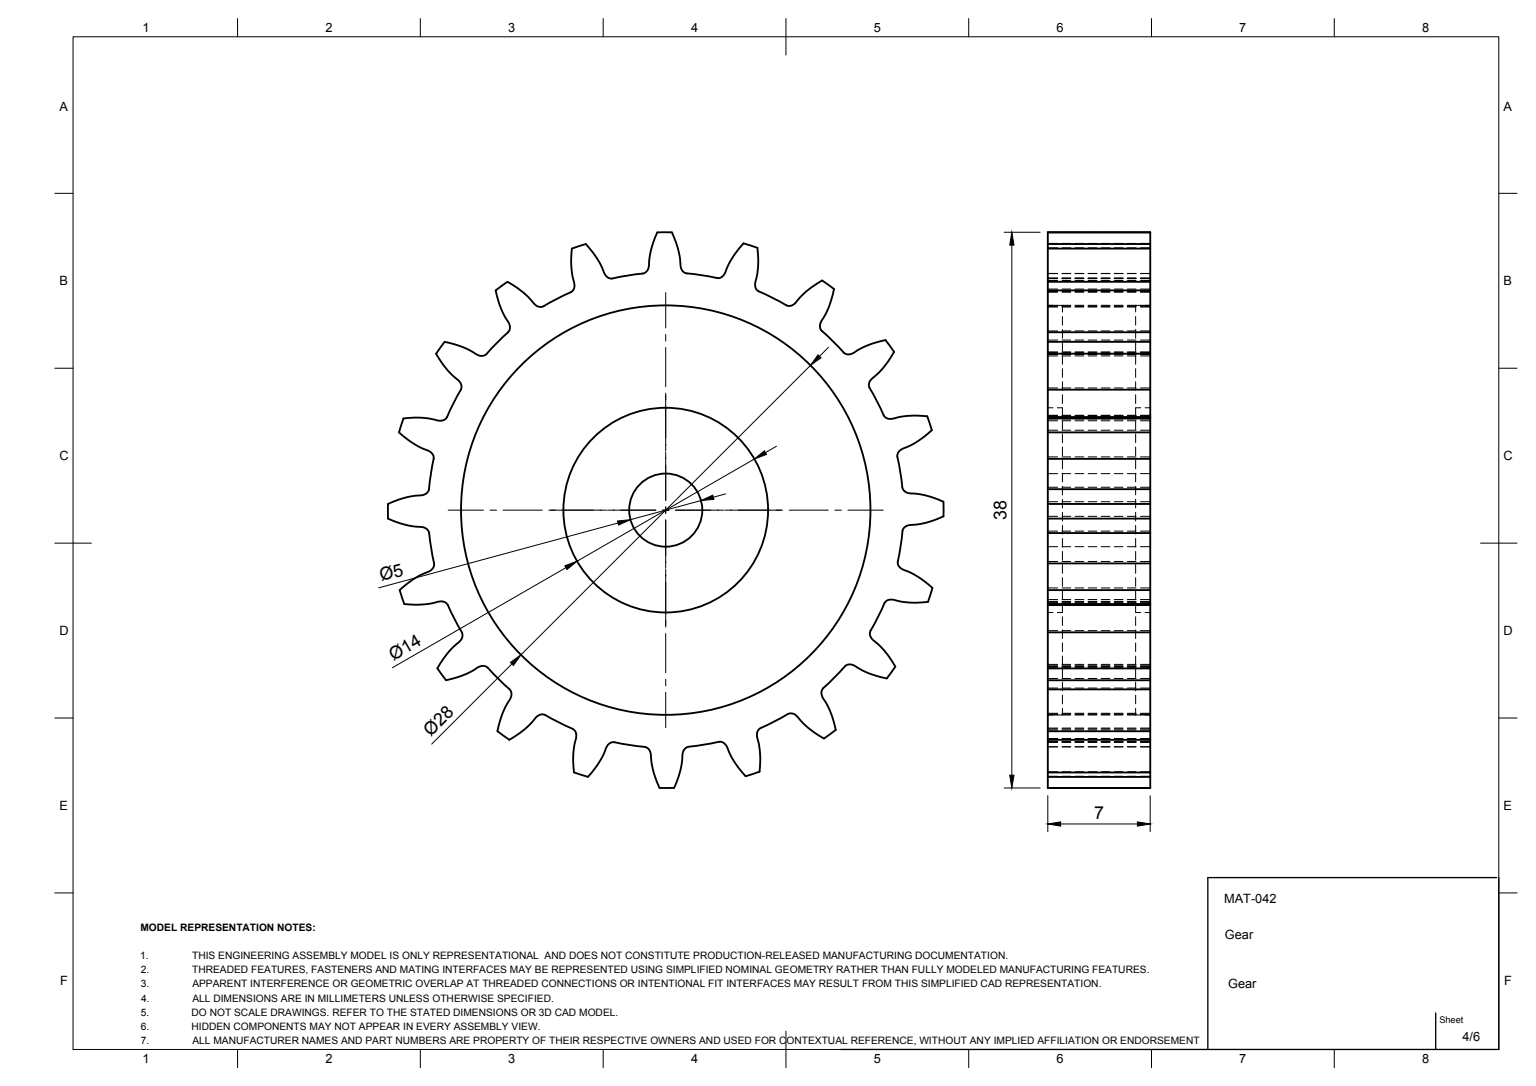
ISO-10303-21;
HEADER;
/* Generated by software containing ST-Developer
 * from STEP Tools, Inc. (www.steptools.com) 
 */

FILE_DESCRIPTION(
/* description */ ('STEP AP214'),
/* implementation_level */ '2;1');

FILE_NAME(
/* name */ 'Gear.step',
/* time_stamp */ '2026-11-14T22:03:06-08:00',
/* author */ (''),
/* organization */ (''),
/* preprocessor_version */ 'ST-DEVELOPER v20.2',
/* originating_system */ 'Autodesk Translation Framework v15.17.0.0',
/* authorisation */ '');

FILE_SCHEMA (('AUTOMOTIVE_DESIGN { 1 0 10303 214 3 1 1 }'));
ENDSEC;

DATA;
#10=MECHANICAL_DESIGN_GEOMETRIC_PRESENTATION_REPRESENTATION('',(#309),#12966);
#167=B_SPLINE_SURFACE_WITH_KNOTS('',3,1,((#10554,#10555),(#10556,#10557),
(#10558,#10559),(#10560,#10561),(#10562,#10563),(#10564,#10565),(#10566,
#10567),(#10568,#10569),(#10570,#10571),(#10572,#10573),(#10574,#10575),
(#10576,#10577),(#10578,#10579),(#10580,#10581),(#10582,#10583),(#10584,
#10585),(#10586,#10587),(#10588,#10589),(#10590,#10591),(#10592,#10593),
(#10594,#10595),(#10596,#10597),(#10598,#10599)),.UNSPECIFIED.,.F.,.F.,
 .F.,(4,1,1,1,1,1,1,1,1,1,1,1,1,1,1,1,1,1,1,1,4),(2,2),(0.0323453817713401,
0.0983189520624214,0.14064060480402,0.176193019733645,0.208307484243854,
0.23948443235858,0.271287112904486,0.28220667781497,0.293329328714142,0.304676551002397,
0.319437818234531,0.350137192454192,0.38765864687273,0.432002181900136,
0.483167797782405,0.541155494678712,0.605965272697963,0.67759713191795,
0.75605107239617,0.841327094176323,1.),(0.,0.84),.UNSPECIFIED.);
#168=B_SPLINE_SURFACE_WITH_KNOTS('',3,1,((#10604,#10605),(#10606,#10607),
(#10608,#10609),(#10610,#10611),(#10612,#10613),(#10614,#10615),(#10616,
#10617),(#10618,#10619),(#10620,#10621),(#10622,#10623),(#10624,#10625),
(#10626,#10627),(#10628,#10629),(#10630,#10631),(#10632,#10633),(#10634,
#10635),(#10636,#10637),(#10638,#10639),(#10640,#10641),(#10642,#10643),
(#10644,#10645),(#10646,#10647),(#10648,#10649)),.UNSPECIFIED.,.F.,.F.,
 .F.,(4,1,1,1,1,1,1,1,1,1,1,1,1,1,1,1,1,1,1,1,4),(2,2),(0.,0.158672905823676,
0.243948927603829,0.322402868082049,0.394034727302036,0.458844505321287,
0.516832202217594,0.567997818099863,0.612341353127269,0.649862807545807,
0.680562181765468,0.695323448997602,0.706670671285856,0.717793322185029,
0.728712887095513,0.760515567641419,0.791692515756145,0.823806980266354,
0.859359395195979,0.901681047937578,0.967654618228659),(0.,0.839999999999999),
 .UNSPECIFIED.);
#169=B_SPLINE_SURFACE_WITH_KNOTS('',3,1,((#10653,#10654),(#10655,#10656),
(#10657,#10658),(#10659,#10660),(#10661,#10662),(#10663,#10664),(#10665,
#10666),(#10667,#10668),(#10669,#10670),(#10671,#10672),(#10673,#10674),
(#10675,#10676),(#10677,#10678),(#10679,#10680),(#10681,#10682),(#10683,
#10684),(#10685,#10686),(#10687,#10688),(#10689,#10690),(#10691,#10692),
(#10693,#10694),(#10695,#10696),(#10697,#10698)),.UNSPECIFIED.,.F.,.F.,
 .F.,(4,1,1,1,1,1,1,1,1,1,1,1,1,1,1,1,1,1,1,1,4),(2,2),(0.0323453817713401,
0.0983189520624214,0.14064060480402,0.176193019733645,0.208307484243854,
0.23948443235858,0.271287112904486,0.28220667781497,0.293329328714142,0.304676551002397,
0.319437818234531,0.350137192454192,0.38765864687273,0.432002181900136,
0.483167797782405,0.541155494678712,0.605965272697963,0.67759713191795,
0.75605107239617,0.841327094176323,1.),(0.,0.84),.UNSPECIFIED.);
#170=B_SPLINE_SURFACE_WITH_KNOTS('',3,1,((#10702,#10703),(#10704,#10705),
(#10706,#10707),(#10708,#10709),(#10710,#10711),(#10712,#10713),(#10714,
#10715),(#10716,#10717),(#10718,#10719),(#10720,#10721),(#10722,#10723),
(#10724,#10725),(#10726,#10727),(#10728,#10729),(#10730,#10731),(#10732,
#10733),(#10734,#10735),(#10736,#10737),(#10738,#10739),(#10740,#10741),
(#10742,#10743),(#10744,#10745),(#10746,#10747)),.UNSPECIFIED.,.F.,.F.,
 .F.,(4,1,1,1,1,1,1,1,1,1,1,1,1,1,1,1,1,1,1,1,4),(2,2),(0.,0.158672905823676,
0.243948927603829,0.322402868082049,0.394034727302036,0.458844505321287,
0.516832202217594,0.567997818099863,0.612341353127269,0.649862807545807,
0.680562181765468,0.695323448997602,0.706670671285856,0.717793322185029,
0.728712887095513,0.760515567641419,0.791692515756145,0.823806980266354,
0.859359395195979,0.901681047937578,0.967654618228659),(0.,0.839999999999998),
 .UNSPECIFIED.);
#171=B_SPLINE_SURFACE_WITH_KNOTS('',3,1,((#10751,#10752),(#10753,#10754),
(#10755,#10756),(#10757,#10758),(#10759,#10760),(#10761,#10762),(#10763,
#10764),(#10765,#10766),(#10767,#10768),(#10769,#10770),(#10771,#10772),
(#10773,#10774),(#10775,#10776),(#10777,#10778),(#10779,#10780),(#10781,
#10782),(#10783,#10784),(#10785,#10786),(#10787,#10788),(#10789,#10790),
(#10791,#10792),(#10793,#10794),(#10795,#10796)),.UNSPECIFIED.,.F.,.F.,
 .F.,(4,1,1,1,1,1,1,1,1,1,1,1,1,1,1,1,1,1,1,1,4),(2,2),(0.0323453817713401,
0.0983189520624214,0.14064060480402,0.176193019733645,0.208307484243854,
0.23948443235858,0.271287112904486,0.28220667781497,0.293329328714142,0.304676551002397,
0.319437818234531,0.350137192454192,0.38765864687273,0.432002181900136,
0.483167797782405,0.541155494678712,0.605965272697963,0.67759713191795,
0.75605107239617,0.841327094176323,1.),(0.,0.84),.UNSPECIFIED.);
#172=B_SPLINE_SURFACE_WITH_KNOTS('',3,1,((#10800,#10801),(#10802,#10803),
(#10804,#10805),(#10806,#10807),(#10808,#10809),(#10810,#10811),(#10812,
#10813),(#10814,#10815),(#10816,#10817),(#10818,#10819),(#10820,#10821),
(#10822,#10823),(#10824,#10825),(#10826,#10827),(#10828,#10829),(#10830,
#10831),(#10832,#10833),(#10834,#10835),(#10836,#10837),(#10838,#10839),
(#10840,#10841),(#10842,#10843),(#10844,#10845)),.UNSPECIFIED.,.F.,.F.,
 .F.,(4,1,1,1,1,1,1,1,1,1,1,1,1,1,1,1,1,1,1,1,4),(2,2),(0.,0.158672905823676,
0.243948927603829,0.322402868082049,0.394034727302036,0.458844505321287,
0.516832202217594,0.567997818099863,0.612341353127269,0.649862807545807,
0.680562181765468,0.695323448997602,0.706670671285856,0.717793322185029,
0.728712887095513,0.760515567641419,0.791692515756145,0.823806980266354,
0.859359395195979,0.901681047937578,0.967654618228659),(0.,0.839999999999999),
 .UNSPECIFIED.);
#173=B_SPLINE_SURFACE_WITH_KNOTS('',3,1,((#10849,#10850),(#10851,#10852),
(#10853,#10854),(#10855,#10856),(#10857,#10858),(#10859,#10860),(#10861,
#10862),(#10863,#10864),(#10865,#10866),(#10867,#10868),(#10869,#10870),
(#10871,#10872),(#10873,#10874),(#10875,#10876),(#10877,#10878),(#10879,
#10880),(#10881,#10882),(#10883,#10884),(#10885,#10886),(#10887,#10888),
(#10889,#10890),(#10891,#10892),(#10893,#10894)),.UNSPECIFIED.,.F.,.F.,
 .F.,(4,1,1,1,1,1,1,1,1,1,1,1,1,1,1,1,1,1,1,1,4),(2,2),(0.0323453817713401,
0.0983189520624214,0.14064060480402,0.176193019733645,0.208307484243854,
0.23948443235858,0.271287112904486,0.28220667781497,0.293329328714142,0.304676551002397,
0.319437818234531,0.350137192454192,0.38765864687273,0.432002181900136,
0.483167797782405,0.541155494678712,0.605965272697963,0.67759713191795,
0.75605107239617,0.841327094176323,1.),(0.,0.840000000000002),
 .UNSPECIFIED.);
#174=B_SPLINE_SURFACE_WITH_KNOTS('',3,1,((#10898,#10899),(#10900,#10901),
(#10902,#10903),(#10904,#10905),(#10906,#10907),(#10908,#10909),(#10910,
#10911),(#10912,#10913),(#10914,#10915),(#10916,#10917),(#10918,#10919),
(#10920,#10921),(#10922,#10923),(#10924,#10925),(#10926,#10927),(#10928,
#10929),(#10930,#10931),(#10932,#10933),(#10934,#10935),(#10936,#10937),
(#10938,#10939),(#10940,#10941),(#10942,#10943)),.UNSPECIFIED.,.F.,.F.,
 .F.,(4,1,1,1,1,1,1,1,1,1,1,1,1,1,1,1,1,1,1,1,4),(2,2),(0.,0.158672905823676,
0.243948927603829,0.322402868082049,0.394034727302036,0.458844505321287,
0.516832202217594,0.567997818099863,0.612341353127269,0.649862807545807,
0.680562181765468,0.695323448997602,0.706670671285856,0.717793322185029,
0.728712887095513,0.760515567641419,0.791692515756145,0.823806980266354,
0.859359395195979,0.901681047937578,0.967654618228659),(0.,0.84),
 .UNSPECIFIED.);
#175=B_SPLINE_SURFACE_WITH_KNOTS('',3,1,((#10947,#10948),(#10949,#10950),
(#10951,#10952),(#10953,#10954),(#10955,#10956),(#10957,#10958),(#10959,
#10960),(#10961,#10962),(#10963,#10964),(#10965,#10966),(#10967,#10968),
(#10969,#10970),(#10971,#10972),(#10973,#10974),(#10975,#10976),(#10977,
#10978),(#10979,#10980),(#10981,#10982),(#10983,#10984),(#10985,#10986),
(#10987,#10988),(#10989,#10990),(#10991,#10992)),.UNSPECIFIED.,.F.,.F.,
 .F.,(4,1,1,1,1,1,1,1,1,1,1,1,1,1,1,1,1,1,1,1,4),(2,2),(0.0323453817713401,
0.0983189520624214,0.14064060480402,0.176193019733645,0.208307484243854,
0.23948443235858,0.271287112904486,0.28220667781497,0.293329328714142,0.304676551002397,
0.319437818234531,0.350137192454192,0.38765864687273,0.432002181900136,
0.483167797782405,0.541155494678712,0.605965272697963,0.67759713191795,
0.75605107239617,0.841327094176323,1.),(0.,0.84),.UNSPECIFIED.);
#176=B_SPLINE_SURFACE_WITH_KNOTS('',3,1,((#10996,#10997),(#10998,#10999),
(#11000,#11001),(#11002,#11003),(#11004,#11005),(#11006,#11007),(#11008,
#11009),(#11010,#11011),(#11012,#11013),(#11014,#11015),(#11016,#11017),
(#11018,#11019),(#11020,#11021),(#11022,#11023),(#11024,#11025),(#11026,
#11027),(#11028,#11029),(#11030,#11031),(#11032,#11033),(#11034,#11035),
(#11036,#11037),(#11038,#11039),(#11040,#11041)),.UNSPECIFIED.,.F.,.F.,
 .F.,(4,1,1,1,1,1,1,1,1,1,1,1,1,1,1,1,1,1,1,1,4),(2,2),(0.,0.158672905823676,
0.243948927603829,0.322402868082049,0.394034727302036,0.458844505321287,
0.516832202217594,0.567997818099863,0.612341353127269,0.649862807545807,
0.680562181765468,0.695323448997602,0.706670671285856,0.717793322185029,
0.728712887095513,0.760515567641419,0.791692515756145,0.823806980266354,
0.859359395195979,0.901681047937578,0.967654618228659),(0.,0.839999999999999),
 .UNSPECIFIED.);
#177=B_SPLINE_SURFACE_WITH_KNOTS('',3,1,((#11045,#11046),(#11047,#11048),
(#11049,#11050),(#11051,#11052),(#11053,#11054),(#11055,#11056),(#11057,
#11058),(#11059,#11060),(#11061,#11062),(#11063,#11064),(#11065,#11066),
(#11067,#11068),(#11069,#11070),(#11071,#11072),(#11073,#11074),(#11075,
#11076),(#11077,#11078),(#11079,#11080),(#11081,#11082),(#11083,#11084),
(#11085,#11086),(#11087,#11088),(#11089,#11090)),.UNSPECIFIED.,.F.,.F.,
 .F.,(4,1,1,1,1,1,1,1,1,1,1,1,1,1,1,1,1,1,1,1,4),(2,2),(0.0323453817713401,
0.0983189520624214,0.14064060480402,0.176193019733645,0.208307484243854,
0.23948443235858,0.271287112904486,0.28220667781497,0.293329328714142,0.304676551002397,
0.319437818234531,0.350137192454192,0.38765864687273,0.432002181900136,
0.483167797782405,0.541155494678712,0.605965272697963,0.67759713191795,
0.75605107239617,0.841327094176323,1.),(0.,0.84),.UNSPECIFIED.);
#178=B_SPLINE_SURFACE_WITH_KNOTS('',3,1,((#11094,#11095),(#11096,#11097),
(#11098,#11099),(#11100,#11101),(#11102,#11103),(#11104,#11105),(#11106,
#11107),(#11108,#11109),(#11110,#11111),(#11112,#11113),(#11114,#11115),
(#11116,#11117),(#11118,#11119),(#11120,#11121),(#11122,#11123),(#11124,
#11125),(#11126,#11127),(#11128,#11129),(#11130,#11131),(#11132,#11133),
(#11134,#11135),(#11136,#11137),(#11138,#11139)),.UNSPECIFIED.,.F.,.F.,
 .F.,(4,1,1,1,1,1,1,1,1,1,1,1,1,1,1,1,1,1,1,1,4),(2,2),(0.,0.158672905823676,
0.243948927603829,0.322402868082049,0.394034727302036,0.458844505321287,
0.516832202217594,0.567997818099863,0.612341353127269,0.649862807545807,
0.680562181765468,0.695323448997602,0.706670671285856,0.717793322185029,
0.728712887095513,0.760515567641419,0.791692515756145,0.823806980266354,
0.859359395195979,0.901681047937578,0.967654618228659),(0.,0.84),
 .UNSPECIFIED.);
#179=B_SPLINE_SURFACE_WITH_KNOTS('',3,1,((#11143,#11144),(#11145,#11146),
(#11147,#11148),(#11149,#11150),(#11151,#11152),(#11153,#11154),(#11155,
#11156),(#11157,#11158),(#11159,#11160),(#11161,#11162),(#11163,#11164),
(#11165,#11166),(#11167,#11168),(#11169,#11170),(#11171,#11172),(#11173,
#11174),(#11175,#11176),(#11177,#11178),(#11179,#11180),(#11181,#11182),
(#11183,#11184),(#11185,#11186),(#11187,#11188)),.UNSPECIFIED.,.F.,.F.,
 .F.,(4,1,1,1,1,1,1,1,1,1,1,1,1,1,1,1,1,1,1,1,4),(2,2),(0.0323453817713401,
0.0983189520624214,0.14064060480402,0.176193019733645,0.208307484243854,
0.23948443235858,0.271287112904486,0.28220667781497,0.293329328714142,0.304676551002397,
0.319437818234531,0.350137192454192,0.38765864687273,0.432002181900136,
0.483167797782405,0.541155494678712,0.605965272697963,0.67759713191795,
0.75605107239617,0.841327094176323,1.),(0.,0.84),.UNSPECIFIED.);
#180=B_SPLINE_SURFACE_WITH_KNOTS('',3,1,((#11192,#11193),(#11194,#11195),
(#11196,#11197),(#11198,#11199),(#11200,#11201),(#11202,#11203),(#11204,
#11205),(#11206,#11207),(#11208,#11209),(#11210,#11211),(#11212,#11213),
(#11214,#11215),(#11216,#11217),(#11218,#11219),(#11220,#11221),(#11222,
#11223),(#11224,#11225),(#11226,#11227),(#11228,#11229),(#11230,#11231),
(#11232,#11233),(#11234,#11235),(#11236,#11237)),.UNSPECIFIED.,.F.,.F.,
 .F.,(4,1,1,1,1,1,1,1,1,1,1,1,1,1,1,1,1,1,1,1,4),(2,2),(0.,0.158672905823676,
0.243948927603829,0.322402868082049,0.394034727302036,0.458844505321287,
0.516832202217594,0.567997818099863,0.612341353127269,0.649862807545807,
0.680562181765468,0.695323448997602,0.706670671285856,0.717793322185029,
0.728712887095513,0.760515567641419,0.791692515756145,0.823806980266354,
0.859359395195979,0.901681047937578,0.967654618228659),(0.,0.84),
 .UNSPECIFIED.);
#181=B_SPLINE_SURFACE_WITH_KNOTS('',3,1,((#11241,#11242),(#11243,#11244),
(#11245,#11246),(#11247,#11248),(#11249,#11250),(#11251,#11252),(#11253,
#11254),(#11255,#11256),(#11257,#11258),(#11259,#11260),(#11261,#11262),
(#11263,#11264),(#11265,#11266),(#11267,#11268),(#11269,#11270),(#11271,
#11272),(#11273,#11274),(#11275,#11276),(#11277,#11278),(#11279,#11280),
(#11281,#11282),(#11283,#11284),(#11285,#11286)),.UNSPECIFIED.,.F.,.F.,
 .F.,(4,1,1,1,1,1,1,1,1,1,1,1,1,1,1,1,1,1,1,1,4),(2,2),(0.0323453817713401,
0.0983189520624214,0.14064060480402,0.176193019733645,0.208307484243854,
0.23948443235858,0.271287112904486,0.28220667781497,0.293329328714142,0.304676551002397,
0.319437818234531,0.350137192454192,0.38765864687273,0.432002181900136,
0.483167797782405,0.541155494678712,0.605965272697963,0.67759713191795,
0.75605107239617,0.841327094176323,1.),(0.,0.84),.UNSPECIFIED.);
#182=B_SPLINE_SURFACE_WITH_KNOTS('',3,1,((#11290,#11291),(#11292,#11293),
(#11294,#11295),(#11296,#11297),(#11298,#11299),(#11300,#11301),(#11302,
#11303),(#11304,#11305),(#11306,#11307),(#11308,#11309),(#11310,#11311),
(#11312,#11313),(#11314,#11315),(#11316,#11317),(#11318,#11319),(#11320,
#11321),(#11322,#11323),(#11324,#11325),(#11326,#11327),(#11328,#11329),
(#11330,#11331),(#11332,#11333),(#11334,#11335)),.UNSPECIFIED.,.F.,.F.,
 .F.,(4,1,1,1,1,1,1,1,1,1,1,1,1,1,1,1,1,1,1,1,4),(2,2),(0.,0.158672905823676,
0.243948927603829,0.322402868082049,0.394034727302036,0.458844505321287,
0.516832202217594,0.567997818099863,0.612341353127269,0.649862807545807,
0.680562181765468,0.695323448997602,0.706670671285856,0.717793322185029,
0.728712887095513,0.760515567641419,0.791692515756145,0.823806980266354,
0.859359395195979,0.901681047937578,0.967654618228659),(0.,0.839999999999999),
 .UNSPECIFIED.);
#183=B_SPLINE_SURFACE_WITH_KNOTS('',3,1,((#11339,#11340),(#11341,#11342),
(#11343,#11344),(#11345,#11346),(#11347,#11348),(#11349,#11350),(#11351,
#11352),(#11353,#11354),(#11355,#11356),(#11357,#11358),(#11359,#11360),
(#11361,#11362),(#11363,#11364),(#11365,#11366),(#11367,#11368),(#11369,
#11370),(#11371,#11372),(#11373,#11374),(#11375,#11376),(#11377,#11378),
(#11379,#11380),(#11381,#11382),(#11383,#11384)),.UNSPECIFIED.,.F.,.F.,
 .F.,(4,1,1,1,1,1,1,1,1,1,1,1,1,1,1,1,1,1,1,1,4),(2,2),(0.0323453817713401,
0.0983189520624214,0.14064060480402,0.176193019733645,0.208307484243854,
0.23948443235858,0.271287112904486,0.28220667781497,0.293329328714142,0.304676551002397,
0.319437818234531,0.350137192454192,0.38765864687273,0.432002181900136,
0.483167797782405,0.541155494678712,0.605965272697963,0.67759713191795,
0.75605107239617,0.841327094176323,1.),(0.,0.84),.UNSPECIFIED.);
#184=B_SPLINE_SURFACE_WITH_KNOTS('',3,1,((#11388,#11389),(#11390,#11391),
(#11392,#11393),(#11394,#11395),(#11396,#11397),(#11398,#11399),(#11400,
#11401),(#11402,#11403),(#11404,#11405),(#11406,#11407),(#11408,#11409),
(#11410,#11411),(#11412,#11413),(#11414,#11415),(#11416,#11417),(#11418,
#11419),(#11420,#11421),(#11422,#11423),(#11424,#11425),(#11426,#11427),
(#11428,#11429),(#11430,#11431),(#11432,#11433)),.UNSPECIFIED.,.F.,.F.,
 .F.,(4,1,1,1,1,1,1,1,1,1,1,1,1,1,1,1,1,1,1,1,4),(2,2),(0.,0.158672905823676,
0.243948927603829,0.322402868082049,0.394034727302036,0.458844505321287,
0.516832202217594,0.567997818099863,0.612341353127269,0.649862807545807,
0.680562181765468,0.695323448997602,0.706670671285856,0.717793322185029,
0.728712887095513,0.760515567641419,0.791692515756145,0.823806980266354,
0.859359395195979,0.901681047937578,0.967654618228659),(0.,0.839999999999999),
 .UNSPECIFIED.);
#185=B_SPLINE_SURFACE_WITH_KNOTS('',3,1,((#11434,#11435),(#11436,#11437),
(#11438,#11439),(#11440,#11441),(#11442,#11443),(#11444,#11445),(#11446,
#11447),(#11448,#11449),(#11450,#11451),(#11452,#11453),(#11454,#11455),
(#11456,#11457),(#11458,#11459),(#11460,#11461),(#11462,#11463),(#11464,
#11465),(#11466,#11467),(#11468,#11469),(#11470,#11471),(#11472,#11473),
(#11474,#11475),(#11476,#11477),(#11478,#11479)),.UNSPECIFIED.,.F.,.F.,
 .F.,(4,1,1,1,1,1,1,1,1,1,1,1,1,1,1,1,1,1,1,1,4),(2,2),(0.0323453817713401,
0.0983189520624214,0.14064060480402,0.176193019733645,0.208307484243854,
0.23948443235858,0.271287112904486,0.28220667781497,0.293329328714142,0.304676551002397,
0.319437818234531,0.350137192454192,0.38765864687273,0.432002181900136,
0.483167797782405,0.541155494678712,0.605965272697963,0.67759713191795,
0.75605107239617,0.841327094176323,1.),(0.,0.84),.UNSPECIFIED.);
#186=B_SPLINE_SURFACE_WITH_KNOTS('',3,1,((#11483,#11484),(#11485,#11486),
(#11487,#11488),(#11489,#11490),(#11491,#11492),(#11493,#11494),(#11495,
#11496),(#11497,#11498),(#11499,#11500),(#11501,#11502),(#11503,#11504),
(#11505,#11506),(#11507,#11508),(#11509,#11510),(#11511,#11512),(#11513,
#11514),(#11515,#11516),(#11517,#11518),(#11519,#11520),(#11521,#11522),
(#11523,#11524),(#11525,#11526),(#11527,#11528)),.UNSPECIFIED.,.F.,.F.,
 .F.,(4,1,1,1,1,1,1,1,1,1,1,1,1,1,1,1,1,1,1,1,4),(2,2),(0.,0.158672905823676,
0.243948927603829,0.322402868082049,0.394034727302036,0.458844505321287,
0.516832202217594,0.567997818099863,0.612341353127269,0.649862807545807,
0.680562181765468,0.695323448997602,0.706670671285856,0.717793322185029,
0.728712887095513,0.760515567641419,0.791692515756145,0.823806980266354,
0.859359395195979,0.901681047937578,0.967654618228659),(0.,0.839999999999999),
 .UNSPECIFIED.);
#187=B_SPLINE_SURFACE_WITH_KNOTS('',3,1,((#11532,#11533),(#11534,#11535),
(#11536,#11537),(#11538,#11539),(#11540,#11541),(#11542,#11543),(#11544,
#11545),(#11546,#11547),(#11548,#11549),(#11550,#11551),(#11552,#11553),
(#11554,#11555),(#11556,#11557),(#11558,#11559),(#11560,#11561),(#11562,
#11563),(#11564,#11565),(#11566,#11567),(#11568,#11569),(#11570,#11571),
(#11572,#11573),(#11574,#11575),(#11576,#11577)),.UNSPECIFIED.,.F.,.F.,
 .F.,(4,1,1,1,1,1,1,1,1,1,1,1,1,1,1,1,1,1,1,1,4),(2,2),(0.0323453817713401,
0.0983189520624214,0.14064060480402,0.176193019733645,0.208307484243854,
0.23948443235858,0.271287112904486,0.28220667781497,0.293329328714142,0.304676551002397,
0.319437818234531,0.350137192454192,0.38765864687273,0.432002181900136,
0.483167797782405,0.541155494678712,0.605965272697963,0.67759713191795,
0.75605107239617,0.841327094176323,1.),(0.,0.840000000000002),
 .UNSPECIFIED.);
#188=B_SPLINE_SURFACE_WITH_KNOTS('',3,1,((#11581,#11582),(#11583,#11584),
(#11585,#11586),(#11587,#11588),(#11589,#11590),(#11591,#11592),(#11593,
#11594),(#11595,#11596),(#11597,#11598),(#11599,#11600),(#11601,#11602),
(#11603,#11604),(#11605,#11606),(#11607,#11608),(#11609,#11610),(#11611,
#11612),(#11613,#11614),(#11615,#11616),(#11617,#11618),(#11619,#11620),
(#11621,#11622),(#11623,#11624),(#11625,#11626)),.UNSPECIFIED.,.F.,.F.,
 .F.,(4,1,1,1,1,1,1,1,1,1,1,1,1,1,1,1,1,1,1,1,4),(2,2),(0.,0.158672905823676,
0.243948927603829,0.322402868082049,0.394034727302036,0.458844505321287,
0.516832202217594,0.567997818099863,0.612341353127269,0.649862807545807,
0.680562181765468,0.695323448997602,0.706670671285856,0.717793322185029,
0.728712887095513,0.760515567641419,0.791692515756145,0.823806980266354,
0.859359395195979,0.901681047937578,0.967654618228659),(0.,0.84),
 .UNSPECIFIED.);
#189=B_SPLINE_SURFACE_WITH_KNOTS('',3,1,((#11630,#11631),(#11632,#11633),
(#11634,#11635),(#11636,#11637),(#11638,#11639),(#11640,#11641),(#11642,
#11643),(#11644,#11645),(#11646,#11647),(#11648,#11649),(#11650,#11651),
(#11652,#11653),(#11654,#11655),(#11656,#11657),(#11658,#11659),(#11660,
#11661),(#11662,#11663),(#11664,#11665),(#11666,#11667),(#11668,#11669),
(#11670,#11671),(#11672,#11673),(#11674,#11675)),.UNSPECIFIED.,.F.,.F.,
 .F.,(4,1,1,1,1,1,1,1,1,1,1,1,1,1,1,1,1,1,1,1,4),(2,2),(0.0323453817713401,
0.0983189520624214,0.14064060480402,0.176193019733645,0.208307484243854,
0.23948443235858,0.271287112904486,0.28220667781497,0.293329328714142,0.304676551002397,
0.319437818234531,0.350137192454192,0.38765864687273,0.432002181900136,
0.483167797782405,0.541155494678712,0.605965272697963,0.67759713191795,
0.75605107239617,0.841327094176323,1.),(0.,0.84),.UNSPECIFIED.);
#190=B_SPLINE_SURFACE_WITH_KNOTS('',3,1,((#11679,#11680),(#11681,#11682),
(#11683,#11684),(#11685,#11686),(#11687,#11688),(#11689,#11690),(#11691,
#11692),(#11693,#11694),(#11695,#11696),(#11697,#11698),(#11699,#11700),
(#11701,#11702),(#11703,#11704),(#11705,#11706),(#11707,#11708),(#11709,
#11710),(#11711,#11712),(#11713,#11714),(#11715,#11716),(#11717,#11718),
(#11719,#11720),(#11721,#11722),(#11723,#11724)),.UNSPECIFIED.,.F.,.F.,
 .F.,(4,1,1,1,1,1,1,1,1,1,1,1,1,1,1,1,1,1,1,1,4),(2,2),(0.,0.158672905823676,
0.243948927603829,0.322402868082049,0.394034727302036,0.458844505321287,
0.516832202217594,0.567997818099863,0.612341353127269,0.649862807545807,
0.680562181765468,0.695323448997602,0.706670671285856,0.717793322185029,
0.728712887095513,0.760515567641419,0.791692515756145,0.823806980266354,
0.859359395195979,0.901681047937578,0.967654618228659),(0.,0.839999999999999),
 .UNSPECIFIED.);
#191=B_SPLINE_SURFACE_WITH_KNOTS('',3,1,((#11728,#11729),(#11730,#11731),
(#11732,#11733),(#11734,#11735),(#11736,#11737),(#11738,#11739),(#11740,
#11741),(#11742,#11743),(#11744,#11745),(#11746,#11747),(#11748,#11749),
(#11750,#11751),(#11752,#11753),(#11754,#11755),(#11756,#11757),(#11758,
#11759),(#11760,#11761),(#11762,#11763),(#11764,#11765),(#11766,#11767),
(#11768,#11769),(#11770,#11771),(#11772,#11773)),.UNSPECIFIED.,.F.,.F.,
 .F.,(4,1,1,1,1,1,1,1,1,1,1,1,1,1,1,1,1,1,1,1,4),(2,2),(0.0323453817713401,
0.0983189520624214,0.14064060480402,0.176193019733645,0.208307484243854,
0.23948443235858,0.271287112904486,0.28220667781497,0.293329328714142,0.304676551002397,
0.319437818234531,0.350137192454192,0.38765864687273,0.432002181900136,
0.483167797782405,0.541155494678712,0.605965272697963,0.67759713191795,
0.75605107239617,0.841327094176323,1.),(0.,0.839999999999998),
 .UNSPECIFIED.);
#192=B_SPLINE_SURFACE_WITH_KNOTS('',3,1,((#11777,#11778),(#11779,#11780),
(#11781,#11782),(#11783,#11784),(#11785,#11786),(#11787,#11788),(#11789,
#11790),(#11791,#11792),(#11793,#11794),(#11795,#11796),(#11797,#11798),
(#11799,#11800),(#11801,#11802),(#11803,#11804),(#11805,#11806),(#11807,
#11808),(#11809,#11810),(#11811,#11812),(#11813,#11814),(#11815,#11816),
(#11817,#11818),(#11819,#11820),(#11821,#11822)),.UNSPECIFIED.,.F.,.F.,
 .F.,(4,1,1,1,1,1,1,1,1,1,1,1,1,1,1,1,1,1,1,1,4),(2,2),(0.,0.158672905823676,
0.243948927603829,0.322402868082049,0.394034727302036,0.458844505321287,
0.516832202217594,0.567997818099863,0.612341353127269,0.649862807545807,
0.680562181765468,0.695323448997602,0.706670671285856,0.717793322185029,
0.728712887095513,0.760515567641419,0.791692515756145,0.823806980266354,
0.859359395195979,0.901681047937578,0.967654618228659),(0.,0.839999999999998),
 .UNSPECIFIED.);
#193=B_SPLINE_SURFACE_WITH_KNOTS('',3,1,((#11826,#11827),(#11828,#11829),
(#11830,#11831),(#11832,#11833),(#11834,#11835),(#11836,#11837),(#11838,
#11839),(#11840,#11841),(#11842,#11843),(#11844,#11845),(#11846,#11847),
(#11848,#11849),(#11850,#11851),(#11852,#11853),(#11854,#11855),(#11856,
#11857),(#11858,#11859),(#11860,#11861),(#11862,#11863),(#11864,#11865),
(#11866,#11867),(#11868,#11869),(#11870,#11871)),.UNSPECIFIED.,.F.,.F.,
 .F.,(4,1,1,1,1,1,1,1,1,1,1,1,1,1,1,1,1,1,1,1,4),(2,2),(0.0323453817713401,
0.0983189520624214,0.14064060480402,0.176193019733645,0.208307484243854,
0.23948443235858,0.271287112904486,0.28220667781497,0.293329328714142,0.304676551002397,
0.319437818234531,0.350137192454192,0.38765864687273,0.432002181900136,
0.483167797782405,0.541155494678712,0.605965272697963,0.67759713191795,
0.75605107239617,0.841327094176323,1.),(0.,0.839999999999998),
 .UNSPECIFIED.);
#194=B_SPLINE_SURFACE_WITH_KNOTS('',3,1,((#11875,#11876),(#11877,#11878),
(#11879,#11880),(#11881,#11882),(#11883,#11884),(#11885,#11886),(#11887,
#11888),(#11889,#11890),(#11891,#11892),(#11893,#11894),(#11895,#11896),
(#11897,#11898),(#11899,#11900),(#11901,#11902),(#11903,#11904),(#11905,
#11906),(#11907,#11908),(#11909,#11910),(#11911,#11912),(#11913,#11914),
(#11915,#11916),(#11917,#11918),(#11919,#11920)),.UNSPECIFIED.,.F.,.F.,
 .F.,(4,1,1,1,1,1,1,1,1,1,1,1,1,1,1,1,1,1,1,1,4),(2,2),(0.,0.158672905823676,
0.243948927603829,0.322402868082049,0.394034727302036,0.458844505321287,
0.516832202217594,0.567997818099863,0.612341353127269,0.649862807545807,
0.680562181765468,0.695323448997602,0.706670671285856,0.717793322185029,
0.728712887095513,0.760515567641419,0.791692515756145,0.823806980266354,
0.859359395195979,0.901681047937578,0.967654618228659),(0.,0.839999999999999),
 .UNSPECIFIED.);
#195=B_SPLINE_SURFACE_WITH_KNOTS('',3,1,((#11924,#11925),(#11926,#11927),
(#11928,#11929),(#11930,#11931),(#11932,#11933),(#11934,#11935),(#11936,
#11937),(#11938,#11939),(#11940,#11941),(#11942,#11943),(#11944,#11945),
(#11946,#11947),(#11948,#11949),(#11950,#11951),(#11952,#11953),(#11954,
#11955),(#11956,#11957),(#11958,#11959),(#11960,#11961),(#11962,#11963),
(#11964,#11965),(#11966,#11967),(#11968,#11969)),.UNSPECIFIED.,.F.,.F.,
 .F.,(4,1,1,1,1,1,1,1,1,1,1,1,1,1,1,1,1,1,1,1,4),(2,2),(0.0323453817713401,
0.0983189520624214,0.14064060480402,0.176193019733645,0.208307484243854,
0.23948443235858,0.271287112904486,0.28220667781497,0.293329328714142,0.304676551002397,
0.319437818234531,0.350137192454192,0.38765864687273,0.432002181900136,
0.483167797782405,0.541155494678712,0.605965272697963,0.67759713191795,
0.75605107239617,0.841327094176323,1.),(0.,0.84),.UNSPECIFIED.);
#196=B_SPLINE_SURFACE_WITH_KNOTS('',3,1,((#11973,#11974),(#11975,#11976),
(#11977,#11978),(#11979,#11980),(#11981,#11982),(#11983,#11984),(#11985,
#11986),(#11987,#11988),(#11989,#11990),(#11991,#11992),(#11993,#11994),
(#11995,#11996),(#11997,#11998),(#11999,#12000),(#12001,#12002),(#12003,
#12004),(#12005,#12006),(#12007,#12008),(#12009,#12010),(#12011,#12012),
(#12013,#12014),(#12015,#12016),(#12017,#12018)),.UNSPECIFIED.,.F.,.F.,
 .F.,(4,1,1,1,1,1,1,1,1,1,1,1,1,1,1,1,1,1,1,1,4),(2,2),(0.,0.158672905823676,
0.243948927603829,0.322402868082049,0.394034727302036,0.458844505321287,
0.516832202217594,0.567997818099863,0.612341353127269,0.649862807545807,
0.680562181765468,0.695323448997602,0.706670671285856,0.717793322185029,
0.728712887095513,0.760515567641419,0.791692515756145,0.823806980266354,
0.859359395195979,0.901681047937578,0.967654618228659),(0.,0.84),
 .UNSPECIFIED.);
#197=B_SPLINE_SURFACE_WITH_KNOTS('',3,1,((#12022,#12023),(#12024,#12025),
(#12026,#12027),(#12028,#12029),(#12030,#12031),(#12032,#12033),(#12034,
#12035),(#12036,#12037),(#12038,#12039),(#12040,#12041),(#12042,#12043),
(#12044,#12045),(#12046,#12047),(#12048,#12049),(#12050,#12051),(#12052,
#12053),(#12054,#12055),(#12056,#12057),(#12058,#12059),(#12060,#12061),
(#12062,#12063),(#12064,#12065),(#12066,#12067)),.UNSPECIFIED.,.F.,.F.,
 .F.,(4,1,1,1,1,1,1,1,1,1,1,1,1,1,1,1,1,1,1,1,4),(2,2),(0.0323453817713401,
0.0983189520624214,0.14064060480402,0.176193019733645,0.208307484243854,
0.23948443235858,0.271287112904486,0.28220667781497,0.293329328714142,0.304676551002397,
0.319437818234531,0.350137192454192,0.38765864687273,0.432002181900136,
0.483167797782405,0.541155494678712,0.605965272697963,0.67759713191795,
0.75605107239617,0.841327094176323,1.),(0.,0.84),.UNSPECIFIED.);
#198=B_SPLINE_SURFACE_WITH_KNOTS('',3,1,((#12071,#12072),(#12073,#12074),
(#12075,#12076),(#12077,#12078),(#12079,#12080),(#12081,#12082),(#12083,
#12084),(#12085,#12086),(#12087,#12088),(#12089,#12090),(#12091,#12092),
(#12093,#12094),(#12095,#12096),(#12097,#12098),(#12099,#12100),(#12101,
#12102),(#12103,#12104),(#12105,#12106),(#12107,#12108),(#12109,#12110),
(#12111,#12112),(#12113,#12114),(#12115,#12116)),.UNSPECIFIED.,.F.,.F.,
 .F.,(4,1,1,1,1,1,1,1,1,1,1,1,1,1,1,1,1,1,1,1,4),(2,2),(0.,0.158672905823676,
0.243948927603829,0.322402868082049,0.394034727302036,0.458844505321287,
0.516832202217594,0.567997818099863,0.612341353127269,0.649862807545807,
0.680562181765468,0.695323448997602,0.706670671285856,0.717793322185029,
0.728712887095513,0.760515567641419,0.791692515756145,0.823806980266354,
0.859359395195979,0.901681047937578,0.967654618228659),(0.,0.839999999999999),
 .UNSPECIFIED.);
#199=B_SPLINE_SURFACE_WITH_KNOTS('',3,1,((#12120,#12121),(#12122,#12123),
(#12124,#12125),(#12126,#12127),(#12128,#12129),(#12130,#12131),(#12132,
#12133),(#12134,#12135),(#12136,#12137),(#12138,#12139),(#12140,#12141),
(#12142,#12143),(#12144,#12145),(#12146,#12147),(#12148,#12149),(#12150,
#12151),(#12152,#12153),(#12154,#12155),(#12156,#12157),(#12158,#12159),
(#12160,#12161),(#12162,#12163),(#12164,#12165)),.UNSPECIFIED.,.F.,.F.,
 .F.,(4,1,1,1,1,1,1,1,1,1,1,1,1,1,1,1,1,1,1,1,4),(2,2),(0.0323453817713401,
0.0983189520624214,0.14064060480402,0.176193019733645,0.208307484243854,
0.23948443235858,0.271287112904486,0.28220667781497,0.293329328714142,0.304676551002397,
0.319437818234531,0.350137192454192,0.38765864687273,0.432002181900136,
0.483167797782405,0.541155494678712,0.605965272697963,0.67759713191795,
0.75605107239617,0.841327094176323,1.),(0.,0.84),.UNSPECIFIED.);
#200=B_SPLINE_SURFACE_WITH_KNOTS('',3,1,((#12169,#12170),(#12171,#12172),
(#12173,#12174),(#12175,#12176),(#12177,#12178),(#12179,#12180),(#12181,
#12182),(#12183,#12184),(#12185,#12186),(#12187,#12188),(#12189,#12190),
(#12191,#12192),(#12193,#12194),(#12195,#12196),(#12197,#12198),(#12199,
#12200),(#12201,#12202),(#12203,#12204),(#12205,#12206),(#12207,#12208),
(#12209,#12210),(#12211,#12212),(#12213,#12214)),.UNSPECIFIED.,.F.,.F.,
 .F.,(4,1,1,1,1,1,1,1,1,1,1,1,1,1,1,1,1,1,1,1,4),(2,2),(0.,0.158672905823676,
0.243948927603829,0.322402868082049,0.394034727302036,0.458844505321287,
0.516832202217594,0.567997818099863,0.612341353127269,0.649862807545807,
0.680562181765468,0.695323448997602,0.706670671285856,0.717793322185029,
0.728712887095513,0.760515567641419,0.791692515756145,0.823806980266354,
0.859359395195979,0.901681047937578,0.967654618228659),(0.,0.84),
 .UNSPECIFIED.);
#201=B_SPLINE_SURFACE_WITH_KNOTS('',3,1,((#12218,#12219),(#12220,#12221),
(#12222,#12223),(#12224,#12225),(#12226,#12227),(#12228,#12229),(#12230,
#12231),(#12232,#12233),(#12234,#12235),(#12236,#12237),(#12238,#12239),
(#12240,#12241),(#12242,#12243),(#12244,#12245),(#12246,#12247),(#12248,
#12249),(#12250,#12251),(#12252,#12253),(#12254,#12255),(#12256,#12257),
(#12258,#12259),(#12260,#12261),(#12262,#12263)),.UNSPECIFIED.,.F.,.F.,
 .F.,(4,1,1,1,1,1,1,1,1,1,1,1,1,1,1,1,1,1,1,1,4),(2,2),(0.0323453817713401,
0.0983189520624214,0.14064060480402,0.176193019733645,0.208307484243854,
0.23948443235858,0.271287112904486,0.28220667781497,0.293329328714142,0.304676551002397,
0.319437818234531,0.350137192454192,0.38765864687273,0.432002181900136,
0.483167797782405,0.541155494678712,0.605965272697963,0.67759713191795,
0.75605107239617,0.841327094176323,1.),(0.,0.839999999999998),
 .UNSPECIFIED.);
#202=B_SPLINE_SURFACE_WITH_KNOTS('',3,1,((#12267,#12268),(#12269,#12270),
(#12271,#12272),(#12273,#12274),(#12275,#12276),(#12277,#12278),(#12279,
#12280),(#12281,#12282),(#12283,#12284),(#12285,#12286),(#12287,#12288),
(#12289,#12290),(#12291,#12292),(#12293,#12294),(#12295,#12296),(#12297,
#12298),(#12299,#12300),(#12301,#12302),(#12303,#12304),(#12305,#12306),
(#12307,#12308),(#12309,#12310),(#12311,#12312)),.UNSPECIFIED.,.F.,.F.,
 .F.,(4,1,1,1,1,1,1,1,1,1,1,1,1,1,1,1,1,1,1,1,4),(2,2),(0.,0.158672905823676,
0.243948927603829,0.322402868082049,0.394034727302036,0.458844505321287,
0.516832202217594,0.567997818099863,0.612341353127269,0.649862807545807,
0.680562181765468,0.695323448997602,0.706670671285856,0.717793322185029,
0.728712887095513,0.760515567641419,0.791692515756145,0.823806980266354,
0.859359395195979,0.901681047937578,0.967654618228659),(0.,0.839999999999999),
 .UNSPECIFIED.);
#203=B_SPLINE_SURFACE_WITH_KNOTS('',3,1,((#12316,#12317),(#12318,#12319),
(#12320,#12321),(#12322,#12323),(#12324,#12325),(#12326,#12327),(#12328,
#12329),(#12330,#12331),(#12332,#12333),(#12334,#12335),(#12336,#12337),
(#12338,#12339),(#12340,#12341),(#12342,#12343),(#12344,#12345),(#12346,
#12347),(#12348,#12349),(#12350,#12351),(#12352,#12353),(#12354,#12355),
(#12356,#12357),(#12358,#12359),(#12360,#12361)),.UNSPECIFIED.,.F.,.F.,
 .F.,(4,1,1,1,1,1,1,1,1,1,1,1,1,1,1,1,1,1,1,1,4),(2,2),(0.0323453817713401,
0.0983189520624214,0.14064060480402,0.176193019733645,0.208307484243854,
0.23948443235858,0.271287112904486,0.28220667781497,0.293329328714142,0.304676551002397,
0.319437818234531,0.350137192454192,0.38765864687273,0.432002181900136,
0.483167797782405,0.541155494678712,0.605965272697963,0.67759713191795,
0.75605107239617,0.841327094176323,1.),(0.,0.84),.UNSPECIFIED.);
#204=B_SPLINE_SURFACE_WITH_KNOTS('',3,1,((#12365,#12366),(#12367,#12368),
(#12369,#12370),(#12371,#12372),(#12373,#12374),(#12375,#12376),(#12377,
#12378),(#12379,#12380),(#12381,#12382),(#12383,#12384),(#12385,#12386),
(#12387,#12388),(#12389,#12390),(#12391,#12392),(#12393,#12394),(#12395,
#12396),(#12397,#12398),(#12399,#12400),(#12401,#12402),(#12403,#12404),
(#12405,#12406),(#12407,#12408),(#12409,#12410)),.UNSPECIFIED.,.F.,.F.,
 .F.,(4,1,1,1,1,1,1,1,1,1,1,1,1,1,1,1,1,1,1,1,4),(2,2),(0.,0.158672905823676,
0.243948927603829,0.322402868082049,0.394034727302036,0.458844505321287,
0.516832202217594,0.567997818099863,0.612341353127269,0.649862807545807,
0.680562181765468,0.695323448997602,0.706670671285856,0.717793322185029,
0.728712887095513,0.760515567641419,0.791692515756145,0.823806980266354,
0.859359395195979,0.901681047937578,0.967654618228659),(0.,0.839999999999999),
 .UNSPECIFIED.);
#205=B_SPLINE_SURFACE_WITH_KNOTS('',3,1,((#12414,#12415),(#12416,#12417),
(#12418,#12419),(#12420,#12421),(#12422,#12423),(#12424,#12425),(#12426,
#12427),(#12428,#12429),(#12430,#12431),(#12432,#12433),(#12434,#12435),
(#12436,#12437),(#12438,#12439),(#12440,#12441),(#12442,#12443),(#12444,
#12445),(#12446,#12447),(#12448,#12449),(#12450,#12451),(#12452,#12453),
(#12454,#12455),(#12456,#12457),(#12458,#12459)),.UNSPECIFIED.,.F.,.F.,
 .F.,(4,1,1,1,1,1,1,1,1,1,1,1,1,1,1,1,1,1,1,1,4),(2,2),(0.0323453817713401,
0.0983189520624214,0.14064060480402,0.176193019733645,0.208307484243854,
0.23948443235858,0.271287112904486,0.28220667781497,0.293329328714142,0.304676551002397,
0.319437818234531,0.350137192454192,0.38765864687273,0.432002181900136,
0.483167797782405,0.541155494678712,0.605965272697963,0.67759713191795,
0.75605107239617,0.841327094176323,1.),(0.,0.84),.UNSPECIFIED.);
#206=B_SPLINE_SURFACE_WITH_KNOTS('',3,1,((#12463,#12464),(#12465,#12466),
(#12467,#12468),(#12469,#12470),(#12471,#12472),(#12473,#12474),(#12475,
#12476),(#12477,#12478),(#12479,#12480),(#12481,#12482),(#12483,#12484),
(#12485,#12486),(#12487,#12488),(#12489,#12490),(#12491,#12492),(#12493,
#12494),(#12495,#12496),(#12497,#12498),(#12499,#12500),(#12501,#12502),
(#12503,#12504),(#12505,#12506),(#12507,#12508)),.UNSPECIFIED.,.F.,.F.,
 .F.,(4,1,1,1,1,1,1,1,1,1,1,1,1,1,1,1,1,1,1,1,4),(2,2),(0.,0.158672905823676,
0.243948927603829,0.322402868082049,0.394034727302036,0.458844505321287,
0.516832202217594,0.567997818099863,0.612341353127269,0.649862807545807,
0.680562181765468,0.695323448997602,0.706670671285856,0.717793322185029,
0.728712887095513,0.760515567641419,0.791692515756145,0.823806980266354,
0.859359395195979,0.901681047937578,0.967654618228659),(0.,0.839999999999999),
 .UNSPECIFIED.);
#207=B_SPLINE_CURVE_WITH_KNOTS('',3,(#8481,#8482,#8483,#8484,#8485,#8486,
#8487,#8488,#8489,#8490,#8491,#8492,#8493,#8494,#8495,#8496,#8497,#8498,
#8499,#8500,#8501,#8502,#8503),.UNSPECIFIED.,.F.,.F.,(4,1,1,1,1,1,1,1,1,
1,1,1,1,1,1,1,1,1,1,1,4),(0.0323453817713401,0.0983189520624214,0.14064060480402,
0.176193019733645,0.208307484243854,0.23948443235858,0.271287112904486,
0.28220667781497,0.293329328714142,0.304676551002397,0.319437818234531,
0.350137192454192,0.38765864687273,0.432002181900136,0.483167797782405,
0.541155494678712,0.605965272697963,0.67759713191795,0.75605107239617,0.841327094176323,
1.),.UNSPECIFIED.);
#208=B_SPLINE_CURVE_WITH_KNOTS('',3,(#8507,#8508,#8509,#8510,#8511,#8512,
#8513,#8514,#8515,#8516,#8517,#8518,#8519,#8520,#8521,#8522,#8523,#8524,
#8525,#8526,#8527,#8528,#8529),.UNSPECIFIED.,.F.,.F.,(4,1,1,1,1,1,1,1,1,
1,1,1,1,1,1,1,1,1,1,1,4),(0.,0.158672905823676,0.243948927603829,0.322402868082049,
0.394034727302036,0.458844505321287,0.516832202217594,0.567997818099863,
0.612341353127269,0.649862807545807,0.680562181765468,0.695323448997602,
0.706670671285856,0.717793322185029,0.728712887095513,0.760515567641419,
0.791692515756145,0.823806980266354,0.859359395195979,0.901681047937578,
0.967654618228659),.UNSPECIFIED.);
#209=B_SPLINE_CURVE_WITH_KNOTS('',3,(#8533,#8534,#8535,#8536,#8537,#8538,
#8539,#8540,#8541,#8542,#8543,#8544,#8545,#8546,#8547,#8548,#8549,#8550,
#8551,#8552,#8553,#8554,#8555),.UNSPECIFIED.,.F.,.F.,(4,1,1,1,1,1,1,1,1,
1,1,1,1,1,1,1,1,1,1,1,4),(0.0323453817713401,0.0983189520624214,0.14064060480402,
0.176193019733645,0.208307484243854,0.23948443235858,0.271287112904486,
0.28220667781497,0.293329328714142,0.304676551002397,0.319437818234531,
0.350137192454192,0.38765864687273,0.432002181900136,0.483167797782405,
0.541155494678712,0.605965272697963,0.67759713191795,0.75605107239617,0.841327094176323,
1.),.UNSPECIFIED.);
#210=B_SPLINE_CURVE_WITH_KNOTS('',3,(#8559,#8560,#8561,#8562,#8563,#8564,
#8565,#8566,#8567,#8568,#8569,#8570,#8571,#8572,#8573,#8574,#8575,#8576,
#8577,#8578,#8579,#8580,#8581),.UNSPECIFIED.,.F.,.F.,(4,1,1,1,1,1,1,1,1,
1,1,1,1,1,1,1,1,1,1,1,4),(0.,0.158672905823676,0.243948927603829,0.322402868082049,
0.394034727302036,0.458844505321287,0.516832202217594,0.567997818099863,
0.612341353127269,0.649862807545807,0.680562181765468,0.695323448997602,
0.706670671285856,0.717793322185029,0.728712887095513,0.760515567641419,
0.791692515756145,0.823806980266354,0.859359395195979,0.901681047937578,
0.967654618228659),.UNSPECIFIED.);
#211=B_SPLINE_CURVE_WITH_KNOTS('',3,(#8585,#8586,#8587,#8588,#8589,#8590,
#8591,#8592,#8593,#8594,#8595,#8596,#8597,#8598,#8599,#8600,#8601,#8602,
#8603,#8604,#8605,#8606,#8607),.UNSPECIFIED.,.F.,.F.,(4,1,1,1,1,1,1,1,1,
1,1,1,1,1,1,1,1,1,1,1,4),(0.0323453817713401,0.0983189520624214,0.14064060480402,
0.176193019733645,0.208307484243854,0.23948443235858,0.271287112904486,
0.28220667781497,0.293329328714142,0.304676551002397,0.319437818234531,
0.350137192454192,0.38765864687273,0.432002181900136,0.483167797782405,
0.541155494678712,0.605965272697963,0.67759713191795,0.75605107239617,0.841327094176323,
1.),.UNSPECIFIED.);
#212=B_SPLINE_CURVE_WITH_KNOTS('',3,(#8611,#8612,#8613,#8614,#8615,#8616,
#8617,#8618,#8619,#8620,#8621,#8622,#8623,#8624,#8625,#8626,#8627,#8628,
#8629,#8630,#8631,#8632,#8633),.UNSPECIFIED.,.F.,.F.,(4,1,1,1,1,1,1,1,1,
1,1,1,1,1,1,1,1,1,1,1,4),(0.,0.158672905823676,0.243948927603829,0.322402868082049,
0.394034727302036,0.458844505321287,0.516832202217594,0.567997818099863,
0.612341353127269,0.649862807545807,0.680562181765468,0.695323448997602,
0.706670671285856,0.717793322185029,0.728712887095513,0.760515567641419,
0.791692515756145,0.823806980266354,0.859359395195979,0.901681047937578,
0.967654618228659),.UNSPECIFIED.);
#213=B_SPLINE_CURVE_WITH_KNOTS('',3,(#8637,#8638,#8639,#8640,#8641,#8642,
#8643,#8644,#8645,#8646,#8647,#8648,#8649,#8650,#8651,#8652,#8653,#8654,
#8655,#8656,#8657,#8658,#8659),.UNSPECIFIED.,.F.,.F.,(4,1,1,1,1,1,1,1,1,
1,1,1,1,1,1,1,1,1,1,1,4),(0.0323453817713401,0.0983189520624214,0.14064060480402,
0.176193019733645,0.208307484243854,0.23948443235858,0.271287112904486,
0.28220667781497,0.293329328714142,0.304676551002397,0.319437818234531,
0.350137192454192,0.38765864687273,0.432002181900136,0.483167797782405,
0.541155494678712,0.605965272697963,0.67759713191795,0.75605107239617,0.841327094176323,
1.),.UNSPECIFIED.);
#214=B_SPLINE_CURVE_WITH_KNOTS('',3,(#8663,#8664,#8665,#8666,#8667,#8668,
#8669,#8670,#8671,#8672,#8673,#8674,#8675,#8676,#8677,#8678,#8679,#8680,
#8681,#8682,#8683,#8684,#8685),.UNSPECIFIED.,.F.,.F.,(4,1,1,1,1,1,1,1,1,
1,1,1,1,1,1,1,1,1,1,1,4),(0.,0.158672905823676,0.243948927603829,0.322402868082049,
0.394034727302036,0.458844505321287,0.516832202217594,0.567997818099863,
0.612341353127269,0.649862807545807,0.680562181765468,0.695323448997602,
0.706670671285856,0.717793322185029,0.728712887095513,0.760515567641419,
0.791692515756145,0.823806980266354,0.859359395195979,0.901681047937578,
0.967654618228659),.UNSPECIFIED.);
#215=B_SPLINE_CURVE_WITH_KNOTS('',3,(#8689,#8690,#8691,#8692,#8693,#8694,
#8695,#8696,#8697,#8698,#8699,#8700,#8701,#8702,#8703,#8704,#8705,#8706,
#8707,#8708,#8709,#8710,#8711),.UNSPECIFIED.,.F.,.F.,(4,1,1,1,1,1,1,1,1,
1,1,1,1,1,1,1,1,1,1,1,4),(0.0323453817713401,0.0983189520624214,0.14064060480402,
0.176193019733645,0.208307484243854,0.23948443235858,0.271287112904486,
0.28220667781497,0.293329328714142,0.304676551002397,0.319437818234531,
0.350137192454192,0.38765864687273,0.432002181900136,0.483167797782405,
0.541155494678712,0.605965272697963,0.67759713191795,0.75605107239617,0.841327094176323,
1.),.UNSPECIFIED.);
#216=B_SPLINE_CURVE_WITH_KNOTS('',3,(#8715,#8716,#8717,#8718,#8719,#8720,
#8721,#8722,#8723,#8724,#8725,#8726,#8727,#8728,#8729,#8730,#8731,#8732,
#8733,#8734,#8735,#8736,#8737),.UNSPECIFIED.,.F.,.F.,(4,1,1,1,1,1,1,1,1,
1,1,1,1,1,1,1,1,1,1,1,4),(0.,0.158672905823676,0.243948927603829,0.322402868082049,
0.394034727302036,0.458844505321287,0.516832202217594,0.567997818099863,
0.612341353127269,0.649862807545807,0.680562181765468,0.695323448997602,
0.706670671285856,0.717793322185029,0.728712887095513,0.760515567641419,
0.791692515756145,0.823806980266354,0.859359395195979,0.901681047937578,
0.967654618228659),.UNSPECIFIED.);
#217=B_SPLINE_CURVE_WITH_KNOTS('',3,(#8741,#8742,#8743,#8744,#8745,#8746,
#8747,#8748,#8749,#8750,#8751,#8752,#8753,#8754,#8755,#8756,#8757,#8758,
#8759,#8760,#8761,#8762,#8763),.UNSPECIFIED.,.F.,.F.,(4,1,1,1,1,1,1,1,1,
1,1,1,1,1,1,1,1,1,1,1,4),(0.0323453817713401,0.0983189520624214,0.14064060480402,
0.176193019733645,0.208307484243854,0.23948443235858,0.271287112904486,
0.28220667781497,0.293329328714142,0.304676551002397,0.319437818234531,
0.350137192454192,0.38765864687273,0.432002181900136,0.483167797782405,
0.541155494678712,0.605965272697963,0.67759713191795,0.75605107239617,0.841327094176323,
1.),.UNSPECIFIED.);
#218=B_SPLINE_CURVE_WITH_KNOTS('',3,(#8767,#8768,#8769,#8770,#8771,#8772,
#8773,#8774,#8775,#8776,#8777,#8778,#8779,#8780,#8781,#8782,#8783,#8784,
#8785,#8786,#8787,#8788,#8789),.UNSPECIFIED.,.F.,.F.,(4,1,1,1,1,1,1,1,1,
1,1,1,1,1,1,1,1,1,1,1,4),(0.,0.158672905823676,0.243948927603829,0.322402868082049,
0.394034727302036,0.458844505321287,0.516832202217594,0.567997818099863,
0.612341353127269,0.649862807545807,0.680562181765468,0.695323448997602,
0.706670671285856,0.717793322185029,0.728712887095513,0.760515567641419,
0.791692515756145,0.823806980266354,0.859359395195979,0.901681047937578,
0.967654618228659),.UNSPECIFIED.);
#219=B_SPLINE_CURVE_WITH_KNOTS('',3,(#8793,#8794,#8795,#8796,#8797,#8798,
#8799,#8800,#8801,#8802,#8803,#8804,#8805,#8806,#8807,#8808,#8809,#8810,
#8811,#8812,#8813,#8814,#8815),.UNSPECIFIED.,.F.,.F.,(4,1,1,1,1,1,1,1,1,
1,1,1,1,1,1,1,1,1,1,1,4),(0.0323453817713401,0.0983189520624214,0.14064060480402,
0.176193019733645,0.208307484243854,0.23948443235858,0.271287112904486,
0.28220667781497,0.293329328714142,0.304676551002397,0.319437818234531,
0.350137192454192,0.38765864687273,0.432002181900136,0.483167797782405,
0.541155494678712,0.605965272697963,0.67759713191795,0.75605107239617,0.841327094176323,
1.),.UNSPECIFIED.);
#220=B_SPLINE_CURVE_WITH_KNOTS('',3,(#8819,#8820,#8821,#8822,#8823,#8824,
#8825,#8826,#8827,#8828,#8829,#8830,#8831,#8832,#8833,#8834,#8835,#8836,
#8837,#8838,#8839,#8840,#8841),.UNSPECIFIED.,.F.,.F.,(4,1,1,1,1,1,1,1,1,
1,1,1,1,1,1,1,1,1,1,1,4),(0.,0.158672905823676,0.243948927603829,0.322402868082049,
0.394034727302036,0.458844505321287,0.516832202217594,0.567997818099863,
0.612341353127269,0.649862807545807,0.680562181765468,0.695323448997602,
0.706670671285856,0.717793322185029,0.728712887095513,0.760515567641419,
0.791692515756145,0.823806980266354,0.859359395195979,0.901681047937578,
0.967654618228659),.UNSPECIFIED.);
#221=B_SPLINE_CURVE_WITH_KNOTS('',3,(#8845,#8846,#8847,#8848,#8849,#8850,
#8851,#8852,#8853,#8854,#8855,#8856,#8857,#8858,#8859,#8860,#8861,#8862,
#8863,#8864,#8865,#8866,#8867),.UNSPECIFIED.,.F.,.F.,(4,1,1,1,1,1,1,1,1,
1,1,1,1,1,1,1,1,1,1,1,4),(0.0323453817713401,0.0983189520624214,0.14064060480402,
0.176193019733645,0.208307484243854,0.23948443235858,0.271287112904486,
0.28220667781497,0.293329328714142,0.304676551002397,0.319437818234531,
0.350137192454192,0.38765864687273,0.432002181900136,0.483167797782405,
0.541155494678712,0.605965272697963,0.67759713191795,0.75605107239617,0.841327094176323,
1.),.UNSPECIFIED.);
#222=B_SPLINE_CURVE_WITH_KNOTS('',3,(#8871,#8872,#8873,#8874,#8875,#8876,
#8877,#8878,#8879,#8880,#8881,#8882,#8883,#8884,#8885,#8886,#8887,#8888,
#8889,#8890,#8891,#8892,#8893),.UNSPECIFIED.,.F.,.F.,(4,1,1,1,1,1,1,1,1,
1,1,1,1,1,1,1,1,1,1,1,4),(0.,0.158672905823676,0.243948927603829,0.322402868082049,
0.394034727302036,0.458844505321287,0.516832202217594,0.567997818099863,
0.612341353127269,0.649862807545807,0.680562181765468,0.695323448997602,
0.706670671285856,0.717793322185029,0.728712887095513,0.760515567641419,
0.791692515756145,0.823806980266354,0.859359395195979,0.901681047937578,
0.967654618228659),.UNSPECIFIED.);
#223=B_SPLINE_CURVE_WITH_KNOTS('',3,(#8897,#8898,#8899,#8900,#8901,#8902,
#8903,#8904,#8905,#8906,#8907,#8908,#8909,#8910,#8911,#8912,#8913,#8914,
#8915,#8916,#8917,#8918,#8919),.UNSPECIFIED.,.F.,.F.,(4,1,1,1,1,1,1,1,1,
1,1,1,1,1,1,1,1,1,1,1,4),(0.0323453817713401,0.0983189520624214,0.14064060480402,
0.176193019733645,0.208307484243854,0.23948443235858,0.271287112904486,
0.28220667781497,0.293329328714142,0.304676551002397,0.319437818234531,
0.350137192454192,0.38765864687273,0.432002181900136,0.483167797782405,
0.541155494678712,0.605965272697963,0.67759713191795,0.75605107239617,0.841327094176323,
1.),.UNSPECIFIED.);
#224=B_SPLINE_CURVE_WITH_KNOTS('',3,(#8922,#8923,#8924,#8925,#8926,#8927,
#8928,#8929,#8930,#8931,#8932,#8933,#8934,#8935,#8936,#8937,#8938,#8939,
#8940,#8941,#8942,#8943,#8944),.UNSPECIFIED.,.F.,.F.,(4,1,1,1,1,1,1,1,1,
1,1,1,1,1,1,1,1,1,1,1,4),(0.,0.158672905823676,0.243948927603829,0.322402868082049,
0.394034727302036,0.458844505321287,0.516832202217594,0.567997818099863,
0.612341353127269,0.649862807545807,0.680562181765468,0.695323448997602,
0.706670671285856,0.717793322185029,0.728712887095513,0.760515567641419,
0.791692515756145,0.823806980266354,0.859359395195979,0.901681047937578,
0.967654618228659),.UNSPECIFIED.);
#225=B_SPLINE_CURVE_WITH_KNOTS('',3,(#8946,#8947,#8948,#8949,#8950,#8951,
#8952,#8953,#8954,#8955,#8956,#8957,#8958,#8959,#8960,#8961,#8962,#8963,
#8964,#8965,#8966,#8967,#8968),.UNSPECIFIED.,.F.,.F.,(4,1,1,1,1,1,1,1,1,
1,1,1,1,1,1,1,1,1,1,1,4),(0.0323453817713401,0.0983189520624214,0.14064060480402,
0.176193019733645,0.208307484243854,0.23948443235858,0.271287112904486,
0.28220667781497,0.293329328714142,0.304676551002397,0.319437818234531,
0.350137192454192,0.38765864687273,0.432002181900136,0.483167797782405,
0.541155494678712,0.605965272697963,0.67759713191795,0.75605107239617,0.841327094176323,
1.),.UNSPECIFIED.);
#226=B_SPLINE_CURVE_WITH_KNOTS('',3,(#8972,#8973,#8974,#8975,#8976,#8977,
#8978,#8979,#8980,#8981,#8982,#8983,#8984,#8985,#8986,#8987,#8988,#8989,
#8990,#8991,#8992,#8993,#8994),.UNSPECIFIED.,.F.,.F.,(4,1,1,1,1,1,1,1,1,
1,1,1,1,1,1,1,1,1,1,1,4),(0.,0.158672905823676,0.243948927603829,0.322402868082049,
0.394034727302036,0.458844505321287,0.516832202217594,0.567997818099863,
0.612341353127269,0.649862807545807,0.680562181765468,0.695323448997602,
0.706670671285856,0.717793322185029,0.728712887095513,0.760515567641419,
0.791692515756145,0.823806980266354,0.859359395195979,0.901681047937578,
0.967654618228659),.UNSPECIFIED.);
#227=B_SPLINE_CURVE_WITH_KNOTS('',3,(#8998,#8999,#9000,#9001,#9002,#9003,
#9004,#9005,#9006,#9007,#9008,#9009,#9010,#9011,#9012,#9013,#9014,#9015,
#9016,#9017,#9018,#9019,#9020),.UNSPECIFIED.,.F.,.F.,(4,1,1,1,1,1,1,1,1,
1,1,1,1,1,1,1,1,1,1,1,4),(0.0323453817713401,0.0983189520624214,0.14064060480402,
0.176193019733645,0.208307484243854,0.23948443235858,0.271287112904486,
0.28220667781497,0.293329328714142,0.304676551002397,0.319437818234531,
0.350137192454192,0.38765864687273,0.432002181900136,0.483167797782405,
0.541155494678712,0.605965272697963,0.67759713191795,0.75605107239617,0.841327094176323,
1.),.UNSPECIFIED.);
#228=B_SPLINE_CURVE_WITH_KNOTS('',3,(#9024,#9025,#9026,#9027,#9028,#9029,
#9030,#9031,#9032,#9033,#9034,#9035,#9036,#9037,#9038,#9039,#9040,#9041,
#9042,#9043,#9044,#9045,#9046),.UNSPECIFIED.,.F.,.F.,(4,1,1,1,1,1,1,1,1,
1,1,1,1,1,1,1,1,1,1,1,4),(0.,0.158672905823676,0.243948927603829,0.322402868082049,
0.394034727302036,0.458844505321287,0.516832202217594,0.567997818099863,
0.612341353127269,0.649862807545807,0.680562181765468,0.695323448997602,
0.706670671285856,0.717793322185029,0.728712887095513,0.760515567641419,
0.791692515756145,0.823806980266354,0.859359395195979,0.901681047937578,
0.967654618228659),.UNSPECIFIED.);
#229=B_SPLINE_CURVE_WITH_KNOTS('',3,(#9050,#9051,#9052,#9053,#9054,#9055,
#9056,#9057,#9058,#9059,#9060,#9061,#9062,#9063,#9064,#9065,#9066,#9067,
#9068,#9069,#9070,#9071,#9072),.UNSPECIFIED.,.F.,.F.,(4,1,1,1,1,1,1,1,1,
1,1,1,1,1,1,1,1,1,1,1,4),(0.0323453817713401,0.0983189520624214,0.14064060480402,
0.176193019733645,0.208307484243854,0.23948443235858,0.271287112904486,
0.28220667781497,0.293329328714142,0.304676551002397,0.319437818234531,
0.350137192454192,0.38765864687273,0.432002181900136,0.483167797782405,
0.541155494678712,0.605965272697963,0.67759713191795,0.75605107239617,0.841327094176323,
1.),.UNSPECIFIED.);
#230=B_SPLINE_CURVE_WITH_KNOTS('',3,(#9076,#9077,#9078,#9079,#9080,#9081,
#9082,#9083,#9084,#9085,#9086,#9087,#9088,#9089,#9090,#9091,#9092,#9093,
#9094,#9095,#9096,#9097,#9098),.UNSPECIFIED.,.F.,.F.,(4,1,1,1,1,1,1,1,1,
1,1,1,1,1,1,1,1,1,1,1,4),(0.,0.158672905823676,0.243948927603829,0.322402868082049,
0.394034727302036,0.458844505321287,0.516832202217594,0.567997818099863,
0.612341353127269,0.649862807545807,0.680562181765468,0.695323448997602,
0.706670671285856,0.717793322185029,0.728712887095513,0.760515567641419,
0.791692515756145,0.823806980266354,0.859359395195979,0.901681047937578,
0.967654618228659),.UNSPECIFIED.);
#231=B_SPLINE_CURVE_WITH_KNOTS('',3,(#9102,#9103,#9104,#9105,#9106,#9107,
#9108,#9109,#9110,#9111,#9112,#9113,#9114,#9115,#9116,#9117,#9118,#9119,
#9120,#9121,#9122,#9123,#9124),.UNSPECIFIED.,.F.,.F.,(4,1,1,1,1,1,1,1,1,
1,1,1,1,1,1,1,1,1,1,1,4),(0.0323453817713401,0.0983189520624214,0.14064060480402,
0.176193019733645,0.208307484243854,0.23948443235858,0.271287112904486,
0.28220667781497,0.293329328714142,0.304676551002397,0.319437818234531,
0.350137192454192,0.38765864687273,0.432002181900136,0.483167797782405,
0.541155494678712,0.605965272697963,0.67759713191795,0.75605107239617,0.841327094176323,
1.),.UNSPECIFIED.);
#232=B_SPLINE_CURVE_WITH_KNOTS('',3,(#9128,#9129,#9130,#9131,#9132,#9133,
#9134,#9135,#9136,#9137,#9138,#9139,#9140,#9141,#9142,#9143,#9144,#9145,
#9146,#9147,#9148,#9149,#9150),.UNSPECIFIED.,.F.,.F.,(4,1,1,1,1,1,1,1,1,
1,1,1,1,1,1,1,1,1,1,1,4),(0.,0.158672905823676,0.243948927603829,0.322402868082049,
0.394034727302036,0.458844505321287,0.516832202217594,0.567997818099863,
0.612341353127269,0.649862807545807,0.680562181765468,0.695323448997602,
0.706670671285856,0.717793322185029,0.728712887095513,0.760515567641419,
0.791692515756145,0.823806980266354,0.859359395195979,0.901681047937578,
0.967654618228659),.UNSPECIFIED.);
#233=B_SPLINE_CURVE_WITH_KNOTS('',3,(#9154,#9155,#9156,#9157,#9158,#9159,
#9160,#9161,#9162,#9163,#9164,#9165,#9166,#9167,#9168,#9169,#9170,#9171,
#9172,#9173,#9174,#9175,#9176),.UNSPECIFIED.,.F.,.F.,(4,1,1,1,1,1,1,1,1,
1,1,1,1,1,1,1,1,1,1,1,4),(0.0323453817713401,0.0983189520624214,0.14064060480402,
0.176193019733645,0.208307484243854,0.23948443235858,0.271287112904486,
0.28220667781497,0.293329328714142,0.304676551002397,0.319437818234531,
0.350137192454192,0.38765864687273,0.432002181900136,0.483167797782405,
0.541155494678712,0.605965272697963,0.67759713191795,0.75605107239617,0.841327094176323,
1.),.UNSPECIFIED.);
#234=B_SPLINE_CURVE_WITH_KNOTS('',3,(#9180,#9181,#9182,#9183,#9184,#9185,
#9186,#9187,#9188,#9189,#9190,#9191,#9192,#9193,#9194,#9195,#9196,#9197,
#9198,#9199,#9200,#9201,#9202),.UNSPECIFIED.,.F.,.F.,(4,1,1,1,1,1,1,1,1,
1,1,1,1,1,1,1,1,1,1,1,4),(0.,0.158672905823676,0.243948927603829,0.322402868082049,
0.394034727302036,0.458844505321287,0.516832202217594,0.567997818099863,
0.612341353127269,0.649862807545807,0.680562181765468,0.695323448997602,
0.706670671285856,0.717793322185029,0.728712887095513,0.760515567641419,
0.791692515756145,0.823806980266354,0.859359395195979,0.901681047937578,
0.967654618228659),.UNSPECIFIED.);
#235=B_SPLINE_CURVE_WITH_KNOTS('',3,(#9206,#9207,#9208,#9209,#9210,#9211,
#9212,#9213,#9214,#9215,#9216,#9217,#9218,#9219,#9220,#9221,#9222,#9223,
#9224,#9225,#9226,#9227,#9228),.UNSPECIFIED.,.F.,.F.,(4,1,1,1,1,1,1,1,1,
1,1,1,1,1,1,1,1,1,1,1,4),(0.0323453817713401,0.0983189520624214,0.14064060480402,
0.176193019733645,0.208307484243854,0.23948443235858,0.271287112904486,
0.28220667781497,0.293329328714142,0.304676551002397,0.319437818234531,
0.350137192454192,0.38765864687273,0.432002181900136,0.483167797782405,
0.541155494678712,0.605965272697963,0.67759713191795,0.75605107239617,0.841327094176323,
1.),.UNSPECIFIED.);
#236=B_SPLINE_CURVE_WITH_KNOTS('',3,(#9232,#9233,#9234,#9235,#9236,#9237,
#9238,#9239,#9240,#9241,#9242,#9243,#9244,#9245,#9246,#9247,#9248,#9249,
#9250,#9251,#9252,#9253,#9254),.UNSPECIFIED.,.F.,.F.,(4,1,1,1,1,1,1,1,1,
1,1,1,1,1,1,1,1,1,1,1,4),(0.,0.158672905823676,0.243948927603829,0.322402868082049,
0.394034727302036,0.458844505321287,0.516832202217594,0.567997818099863,
0.612341353127269,0.649862807545807,0.680562181765468,0.695323448997602,
0.706670671285856,0.717793322185029,0.728712887095513,0.760515567641419,
0.791692515756145,0.823806980266354,0.859359395195979,0.901681047937578,
0.967654618228659),.UNSPECIFIED.);
#237=B_SPLINE_CURVE_WITH_KNOTS('',3,(#9258,#9259,#9260,#9261,#9262,#9263,
#9264,#9265,#9266,#9267,#9268,#9269,#9270,#9271,#9272,#9273,#9274,#9275,
#9276,#9277,#9278,#9279,#9280),.UNSPECIFIED.,.F.,.F.,(4,1,1,1,1,1,1,1,1,
1,1,1,1,1,1,1,1,1,1,1,4),(0.0323453817713401,0.0983189520624214,0.14064060480402,
0.176193019733645,0.208307484243854,0.23948443235858,0.271287112904486,
0.28220667781497,0.293329328714142,0.304676551002397,0.319437818234531,
0.350137192454192,0.38765864687273,0.432002181900136,0.483167797782405,
0.541155494678712,0.605965272697963,0.67759713191795,0.75605107239617,0.841327094176323,
1.),.UNSPECIFIED.);
#238=B_SPLINE_CURVE_WITH_KNOTS('',3,(#9284,#9285,#9286,#9287,#9288,#9289,
#9290,#9291,#9292,#9293,#9294,#9295,#9296,#9297,#9298,#9299,#9300,#9301,
#9302,#9303,#9304,#9305,#9306),.UNSPECIFIED.,.F.,.F.,(4,1,1,1,1,1,1,1,1,
1,1,1,1,1,1,1,1,1,1,1,4),(0.,0.158672905823676,0.243948927603829,0.322402868082049,
0.394034727302036,0.458844505321287,0.516832202217594,0.567997818099863,
0.612341353127269,0.649862807545807,0.680562181765468,0.695323448997602,
0.706670671285856,0.717793322185029,0.728712887095513,0.760515567641419,
0.791692515756145,0.823806980266354,0.859359395195979,0.901681047937578,
0.967654618228659),.UNSPECIFIED.);
#239=B_SPLINE_CURVE_WITH_KNOTS('',3,(#9310,#9311,#9312,#9313,#9314,#9315,
#9316,#9317,#9318,#9319,#9320,#9321,#9322,#9323,#9324,#9325,#9326,#9327,
#9328,#9329,#9330,#9331,#9332),.UNSPECIFIED.,.F.,.F.,(4,1,1,1,1,1,1,1,1,
1,1,1,1,1,1,1,1,1,1,1,4),(0.0323453817713401,0.0983189520624214,0.14064060480402,
0.176193019733645,0.208307484243854,0.23948443235858,0.271287112904486,
0.28220667781497,0.293329328714142,0.304676551002397,0.319437818234531,
0.350137192454192,0.38765864687273,0.432002181900136,0.483167797782405,
0.541155494678712,0.605965272697963,0.67759713191795,0.75605107239617,0.841327094176323,
1.),.UNSPECIFIED.);
#240=B_SPLINE_CURVE_WITH_KNOTS('',3,(#9336,#9337,#9338,#9339,#9340,#9341,
#9342,#9343,#9344,#9345,#9346,#9347,#9348,#9349,#9350,#9351,#9352,#9353,
#9354,#9355,#9356,#9357,#9358),.UNSPECIFIED.,.F.,.F.,(4,1,1,1,1,1,1,1,1,
1,1,1,1,1,1,1,1,1,1,1,4),(0.,0.158672905823676,0.243948927603829,0.322402868082049,
0.394034727302036,0.458844505321287,0.516832202217594,0.567997818099863,
0.612341353127269,0.649862807545807,0.680562181765468,0.695323448997602,
0.706670671285856,0.717793322185029,0.728712887095513,0.760515567641419,
0.791692515756145,0.823806980266354,0.859359395195979,0.901681047937578,
0.967654618228659),.UNSPECIFIED.);
#241=B_SPLINE_CURVE_WITH_KNOTS('',3,(#9362,#9363,#9364,#9365,#9366,#9367,
#9368,#9369,#9370,#9371,#9372,#9373,#9374,#9375,#9376,#9377,#9378,#9379,
#9380,#9381,#9382,#9383,#9384),.UNSPECIFIED.,.F.,.F.,(4,1,1,1,1,1,1,1,1,
1,1,1,1,1,1,1,1,1,1,1,4),(0.0323453817713401,0.0983189520624214,0.14064060480402,
0.176193019733645,0.208307484243854,0.23948443235858,0.271287112904486,
0.28220667781497,0.293329328714142,0.304676551002397,0.319437818234531,
0.350137192454192,0.38765864687273,0.432002181900136,0.483167797782405,
0.541155494678712,0.605965272697963,0.67759713191795,0.75605107239617,0.841327094176323,
1.),.UNSPECIFIED.);
#242=B_SPLINE_CURVE_WITH_KNOTS('',3,(#9388,#9389,#9390,#9391,#9392,#9393,
#9394,#9395,#9396,#9397,#9398,#9399,#9400,#9401,#9402,#9403,#9404,#9405,
#9406,#9407,#9408,#9409,#9410),.UNSPECIFIED.,.F.,.F.,(4,1,1,1,1,1,1,1,1,
1,1,1,1,1,1,1,1,1,1,1,4),(0.,0.158672905823676,0.243948927603829,0.322402868082049,
0.394034727302036,0.458844505321287,0.516832202217594,0.567997818099863,
0.612341353127269,0.649862807545807,0.680562181765468,0.695323448997602,
0.706670671285856,0.717793322185029,0.728712887095513,0.760515567641419,
0.791692515756145,0.823806980266354,0.859359395195979,0.901681047937578,
0.967654618228659),.UNSPECIFIED.);
#243=B_SPLINE_CURVE_WITH_KNOTS('',3,(#9414,#9415,#9416,#9417,#9418,#9419,
#9420,#9421,#9422,#9423,#9424,#9425,#9426,#9427,#9428,#9429,#9430,#9431,
#9432,#9433,#9434,#9435,#9436),.UNSPECIFIED.,.F.,.F.,(4,1,1,1,1,1,1,1,1,
1,1,1,1,1,1,1,1,1,1,1,4),(0.0323453817713401,0.0983189520624214,0.14064060480402,
0.176193019733645,0.208307484243854,0.23948443235858,0.271287112904486,
0.28220667781497,0.293329328714142,0.304676551002397,0.319437818234531,
0.350137192454192,0.38765864687273,0.432002181900136,0.483167797782405,
0.541155494678712,0.605965272697963,0.67759713191795,0.75605107239617,0.841327094176323,
1.),.UNSPECIFIED.);
#244=B_SPLINE_CURVE_WITH_KNOTS('',3,(#9440,#9441,#9442,#9443,#9444,#9445,
#9446,#9447,#9448,#9449,#9450,#9451,#9452,#9453,#9454,#9455,#9456,#9457,
#9458,#9459,#9460,#9461,#9462),.UNSPECIFIED.,.F.,.F.,(4,1,1,1,1,1,1,1,1,
1,1,1,1,1,1,1,1,1,1,1,4),(0.,0.158672905823676,0.243948927603829,0.322402868082049,
0.394034727302036,0.458844505321287,0.516832202217594,0.567997818099863,
0.612341353127269,0.649862807545807,0.680562181765468,0.695323448997602,
0.706670671285856,0.717793322185029,0.728712887095513,0.760515567641419,
0.791692515756145,0.823806980266354,0.859359395195979,0.901681047937578,
0.967654618228659),.UNSPECIFIED.);
#245=B_SPLINE_CURVE_WITH_KNOTS('',3,(#9466,#9467,#9468,#9469,#9470,#9471,
#9472,#9473,#9474,#9475,#9476,#9477,#9478,#9479,#9480,#9481,#9482,#9483,
#9484,#9485,#9486,#9487,#9488),.UNSPECIFIED.,.F.,.F.,(4,1,1,1,1,1,1,1,1,
1,1,1,1,1,1,1,1,1,1,1,4),(0.0323453817713401,0.0983189520624214,0.14064060480402,
0.176193019733645,0.208307484243854,0.23948443235858,0.271287112904486,
0.28220667781497,0.293329328714142,0.304676551002397,0.319437818234531,
0.350137192454192,0.38765864687273,0.432002181900136,0.483167797782405,
0.541155494678712,0.605965272697963,0.67759713191795,0.75605107239617,0.841327094176323,
1.),.UNSPECIFIED.);
#246=B_SPLINE_CURVE_WITH_KNOTS('',3,(#9492,#9493,#9494,#9495,#9496,#9497,
#9498,#9499,#9500,#9501,#9502,#9503,#9504,#9505,#9506,#9507,#9508,#9509,
#9510,#9511,#9512,#9513,#9514),.UNSPECIFIED.,.F.,.F.,(4,1,1,1,1,1,1,1,1,
1,1,1,1,1,1,1,1,1,1,1,4),(0.,0.158672905823676,0.243948927603829,0.322402868082049,
0.394034727302036,0.458844505321287,0.516832202217594,0.567997818099863,
0.612341353127269,0.649862807545807,0.680562181765468,0.695323448997602,
0.706670671285856,0.717793322185029,0.728712887095513,0.760515567641419,
0.791692515756145,0.823806980266354,0.859359395195979,0.901681047937578,
0.967654618228659),.UNSPECIFIED.);
#247=B_SPLINE_CURVE_WITH_KNOTS('',3,(#9519,#9520,#9521,#9522,#9523,#9524,
#9525,#9526,#9527,#9528,#9529,#9530,#9531,#9532,#9533,#9534,#9535,#9536,
#9537,#9538,#9539,#9540,#9541),.UNSPECIFIED.,.F.,.F.,(4,1,1,1,1,1,1,1,1,
1,1,1,1,1,1,1,1,1,1,1,4),(0.0323453817713401,0.0983189520624214,0.14064060480402,
0.176193019733645,0.208307484243854,0.23948443235858,0.271287112904486,
0.28220667781497,0.293329328714142,0.304676551002397,0.319437818234531,
0.350137192454192,0.38765864687273,0.432002181900136,0.483167797782405,
0.541155494678712,0.605965272697963,0.67759713191795,0.75605107239617,0.841327094176323,
1.),.UNSPECIFIED.);
#248=B_SPLINE_CURVE_WITH_KNOTS('',3,(#9545,#9546,#9547,#9548,#9549,#9550,
#9551,#9552,#9553,#9554,#9555,#9556,#9557,#9558,#9559,#9560,#9561,#9562,
#9563,#9564,#9565,#9566,#9567),.UNSPECIFIED.,.F.,.F.,(4,1,1,1,1,1,1,1,1,
1,1,1,1,1,1,1,1,1,1,1,4),(0.,0.158672905823676,0.243948927603829,0.322402868082049,
0.394034727302036,0.458844505321287,0.516832202217594,0.567997818099863,
0.612341353127269,0.649862807545807,0.680562181765468,0.695323448997602,
0.706670671285856,0.717793322185029,0.728712887095513,0.760515567641419,
0.791692515756145,0.823806980266354,0.859359395195979,0.901681047937578,
0.967654618228659),.UNSPECIFIED.);
#249=B_SPLINE_CURVE_WITH_KNOTS('',3,(#9571,#9572,#9573,#9574,#9575,#9576,
#9577,#9578,#9579,#9580,#9581,#9582,#9583,#9584,#9585,#9586,#9587,#9588,
#9589,#9590,#9591,#9592,#9593),.UNSPECIFIED.,.F.,.F.,(4,1,1,1,1,1,1,1,1,
1,1,1,1,1,1,1,1,1,1,1,4),(0.0323453817713401,0.0983189520624214,0.14064060480402,
0.176193019733645,0.208307484243854,0.23948443235858,0.271287112904486,
0.28220667781497,0.293329328714142,0.304676551002397,0.319437818234531,
0.350137192454192,0.38765864687273,0.432002181900136,0.483167797782405,
0.541155494678712,0.605965272697963,0.67759713191795,0.75605107239617,0.841327094176323,
1.),.UNSPECIFIED.);
#250=B_SPLINE_CURVE_WITH_KNOTS('',3,(#9597,#9598,#9599,#9600,#9601,#9602,
#9603,#9604,#9605,#9606,#9607,#9608,#9609,#9610,#9611,#9612,#9613,#9614,
#9615,#9616,#9617,#9618,#9619),.UNSPECIFIED.,.F.,.F.,(4,1,1,1,1,1,1,1,1,
1,1,1,1,1,1,1,1,1,1,1,4),(0.,0.158672905823676,0.243948927603829,0.322402868082049,
0.394034727302036,0.458844505321287,0.516832202217594,0.567997818099863,
0.612341353127269,0.649862807545807,0.680562181765468,0.695323448997602,
0.706670671285856,0.717793322185029,0.728712887095513,0.760515567641419,
0.791692515756145,0.823806980266354,0.859359395195979,0.901681047937578,
0.967654618228659),.UNSPECIFIED.);
#251=B_SPLINE_CURVE_WITH_KNOTS('',3,(#9623,#9624,#9625,#9626,#9627,#9628,
#9629,#9630,#9631,#9632,#9633,#9634,#9635,#9636,#9637,#9638,#9639,#9640,
#9641,#9642,#9643,#9644,#9645),.UNSPECIFIED.,.F.,.F.,(4,1,1,1,1,1,1,1,1,
1,1,1,1,1,1,1,1,1,1,1,4),(0.0323453817713401,0.0983189520624214,0.14064060480402,
0.176193019733645,0.208307484243854,0.23948443235858,0.271287112904486,
0.28220667781497,0.293329328714142,0.304676551002397,0.319437818234531,
0.350137192454192,0.38765864687273,0.432002181900136,0.483167797782405,
0.541155494678712,0.605965272697963,0.67759713191795,0.75605107239617,0.841327094176323,
1.),.UNSPECIFIED.);
#252=B_SPLINE_CURVE_WITH_KNOTS('',3,(#9649,#9650,#9651,#9652,#9653,#9654,
#9655,#9656,#9657,#9658,#9659,#9660,#9661,#9662,#9663,#9664,#9665,#9666,
#9667,#9668,#9669,#9670,#9671),.UNSPECIFIED.,.F.,.F.,(4,1,1,1,1,1,1,1,1,
1,1,1,1,1,1,1,1,1,1,1,4),(0.,0.158672905823676,0.243948927603829,0.322402868082049,
0.394034727302036,0.458844505321287,0.516832202217594,0.567997818099863,
0.612341353127269,0.649862807545807,0.680562181765468,0.695323448997602,
0.706670671285856,0.717793322185029,0.728712887095513,0.760515567641419,
0.791692515756145,0.823806980266354,0.859359395195979,0.901681047937578,
0.967654618228659),.UNSPECIFIED.);
#253=B_SPLINE_CURVE_WITH_KNOTS('',3,(#9675,#9676,#9677,#9678,#9679,#9680,
#9681,#9682,#9683,#9684,#9685,#9686,#9687,#9688,#9689,#9690,#9691,#9692,
#9693,#9694,#9695,#9696,#9697),.UNSPECIFIED.,.F.,.F.,(4,1,1,1,1,1,1,1,1,
1,1,1,1,1,1,1,1,1,1,1,4),(0.0323453817713401,0.0983189520624214,0.14064060480402,
0.176193019733645,0.208307484243854,0.23948443235858,0.271287112904486,
0.28220667781497,0.293329328714142,0.304676551002397,0.319437818234531,
0.350137192454192,0.38765864687273,0.432002181900136,0.483167797782405,
0.541155494678712,0.605965272697963,0.67759713191795,0.75605107239617,0.841327094176323,
1.),.UNSPECIFIED.);
#254=B_SPLINE_CURVE_WITH_KNOTS('',3,(#9701,#9702,#9703,#9704,#9705,#9706,
#9707,#9708,#9709,#9710,#9711,#9712,#9713,#9714,#9715,#9716,#9717,#9718,
#9719,#9720,#9721,#9722,#9723),.UNSPECIFIED.,.F.,.F.,(4,1,1,1,1,1,1,1,1,
1,1,1,1,1,1,1,1,1,1,1,4),(0.,0.158672905823676,0.243948927603829,0.322402868082049,
0.394034727302036,0.458844505321287,0.516832202217594,0.567997818099863,
0.612341353127269,0.649862807545807,0.680562181765468,0.695323448997602,
0.706670671285856,0.717793322185029,0.728712887095513,0.760515567641419,
0.791692515756145,0.823806980266354,0.859359395195979,0.901681047937578,
0.967654618228659),.UNSPECIFIED.);
#255=B_SPLINE_CURVE_WITH_KNOTS('',3,(#9727,#9728,#9729,#9730,#9731,#9732,
#9733,#9734,#9735,#9736,#9737,#9738,#9739,#9740,#9741,#9742,#9743,#9744,
#9745,#9746,#9747,#9748,#9749),.UNSPECIFIED.,.F.,.F.,(4,1,1,1,1,1,1,1,1,
1,1,1,1,1,1,1,1,1,1,1,4),(0.0323453817713401,0.0983189520624214,0.14064060480402,
0.176193019733645,0.208307484243854,0.23948443235858,0.271287112904486,
0.28220667781497,0.293329328714142,0.304676551002397,0.319437818234531,
0.350137192454192,0.38765864687273,0.432002181900136,0.483167797782405,
0.541155494678712,0.605965272697963,0.67759713191795,0.75605107239617,0.841327094176323,
1.),.UNSPECIFIED.);
#256=B_SPLINE_CURVE_WITH_KNOTS('',3,(#9753,#9754,#9755,#9756,#9757,#9758,
#9759,#9760,#9761,#9762,#9763,#9764,#9765,#9766,#9767,#9768,#9769,#9770,
#9771,#9772,#9773,#9774,#9775),.UNSPECIFIED.,.F.,.F.,(4,1,1,1,1,1,1,1,1,
1,1,1,1,1,1,1,1,1,1,1,4),(0.,0.158672905823676,0.243948927603829,0.322402868082049,
0.394034727302036,0.458844505321287,0.516832202217594,0.567997818099863,
0.612341353127269,0.649862807545807,0.680562181765468,0.695323448997602,
0.706670671285856,0.717793322185029,0.728712887095513,0.760515567641419,
0.791692515756145,0.823806980266354,0.859359395195979,0.901681047937578,
0.967654618228659),.UNSPECIFIED.);
#257=B_SPLINE_CURVE_WITH_KNOTS('',3,(#9779,#9780,#9781,#9782,#9783,#9784,
#9785,#9786,#9787,#9788,#9789,#9790,#9791,#9792,#9793,#9794,#9795,#9796,
#9797,#9798,#9799,#9800,#9801),.UNSPECIFIED.,.F.,.F.,(4,1,1,1,1,1,1,1,1,
1,1,1,1,1,1,1,1,1,1,1,4),(0.0323453817713401,0.0983189520624214,0.14064060480402,
0.176193019733645,0.208307484243854,0.23948443235858,0.271287112904486,
0.28220667781497,0.293329328714142,0.304676551002397,0.319437818234531,
0.350137192454192,0.38765864687273,0.432002181900136,0.483167797782405,
0.541155494678712,0.605965272697963,0.67759713191795,0.75605107239617,0.841327094176323,
1.),.UNSPECIFIED.);
#258=B_SPLINE_CURVE_WITH_KNOTS('',3,(#9805,#9806,#9807,#9808,#9809,#9810,
#9811,#9812,#9813,#9814,#9815,#9816,#9817,#9818,#9819,#9820,#9821,#9822,
#9823,#9824,#9825,#9826,#9827),.UNSPECIFIED.,.F.,.F.,(4,1,1,1,1,1,1,1,1,
1,1,1,1,1,1,1,1,1,1,1,4),(0.,0.158672905823676,0.243948927603829,0.322402868082049,
0.394034727302036,0.458844505321287,0.516832202217594,0.567997818099863,
0.612341353127269,0.649862807545807,0.680562181765468,0.695323448997602,
0.706670671285856,0.717793322185029,0.728712887095513,0.760515567641419,
0.791692515756145,0.823806980266354,0.859359395195979,0.901681047937578,
0.967654618228659),.UNSPECIFIED.);
#259=B_SPLINE_CURVE_WITH_KNOTS('',3,(#9831,#9832,#9833,#9834,#9835,#9836,
#9837,#9838,#9839,#9840,#9841,#9842,#9843,#9844,#9845,#9846,#9847,#9848,
#9849,#9850,#9851,#9852,#9853),.UNSPECIFIED.,.F.,.F.,(4,1,1,1,1,1,1,1,1,
1,1,1,1,1,1,1,1,1,1,1,4),(0.0323453817713401,0.0983189520624214,0.14064060480402,
0.176193019733645,0.208307484243854,0.23948443235858,0.271287112904486,
0.28220667781497,0.293329328714142,0.304676551002397,0.319437818234531,
0.350137192454192,0.38765864687273,0.432002181900136,0.483167797782405,
0.541155494678712,0.605965272697963,0.67759713191795,0.75605107239617,0.841327094176323,
1.),.UNSPECIFIED.);
#260=B_SPLINE_CURVE_WITH_KNOTS('',3,(#9857,#9858,#9859,#9860,#9861,#9862,
#9863,#9864,#9865,#9866,#9867,#9868,#9869,#9870,#9871,#9872,#9873,#9874,
#9875,#9876,#9877,#9878,#9879),.UNSPECIFIED.,.F.,.F.,(4,1,1,1,1,1,1,1,1,
1,1,1,1,1,1,1,1,1,1,1,4),(0.,0.158672905823676,0.243948927603829,0.322402868082049,
0.394034727302036,0.458844505321287,0.516832202217594,0.567997818099863,
0.612341353127269,0.649862807545807,0.680562181765468,0.695323448997602,
0.706670671285856,0.717793322185029,0.728712887095513,0.760515567641419,
0.791692515756145,0.823806980266354,0.859359395195979,0.901681047937578,
0.967654618228659),.UNSPECIFIED.);
#261=B_SPLINE_CURVE_WITH_KNOTS('',3,(#9883,#9884,#9885,#9886,#9887,#9888,
#9889,#9890,#9891,#9892,#9893,#9894,#9895,#9896,#9897,#9898,#9899,#9900,
#9901,#9902,#9903,#9904,#9905),.UNSPECIFIED.,.F.,.F.,(4,1,1,1,1,1,1,1,1,
1,1,1,1,1,1,1,1,1,1,1,4),(0.0323453817713401,0.0983189520624214,0.14064060480402,
0.176193019733645,0.208307484243854,0.23948443235858,0.271287112904486,
0.28220667781497,0.293329328714142,0.304676551002397,0.319437818234531,
0.350137192454192,0.38765864687273,0.432002181900136,0.483167797782405,
0.541155494678712,0.605965272697963,0.67759713191795,0.75605107239617,0.841327094176323,
1.),.UNSPECIFIED.);
#262=B_SPLINE_CURVE_WITH_KNOTS('',3,(#9909,#9910,#9911,#9912,#9913,#9914,
#9915,#9916,#9917,#9918,#9919,#9920,#9921,#9922,#9923,#9924,#9925,#9926,
#9927,#9928,#9929,#9930,#9931),.UNSPECIFIED.,.F.,.F.,(4,1,1,1,1,1,1,1,1,
1,1,1,1,1,1,1,1,1,1,1,4),(0.,0.158672905823676,0.243948927603829,0.322402868082049,
0.394034727302036,0.458844505321287,0.516832202217594,0.567997818099863,
0.612341353127269,0.649862807545807,0.680562181765468,0.695323448997602,
0.706670671285856,0.717793322185029,0.728712887095513,0.760515567641419,
0.791692515756145,0.823806980266354,0.859359395195979,0.901681047937578,
0.967654618228659),.UNSPECIFIED.);
#263=B_SPLINE_CURVE_WITH_KNOTS('',3,(#9935,#9936,#9937,#9938,#9939,#9940,
#9941,#9942,#9943,#9944,#9945,#9946,#9947,#9948,#9949,#9950,#9951,#9952,
#9953,#9954,#9955,#9956,#9957),.UNSPECIFIED.,.F.,.F.,(4,1,1,1,1,1,1,1,1,
1,1,1,1,1,1,1,1,1,1,1,4),(0.0323453817713401,0.0983189520624214,0.14064060480402,
0.176193019733645,0.208307484243854,0.23948443235858,0.271287112904486,
0.28220667781497,0.293329328714142,0.304676551002397,0.319437818234531,
0.350137192454192,0.38765864687273,0.432002181900136,0.483167797782405,
0.541155494678712,0.605965272697963,0.67759713191795,0.75605107239617,0.841327094176323,
1.),.UNSPECIFIED.);
#264=B_SPLINE_CURVE_WITH_KNOTS('',3,(#9961,#9962,#9963,#9964,#9965,#9966,
#9967,#9968,#9969,#9970,#9971,#9972,#9973,#9974,#9975,#9976,#9977,#9978,
#9979,#9980,#9981,#9982,#9983),.UNSPECIFIED.,.F.,.F.,(4,1,1,1,1,1,1,1,1,
1,1,1,1,1,1,1,1,1,1,1,4),(0.,0.158672905823676,0.243948927603829,0.322402868082049,
0.394034727302036,0.458844505321287,0.516832202217594,0.567997818099863,
0.612341353127269,0.649862807545807,0.680562181765468,0.695323448997602,
0.706670671285856,0.717793322185029,0.728712887095513,0.760515567641419,
0.791692515756145,0.823806980266354,0.859359395195979,0.901681047937578,
0.967654618228659),.UNSPECIFIED.);
#265=B_SPLINE_CURVE_WITH_KNOTS('',3,(#9987,#9988,#9989,#9990,#9991,#9992,
#9993,#9994,#9995,#9996,#9997,#9998,#9999,#10000,#10001,#10002,#10003,#10004,
#10005,#10006,#10007,#10008,#10009),.UNSPECIFIED.,.F.,.F.,(4,1,1,1,1,1,
1,1,1,1,1,1,1,1,1,1,1,1,1,1,4),(0.0323453817713401,0.0983189520624214,0.14064060480402,
0.176193019733645,0.208307484243854,0.23948443235858,0.271287112904486,
0.28220667781497,0.293329328714142,0.304676551002397,0.319437818234531,
0.350137192454192,0.38765864687273,0.432002181900136,0.483167797782405,
0.541155494678712,0.605965272697963,0.67759713191795,0.75605107239617,0.841327094176323,
1.),.UNSPECIFIED.);
#266=B_SPLINE_CURVE_WITH_KNOTS('',3,(#10013,#10014,#10015,#10016,#10017,
#10018,#10019,#10020,#10021,#10022,#10023,#10024,#10025,#10026,#10027,#10028,
#10029,#10030,#10031,#10032,#10033,#10034,#10035),.UNSPECIFIED.,.F.,.F.,
(4,1,1,1,1,1,1,1,1,1,1,1,1,1,1,1,1,1,1,1,4),(0.,0.158672905823676,0.243948927603829,
0.322402868082049,0.394034727302036,0.458844505321287,0.516832202217594,
0.567997818099863,0.612341353127269,0.649862807545807,0.680562181765468,
0.695323448997602,0.706670671285856,0.717793322185029,0.728712887095513,
0.760515567641419,0.791692515756145,0.823806980266354,0.859359395195979,
0.901681047937578,0.967654618228659),.UNSPECIFIED.);
#267=B_SPLINE_CURVE_WITH_KNOTS('',3,(#10039,#10040,#10041,#10042,#10043,
#10044,#10045,#10046,#10047,#10048,#10049,#10050,#10051,#10052,#10053,#10054,
#10055,#10056,#10057,#10058,#10059,#10060,#10061),.UNSPECIFIED.,.F.,.F.,
(4,1,1,1,1,1,1,1,1,1,1,1,1,1,1,1,1,1,1,1,4),(0.0323453817713401,0.0983189520624214,
0.14064060480402,0.176193019733645,0.208307484243854,0.23948443235858,0.271287112904486,
0.28220667781497,0.293329328714142,0.304676551002397,0.319437818234531,
0.350137192454192,0.38765864687273,0.432002181900136,0.483167797782405,
0.541155494678712,0.605965272697963,0.67759713191795,0.75605107239617,0.841327094176323,
1.),.UNSPECIFIED.);
#268=B_SPLINE_CURVE_WITH_KNOTS('',3,(#10065,#10066,#10067,#10068,#10069,
#10070,#10071,#10072,#10073,#10074,#10075,#10076,#10077,#10078,#10079,#10080,
#10081,#10082,#10083,#10084,#10085,#10086,#10087),.UNSPECIFIED.,.F.,.F.,
(4,1,1,1,1,1,1,1,1,1,1,1,1,1,1,1,1,1,1,1,4),(0.,0.158672905823676,0.243948927603829,
0.322402868082049,0.394034727302036,0.458844505321287,0.516832202217594,
0.567997818099863,0.612341353127269,0.649862807545807,0.680562181765468,
0.695323448997602,0.706670671285856,0.717793322185029,0.728712887095513,
0.760515567641419,0.791692515756145,0.823806980266354,0.859359395195979,
0.901681047937578,0.967654618228659),.UNSPECIFIED.);
#269=B_SPLINE_CURVE_WITH_KNOTS('',3,(#10090,#10091,#10092,#10093,#10094,
#10095,#10096,#10097,#10098,#10099,#10100,#10101,#10102,#10103,#10104,#10105,
#10106,#10107,#10108,#10109,#10110,#10111,#10112),.UNSPECIFIED.,.F.,.F.,
(4,1,1,1,1,1,1,1,1,1,1,1,1,1,1,1,1,1,1,1,4),(0.0323453817713401,0.0983189520624214,
0.14064060480402,0.176193019733645,0.208307484243854,0.23948443235858,0.271287112904486,
0.28220667781497,0.293329328714142,0.304676551002397,0.319437818234531,
0.350137192454192,0.38765864687273,0.432002181900136,0.483167797782405,
0.541155494678712,0.605965272697963,0.67759713191795,0.75605107239617,0.841327094176323,
1.),.UNSPECIFIED.);
#270=B_SPLINE_CURVE_WITH_KNOTS('',3,(#10114,#10115,#10116,#10117,#10118,
#10119,#10120,#10121,#10122,#10123,#10124,#10125,#10126,#10127,#10128,#10129,
#10130,#10131,#10132,#10133,#10134,#10135,#10136),.UNSPECIFIED.,.F.,.F.,
(4,1,1,1,1,1,1,1,1,1,1,1,1,1,1,1,1,1,1,1,4),(0.,0.158672905823676,0.243948927603829,
0.322402868082049,0.394034727302036,0.458844505321287,0.516832202217594,
0.567997818099863,0.612341353127269,0.649862807545807,0.680562181765468,
0.695323448997602,0.706670671285856,0.717793322185029,0.728712887095513,
0.760515567641419,0.791692515756145,0.823806980266354,0.859359395195979,
0.901681047937578,0.967654618228659),.UNSPECIFIED.);
#271=B_SPLINE_CURVE_WITH_KNOTS('',3,(#10140,#10141,#10142,#10143,#10144,
#10145,#10146,#10147,#10148,#10149,#10150,#10151,#10152,#10153,#10154,#10155,
#10156,#10157,#10158,#10159,#10160,#10161,#10162),.UNSPECIFIED.,.F.,.F.,
(4,1,1,1,1,1,1,1,1,1,1,1,1,1,1,1,1,1,1,1,4),(0.0323453817713401,0.0983189520624214,
0.14064060480402,0.176193019733645,0.208307484243854,0.23948443235858,0.271287112904486,
0.28220667781497,0.293329328714142,0.304676551002397,0.319437818234531,
0.350137192454192,0.38765864687273,0.432002181900136,0.483167797782405,
0.541155494678712,0.605965272697963,0.67759713191795,0.75605107239617,0.841327094176323,
1.),.UNSPECIFIED.);
#272=B_SPLINE_CURVE_WITH_KNOTS('',3,(#10166,#10167,#10168,#10169,#10170,
#10171,#10172,#10173,#10174,#10175,#10176,#10177,#10178,#10179,#10180,#10181,
#10182,#10183,#10184,#10185,#10186,#10187,#10188),.UNSPECIFIED.,.F.,.F.,
(4,1,1,1,1,1,1,1,1,1,1,1,1,1,1,1,1,1,1,1,4),(0.,0.158672905823676,0.243948927603829,
0.322402868082049,0.394034727302036,0.458844505321287,0.516832202217594,
0.567997818099863,0.612341353127269,0.649862807545807,0.680562181765468,
0.695323448997602,0.706670671285856,0.717793322185029,0.728712887095513,
0.760515567641419,0.791692515756145,0.823806980266354,0.859359395195979,
0.901681047937578,0.967654618228659),.UNSPECIFIED.);
#273=B_SPLINE_CURVE_WITH_KNOTS('',3,(#10192,#10193,#10194,#10195,#10196,
#10197,#10198,#10199,#10200,#10201,#10202,#10203,#10204,#10205,#10206,#10207,
#10208,#10209,#10210,#10211,#10212,#10213,#10214),.UNSPECIFIED.,.F.,.F.,
(4,1,1,1,1,1,1,1,1,1,1,1,1,1,1,1,1,1,1,1,4),(0.0323453817713401,0.0983189520624214,
0.14064060480402,0.176193019733645,0.208307484243854,0.23948443235858,0.271287112904486,
0.28220667781497,0.293329328714142,0.304676551002397,0.319437818234531,
0.350137192454192,0.38765864687273,0.432002181900136,0.483167797782405,
0.541155494678712,0.605965272697963,0.67759713191795,0.75605107239617,0.841327094176323,
1.),.UNSPECIFIED.);
#274=B_SPLINE_CURVE_WITH_KNOTS('',3,(#10218,#10219,#10220,#10221,#10222,
#10223,#10224,#10225,#10226,#10227,#10228,#10229,#10230,#10231,#10232,#10233,
#10234,#10235,#10236,#10237,#10238,#10239,#10240),.UNSPECIFIED.,.F.,.F.,
(4,1,1,1,1,1,1,1,1,1,1,1,1,1,1,1,1,1,1,1,4),(0.,0.158672905823676,0.243948927603829,
0.322402868082049,0.394034727302036,0.458844505321287,0.516832202217594,
0.567997818099863,0.612341353127269,0.649862807545807,0.680562181765468,
0.695323448997602,0.706670671285856,0.717793322185029,0.728712887095513,
0.760515567641419,0.791692515756145,0.823806980266354,0.859359395195979,
0.901681047937578,0.967654618228659),.UNSPECIFIED.);
#275=B_SPLINE_CURVE_WITH_KNOTS('',3,(#10244,#10245,#10246,#10247,#10248,
#10249,#10250,#10251,#10252,#10253,#10254,#10255,#10256,#10257,#10258,#10259,
#10260,#10261,#10262,#10263,#10264,#10265,#10266),.UNSPECIFIED.,.F.,.F.,
(4,1,1,1,1,1,1,1,1,1,1,1,1,1,1,1,1,1,1,1,4),(0.0323453817713401,0.0983189520624214,
0.14064060480402,0.176193019733645,0.208307484243854,0.23948443235858,0.271287112904486,
0.28220667781497,0.293329328714142,0.304676551002397,0.319437818234531,
0.350137192454192,0.38765864687273,0.432002181900136,0.483167797782405,
0.541155494678712,0.605965272697963,0.67759713191795,0.75605107239617,0.841327094176323,
1.),.UNSPECIFIED.);
#276=B_SPLINE_CURVE_WITH_KNOTS('',3,(#10270,#10271,#10272,#10273,#10274,
#10275,#10276,#10277,#10278,#10279,#10280,#10281,#10282,#10283,#10284,#10285,
#10286,#10287,#10288,#10289,#10290,#10291,#10292),.UNSPECIFIED.,.F.,.F.,
(4,1,1,1,1,1,1,1,1,1,1,1,1,1,1,1,1,1,1,1,4),(0.,0.158672905823676,0.243948927603829,
0.322402868082049,0.394034727302036,0.458844505321287,0.516832202217594,
0.567997818099863,0.612341353127269,0.649862807545807,0.680562181765468,
0.695323448997602,0.706670671285856,0.717793322185029,0.728712887095513,
0.760515567641419,0.791692515756145,0.823806980266354,0.859359395195979,
0.901681047937578,0.967654618228659),.UNSPECIFIED.);
#277=B_SPLINE_CURVE_WITH_KNOTS('',3,(#10296,#10297,#10298,#10299,#10300,
#10301,#10302,#10303,#10304,#10305,#10306,#10307,#10308,#10309,#10310,#10311,
#10312,#10313,#10314,#10315,#10316,#10317,#10318),.UNSPECIFIED.,.F.,.F.,
(4,1,1,1,1,1,1,1,1,1,1,1,1,1,1,1,1,1,1,1,4),(0.0323453817713401,0.0983189520624214,
0.14064060480402,0.176193019733645,0.208307484243854,0.23948443235858,0.271287112904486,
0.28220667781497,0.293329328714142,0.304676551002397,0.319437818234531,
0.350137192454192,0.38765864687273,0.432002181900136,0.483167797782405,
0.541155494678712,0.605965272697963,0.67759713191795,0.75605107239617,0.841327094176323,
1.),.UNSPECIFIED.);
#278=B_SPLINE_CURVE_WITH_KNOTS('',3,(#10322,#10323,#10324,#10325,#10326,
#10327,#10328,#10329,#10330,#10331,#10332,#10333,#10334,#10335,#10336,#10337,
#10338,#10339,#10340,#10341,#10342,#10343,#10344),.UNSPECIFIED.,.F.,.F.,
(4,1,1,1,1,1,1,1,1,1,1,1,1,1,1,1,1,1,1,1,4),(0.,0.158672905823676,0.243948927603829,
0.322402868082049,0.394034727302036,0.458844505321287,0.516832202217594,
0.567997818099863,0.612341353127269,0.649862807545807,0.680562181765468,
0.695323448997602,0.706670671285856,0.717793322185029,0.728712887095513,
0.760515567641419,0.791692515756145,0.823806980266354,0.859359395195979,
0.901681047937578,0.967654618228659),.UNSPECIFIED.);
#279=B_SPLINE_CURVE_WITH_KNOTS('',3,(#10348,#10349,#10350,#10351,#10352,
#10353,#10354,#10355,#10356,#10357,#10358,#10359,#10360,#10361,#10362,#10363,
#10364,#10365,#10366,#10367,#10368,#10369,#10370),.UNSPECIFIED.,.F.,.F.,
(4,1,1,1,1,1,1,1,1,1,1,1,1,1,1,1,1,1,1,1,4),(0.0323453817713401,0.0983189520624214,
0.14064060480402,0.176193019733645,0.208307484243854,0.23948443235858,0.271287112904486,
0.28220667781497,0.293329328714142,0.304676551002397,0.319437818234531,
0.350137192454192,0.38765864687273,0.432002181900136,0.483167797782405,
0.541155494678712,0.605965272697963,0.67759713191795,0.75605107239617,0.841327094176323,
1.),.UNSPECIFIED.);
#280=B_SPLINE_CURVE_WITH_KNOTS('',3,(#10374,#10375,#10376,#10377,#10378,
#10379,#10380,#10381,#10382,#10383,#10384,#10385,#10386,#10387,#10388,#10389,
#10390,#10391,#10392,#10393,#10394,#10395,#10396),.UNSPECIFIED.,.F.,.F.,
(4,1,1,1,1,1,1,1,1,1,1,1,1,1,1,1,1,1,1,1,4),(0.,0.158672905823676,0.243948927603829,
0.322402868082049,0.394034727302036,0.458844505321287,0.516832202217594,
0.567997818099863,0.612341353127269,0.649862807545807,0.680562181765468,
0.695323448997602,0.706670671285856,0.717793322185029,0.728712887095513,
0.760515567641419,0.791692515756145,0.823806980266354,0.859359395195979,
0.901681047937578,0.967654618228659),.UNSPECIFIED.);
#281=B_SPLINE_CURVE_WITH_KNOTS('',3,(#10400,#10401,#10402,#10403,#10404,
#10405,#10406,#10407,#10408,#10409,#10410,#10411,#10412,#10413,#10414,#10415,
#10416,#10417,#10418,#10419,#10420,#10421,#10422),.UNSPECIFIED.,.F.,.F.,
(4,1,1,1,1,1,1,1,1,1,1,1,1,1,1,1,1,1,1,1,4),(0.0323453817713401,0.0983189520624214,
0.14064060480402,0.176193019733645,0.208307484243854,0.23948443235858,0.271287112904486,
0.28220667781497,0.293329328714142,0.304676551002397,0.319437818234531,
0.350137192454192,0.38765864687273,0.432002181900136,0.483167797782405,
0.541155494678712,0.605965272697963,0.67759713191795,0.75605107239617,0.841327094176323,
1.),.UNSPECIFIED.);
#282=B_SPLINE_CURVE_WITH_KNOTS('',3,(#10426,#10427,#10428,#10429,#10430,
#10431,#10432,#10433,#10434,#10435,#10436,#10437,#10438,#10439,#10440,#10441,
#10442,#10443,#10444,#10445,#10446,#10447,#10448),.UNSPECIFIED.,.F.,.F.,
(4,1,1,1,1,1,1,1,1,1,1,1,1,1,1,1,1,1,1,1,4),(0.,0.158672905823676,0.243948927603829,
0.322402868082049,0.394034727302036,0.458844505321287,0.516832202217594,
0.567997818099863,0.612341353127269,0.649862807545807,0.680562181765468,
0.695323448997602,0.706670671285856,0.717793322185029,0.728712887095513,
0.760515567641419,0.791692515756145,0.823806980266354,0.859359395195979,
0.901681047937578,0.967654618228659),.UNSPECIFIED.);
#283=B_SPLINE_CURVE_WITH_KNOTS('',3,(#10452,#10453,#10454,#10455,#10456,
#10457,#10458,#10459,#10460,#10461,#10462,#10463,#10464,#10465,#10466,#10467,
#10468,#10469,#10470,#10471,#10472,#10473,#10474),.UNSPECIFIED.,.F.,.F.,
(4,1,1,1,1,1,1,1,1,1,1,1,1,1,1,1,1,1,1,1,4),(0.0323453817713401,0.0983189520624214,
0.14064060480402,0.176193019733645,0.208307484243854,0.23948443235858,0.271287112904486,
0.28220667781497,0.293329328714142,0.304676551002397,0.319437818234531,
0.350137192454192,0.38765864687273,0.432002181900136,0.483167797782405,
0.541155494678712,0.605965272697963,0.67759713191795,0.75605107239617,0.841327094176323,
1.),.UNSPECIFIED.);
#284=B_SPLINE_CURVE_WITH_KNOTS('',3,(#10478,#10479,#10480,#10481,#10482,
#10483,#10484,#10485,#10486,#10487,#10488,#10489,#10490,#10491,#10492,#10493,
#10494,#10495,#10496,#10497,#10498,#10499,#10500),.UNSPECIFIED.,.F.,.F.,
(4,1,1,1,1,1,1,1,1,1,1,1,1,1,1,1,1,1,1,1,4),(0.,0.158672905823676,0.243948927603829,
0.322402868082049,0.394034727302036,0.458844505321287,0.516832202217594,
0.567997818099863,0.612341353127269,0.649862807545807,0.680562181765468,
0.695323448997602,0.706670671285856,0.717793322185029,0.728712887095513,
0.760515567641419,0.791692515756145,0.823806980266354,0.859359395195979,
0.901681047937578,0.967654618228659),.UNSPECIFIED.);
#285=B_SPLINE_CURVE_WITH_KNOTS('',3,(#10504,#10505,#10506,#10507,#10508,
#10509,#10510,#10511,#10512,#10513,#10514,#10515,#10516,#10517,#10518,#10519,
#10520,#10521,#10522,#10523,#10524,#10525,#10526),.UNSPECIFIED.,.F.,.F.,
(4,1,1,1,1,1,1,1,1,1,1,1,1,1,1,1,1,1,1,1,4),(0.0323453817713401,0.0983189520624214,
0.14064060480402,0.176193019733645,0.208307484243854,0.23948443235858,0.271287112904486,
0.28220667781497,0.293329328714142,0.304676551002397,0.319437818234531,
0.350137192454192,0.38765864687273,0.432002181900136,0.483167797782405,
0.541155494678712,0.605965272697963,0.67759713191795,0.75605107239617,0.841327094176323,
1.),.UNSPECIFIED.);
#286=B_SPLINE_CURVE_WITH_KNOTS('',3,(#10530,#10531,#10532,#10533,#10534,
#10535,#10536,#10537,#10538,#10539,#10540,#10541,#10542,#10543,#10544,#10545,
#10546,#10547,#10548,#10549,#10550,#10551,#10552),.UNSPECIFIED.,.F.,.F.,
(4,1,1,1,1,1,1,1,1,1,1,1,1,1,1,1,1,1,1,1,4),(0.,0.158672905823676,0.243948927603829,
0.322402868082049,0.394034727302036,0.458844505321287,0.516832202217594,
0.567997818099863,0.612341353127269,0.649862807545807,0.680562181765468,
0.695323448997602,0.706670671285856,0.717793322185029,0.728712887095513,
0.760515567641419,0.791692515756145,0.823806980266354,0.859359395195979,
0.901681047937578,0.967654618228659),.UNSPECIFIED.);
#289=SHAPE_REPRESENTATION_RELATIONSHIP('SRR','None',#13027,#297);
#297=ADVANCED_BREP_SHAPE_REPRESENTATION('',(#321),#12960);
#309=STYLED_ITEM('',(#13076),#321);
#321=MANIFOLD_SOLID_BREP('Body1',#5584);
#367=FACE_BOUND('',#1036,.T.);
#368=FACE_BOUND('',#1038,.T.);
#369=FACE_BOUND('',#1040,.T.);
#370=FACE_BOUND('',#1042,.T.);
#371=FACE_BOUND('',#1123,.T.);
#372=FACE_BOUND('',#1125,.T.);
#480=PLANE('',#5903);
#481=PLANE('',#5904);
#482=PLANE('',#5905);
#483=PLANE('',#5945);
#484=PLANE('',#6024);
#485=PLANE('',#6025);
#678=FACE_OUTER_BOUND('',#1029,.T.);
#679=FACE_OUTER_BOUND('',#1030,.T.);
#680=FACE_OUTER_BOUND('',#1031,.T.);
#681=FACE_OUTER_BOUND('',#1032,.T.);
#682=FACE_OUTER_BOUND('',#1033,.T.);
#683=FACE_OUTER_BOUND('',#1034,.T.);
#684=FACE_OUTER_BOUND('',#1035,.T.);
#685=FACE_OUTER_BOUND('',#1037,.T.);
#686=FACE_OUTER_BOUND('',#1039,.T.);
#687=FACE_OUTER_BOUND('',#1041,.T.);
#688=FACE_OUTER_BOUND('',#1043,.T.);
#689=FACE_OUTER_BOUND('',#1044,.T.);
#690=FACE_OUTER_BOUND('',#1045,.T.);
#691=FACE_OUTER_BOUND('',#1046,.T.);
#692=FACE_OUTER_BOUND('',#1047,.T.);
#693=FACE_OUTER_BOUND('',#1048,.T.);
#694=FACE_OUTER_BOUND('',#1049,.T.);
#695=FACE_OUTER_BOUND('',#1050,.T.);
#696=FACE_OUTER_BOUND('',#1051,.T.);
#697=FACE_OUTER_BOUND('',#1052,.T.);
#698=FACE_OUTER_BOUND('',#1053,.T.);
#699=FACE_OUTER_BOUND('',#1054,.T.);
#700=FACE_OUTER_BOUND('',#1055,.T.);
#701=FACE_OUTER_BOUND('',#1056,.T.);
#702=FACE_OUTER_BOUND('',#1057,.T.);
#703=FACE_OUTER_BOUND('',#1058,.T.);
#704=FACE_OUTER_BOUND('',#1059,.T.);
#705=FACE_OUTER_BOUND('',#1060,.T.);
#706=FACE_OUTER_BOUND('',#1061,.T.);
#707=FACE_OUTER_BOUND('',#1062,.T.);
#708=FACE_OUTER_BOUND('',#1063,.T.);
#709=FACE_OUTER_BOUND('',#1064,.T.);
#710=FACE_OUTER_BOUND('',#1065,.T.);
#711=FACE_OUTER_BOUND('',#1066,.T.);
#712=FACE_OUTER_BOUND('',#1067,.T.);
#713=FACE_OUTER_BOUND('',#1068,.T.);
#714=FACE_OUTER_BOUND('',#1069,.T.);
#715=FACE_OUTER_BOUND('',#1070,.T.);
#716=FACE_OUTER_BOUND('',#1071,.T.);
#717=FACE_OUTER_BOUND('',#1072,.T.);
#718=FACE_OUTER_BOUND('',#1073,.T.);
#719=FACE_OUTER_BOUND('',#1074,.T.);
#720=FACE_OUTER_BOUND('',#1075,.T.);
#721=FACE_OUTER_BOUND('',#1076,.T.);
#722=FACE_OUTER_BOUND('',#1077,.T.);
#723=FACE_OUTER_BOUND('',#1078,.T.);
#724=FACE_OUTER_BOUND('',#1079,.T.);
#725=FACE_OUTER_BOUND('',#1080,.T.);
#726=FACE_OUTER_BOUND('',#1081,.T.);
#727=FACE_OUTER_BOUND('',#1082,.T.);
#728=FACE_OUTER_BOUND('',#1083,.T.);
#729=FACE_OUTER_BOUND('',#1084,.T.);
#730=FACE_OUTER_BOUND('',#1085,.T.);
#731=FACE_OUTER_BOUND('',#1086,.T.);
#732=FACE_OUTER_BOUND('',#1087,.T.);
#733=FACE_OUTER_BOUND('',#1088,.T.);
#734=FACE_OUTER_BOUND('',#1089,.T.);
#735=FACE_OUTER_BOUND('',#1090,.T.);
#736=FACE_OUTER_BOUND('',#1091,.T.);
#737=FACE_OUTER_BOUND('',#1092,.T.);
#738=FACE_OUTER_BOUND('',#1093,.T.);
#739=FACE_OUTER_BOUND('',#1094,.T.);
#740=FACE_OUTER_BOUND('',#1095,.T.);
#741=FACE_OUTER_BOUND('',#1096,.T.);
#742=FACE_OUTER_BOUND('',#1097,.T.);
#743=FACE_OUTER_BOUND('',#1098,.T.);
#744=FACE_OUTER_BOUND('',#1099,.T.);
#745=FACE_OUTER_BOUND('',#1100,.T.);
#746=FACE_OUTER_BOUND('',#1101,.T.);
#747=FACE_OUTER_BOUND('',#1102,.T.);
#748=FACE_OUTER_BOUND('',#1103,.T.);
#749=FACE_OUTER_BOUND('',#1104,.T.);
#750=FACE_OUTER_BOUND('',#1105,.T.);
#751=FACE_OUTER_BOUND('',#1106,.T.);
#752=FACE_OUTER_BOUND('',#1107,.T.);
#753=FACE_OUTER_BOUND('',#1108,.T.);
#754=FACE_OUTER_BOUND('',#1109,.T.);
#755=FACE_OUTER_BOUND('',#1110,.T.);
#756=FACE_OUTER_BOUND('',#1111,.T.);
#757=FACE_OUTER_BOUND('',#1112,.T.);
#758=FACE_OUTER_BOUND('',#1113,.T.);
#759=FACE_OUTER_BOUND('',#1114,.T.);
#760=FACE_OUTER_BOUND('',#1115,.T.);
#761=FACE_OUTER_BOUND('',#1116,.T.);
#762=FACE_OUTER_BOUND('',#1117,.T.);
#763=FACE_OUTER_BOUND('',#1118,.T.);
#764=FACE_OUTER_BOUND('',#1119,.T.);
#765=FACE_OUTER_BOUND('',#1120,.T.);
#766=FACE_OUTER_BOUND('',#1121,.T.);
#767=FACE_OUTER_BOUND('',#1122,.T.);
#768=FACE_OUTER_BOUND('',#1124,.T.);
#1029=EDGE_LOOP('',(#4291,#4292,#4293,#4294));
#1030=EDGE_LOOP('',(#4295,#4296,#4297,#4298));
#1031=EDGE_LOOP('',(#4299,#4300,#4301,#4302));
#1032=EDGE_LOOP('',(#4303,#4304,#4305,#4306));
#1033=EDGE_LOOP('',(#4307,#4308,#4309,#4310));
#1034=EDGE_LOOP('',(#4311,#4312,#4313,#4314));
#1035=EDGE_LOOP('',(#4315));
#1036=EDGE_LOOP('',(#4316));
#1037=EDGE_LOOP('',(#4317));
#1038=EDGE_LOOP('',(#4318));
#1039=EDGE_LOOP('',(#4319,#4320,#4321,#4322,#4323,#4324,#4325,#4326,#4327,
#4328,#4329,#4330,#4331,#4332,#4333,#4334,#4335,#4336,#4337,#4338,#4339,
#4340,#4341,#4342,#4343,#4344,#4345,#4346,#4347,#4348,#4349,#4350,#4351,
#4352,#4353,#4354,#4355,#4356,#4357,#4358,#4359,#4360,#4361,#4362,#4363,
#4364,#4365,#4366,#4367,#4368,#4369,#4370,#4371,#4372,#4373,#4374,#4375,
#4376,#4377,#4378,#4379,#4380,#4381,#4382,#4383,#4384,#4385,#4386,#4387,
#4388,#4389,#4390,#4391,#4392,#4393,#4394,#4395,#4396,#4397,#4398));
#1040=EDGE_LOOP('',(#4399));
#1041=EDGE_LOOP('',(#4400,#4401,#4402,#4403,#4404,#4405,#4406,#4407,#4408,
#4409,#4410,#4411,#4412,#4413,#4414,#4415,#4416,#4417,#4418,#4419,#4420,
#4421,#4422,#4423,#4424,#4425,#4426,#4427,#4428,#4429,#4430,#4431,#4432,
#4433,#4434,#4435,#4436,#4437,#4438,#4439,#4440,#4441,#4442,#4443,#4444,
#4445,#4446,#4447,#4448,#4449,#4450,#4451,#4452,#4453,#4454,#4455,#4456,
#4457,#4458,#4459,#4460,#4461,#4462,#4463,#4464,#4465,#4466,#4467,#4468,
#4469,#4470,#4471,#4472,#4473,#4474,#4475,#4476,#4477,#4478,#4479));
#1042=EDGE_LOOP('',(#4480));
#1043=EDGE_LOOP('',(#4481,#4482,#4483,#4484));
#1044=EDGE_LOOP('',(#4485,#4486,#4487,#4488));
#1045=EDGE_LOOP('',(#4489,#4490,#4491,#4492));
#1046=EDGE_LOOP('',(#4493,#4494,#4495,#4496));
#1047=EDGE_LOOP('',(#4497,#4498,#4499,#4500));
#1048=EDGE_LOOP('',(#4501,#4502,#4503,#4504));
#1049=EDGE_LOOP('',(#4505,#4506,#4507,#4508));
#1050=EDGE_LOOP('',(#4509,#4510,#4511,#4512));
#1051=EDGE_LOOP('',(#4513,#4514,#4515,#4516));
#1052=EDGE_LOOP('',(#4517,#4518,#4519,#4520));
#1053=EDGE_LOOP('',(#4521,#4522,#4523,#4524));
#1054=EDGE_LOOP('',(#4525,#4526,#4527,#4528));
#1055=EDGE_LOOP('',(#4529,#4530,#4531,#4532));
#1056=EDGE_LOOP('',(#4533,#4534,#4535,#4536));
#1057=EDGE_LOOP('',(#4537,#4538,#4539,#4540));
#1058=EDGE_LOOP('',(#4541,#4542,#4543,#4544));
#1059=EDGE_LOOP('',(#4545,#4546,#4547,#4548));
#1060=EDGE_LOOP('',(#4549,#4550,#4551,#4552));
#1061=EDGE_LOOP('',(#4553,#4554,#4555,#4556));
#1062=EDGE_LOOP('',(#4557,#4558,#4559,#4560));
#1063=EDGE_LOOP('',(#4561,#4562,#4563,#4564));
#1064=EDGE_LOOP('',(#4565,#4566,#4567,#4568));
#1065=EDGE_LOOP('',(#4569,#4570,#4571,#4572));
#1066=EDGE_LOOP('',(#4573,#4574,#4575,#4576));
#1067=EDGE_LOOP('',(#4577,#4578,#4579,#4580));
#1068=EDGE_LOOP('',(#4581,#4582,#4583,#4584));
#1069=EDGE_LOOP('',(#4585,#4586,#4587,#4588));
#1070=EDGE_LOOP('',(#4589,#4590,#4591,#4592));
#1071=EDGE_LOOP('',(#4593,#4594,#4595,#4596));
#1072=EDGE_LOOP('',(#4597,#4598,#4599,#4600));
#1073=EDGE_LOOP('',(#4601,#4602,#4603,#4604));
#1074=EDGE_LOOP('',(#4605,#4606,#4607,#4608));
#1075=EDGE_LOOP('',(#4609,#4610,#4611,#4612));
#1076=EDGE_LOOP('',(#4613,#4614,#4615,#4616));
#1077=EDGE_LOOP('',(#4617,#4618,#4619,#4620));
#1078=EDGE_LOOP('',(#4621,#4622,#4623,#4624));
#1079=EDGE_LOOP('',(#4625,#4626,#4627,#4628));
#1080=EDGE_LOOP('',(#4629,#4630,#4631,#4632));
#1081=EDGE_LOOP('',(#4633,#4634,#4635,#4636));
#1082=EDGE_LOOP('',(#4637,#4638,#4639,#4640));
#1083=EDGE_LOOP('',(#4641,#4642,#4643,#4644));
#1084=EDGE_LOOP('',(#4645,#4646,#4647,#4648));
#1085=EDGE_LOOP('',(#4649,#4650,#4651,#4652));
#1086=EDGE_LOOP('',(#4653,#4654,#4655,#4656));
#1087=EDGE_LOOP('',(#4657,#4658,#4659,#4660));
#1088=EDGE_LOOP('',(#4661,#4662,#4663,#4664));
#1089=EDGE_LOOP('',(#4665,#4666,#4667,#4668));
#1090=EDGE_LOOP('',(#4669,#4670,#4671,#4672));
#1091=EDGE_LOOP('',(#4673,#4674,#4675,#4676));
#1092=EDGE_LOOP('',(#4677,#4678,#4679,#4680));
#1093=EDGE_LOOP('',(#4681,#4682,#4683,#4684));
#1094=EDGE_LOOP('',(#4685,#4686,#4687,#4688));
#1095=EDGE_LOOP('',(#4689,#4690,#4691,#4692));
#1096=EDGE_LOOP('',(#4693,#4694,#4695,#4696));
#1097=EDGE_LOOP('',(#4697,#4698,#4699,#4700));
#1098=EDGE_LOOP('',(#4701,#4702,#4703,#4704));
#1099=EDGE_LOOP('',(#4705,#4706,#4707,#4708));
#1100=EDGE_LOOP('',(#4709,#4710,#4711,#4712));
#1101=EDGE_LOOP('',(#4713,#4714,#4715,#4716));
#1102=EDGE_LOOP('',(#4717,#4718,#4719,#4720));
#1103=EDGE_LOOP('',(#4721,#4722,#4723,#4724));
#1104=EDGE_LOOP('',(#4725,#4726,#4727,#4728));
#1105=EDGE_LOOP('',(#4729,#4730,#4731,#4732));
#1106=EDGE_LOOP('',(#4733,#4734,#4735,#4736));
#1107=EDGE_LOOP('',(#4737,#4738,#4739,#4740));
#1108=EDGE_LOOP('',(#4741,#4742,#4743,#4744));
#1109=EDGE_LOOP('',(#4745,#4746,#4747,#4748));
#1110=EDGE_LOOP('',(#4749,#4750,#4751,#4752));
#1111=EDGE_LOOP('',(#4753,#4754,#4755,#4756));
#1112=EDGE_LOOP('',(#4757,#4758,#4759,#4760));
#1113=EDGE_LOOP('',(#4761,#4762,#4763,#4764));
#1114=EDGE_LOOP('',(#4765,#4766,#4767,#4768));
#1115=EDGE_LOOP('',(#4769,#4770,#4771,#4772));
#1116=EDGE_LOOP('',(#4773,#4774,#4775,#4776));
#1117=EDGE_LOOP('',(#4777,#4778,#4779,#4780));
#1118=EDGE_LOOP('',(#4781,#4782,#4783,#4784));
#1119=EDGE_LOOP('',(#4785,#4786,#4787,#4788));
#1120=EDGE_LOOP('',(#4789,#4790,#4791,#4792));
#1121=EDGE_LOOP('',(#4793,#4794,#4795,#4796));
#1122=EDGE_LOOP('',(#4797));
#1123=EDGE_LOOP('',(#4798));
#1124=EDGE_LOOP('',(#4799));
#1125=EDGE_LOOP('',(#4800));
#1484=LINE('',#8441,#1941);
#1485=LINE('',#8447,#1942);
#1486=LINE('',#8453,#1943);
#1487=LINE('',#8459,#1944);
#1488=LINE('',#8465,#1945);
#1489=LINE('',#8472,#1946);
#1490=LINE('',#8475,#1947);
#1491=LINE('',#10600,#1948);
#1492=LINE('',#10601,#1949);
#1493=LINE('',#10603,#1950);
#1494=LINE('',#10650,#1951);
#1495=LINE('',#10652,#1952);
#1496=LINE('',#10699,#1953);
#1497=LINE('',#10701,#1954);
#1498=LINE('',#10748,#1955);
#1499=LINE('',#10750,#1956);
#1500=LINE('',#10797,#1957);
#1501=LINE('',#10799,#1958);
#1502=LINE('',#10846,#1959);
#1503=LINE('',#10848,#1960);
#1504=LINE('',#10895,#1961);
#1505=LINE('',#10897,#1962);
#1506=LINE('',#10944,#1963);
#1507=LINE('',#10946,#1964);
#1508=LINE('',#10993,#1965);
#1509=LINE('',#10995,#1966);
#1510=LINE('',#11042,#1967);
#1511=LINE('',#11044,#1968);
#1512=LINE('',#11091,#1969);
#1513=LINE('',#11093,#1970);
#1514=LINE('',#11140,#1971);
#1515=LINE('',#11142,#1972);
#1516=LINE('',#11189,#1973);
#1517=LINE('',#11191,#1974);
#1518=LINE('',#11238,#1975);
#1519=LINE('',#11240,#1976);
#1520=LINE('',#11287,#1977);
#1521=LINE('',#11289,#1978);
#1522=LINE('',#11336,#1979);
#1523=LINE('',#11338,#1980);
#1524=LINE('',#11385,#1981);
#1525=LINE('',#11387,#1982);
#1526=LINE('',#11480,#1983);
#1527=LINE('',#11482,#1984);
#1528=LINE('',#11529,#1985);
#1529=LINE('',#11531,#1986);
#1530=LINE('',#11578,#1987);
#1531=LINE('',#11580,#1988);
#1532=LINE('',#11627,#1989);
#1533=LINE('',#11629,#1990);
#1534=LINE('',#11676,#1991);
#1535=LINE('',#11678,#1992);
#1536=LINE('',#11725,#1993);
#1537=LINE('',#11727,#1994);
#1538=LINE('',#11774,#1995);
#1539=LINE('',#11776,#1996);
#1540=LINE('',#11823,#1997);
#1541=LINE('',#11825,#1998);
#1542=LINE('',#11872,#1999);
#1543=LINE('',#11874,#2000);
#1544=LINE('',#11921,#2001);
#1545=LINE('',#11923,#2002);
#1546=LINE('',#11970,#2003);
#1547=LINE('',#11972,#2004);
#1548=LINE('',#12019,#2005);
#1549=LINE('',#12021,#2006);
#1550=LINE('',#12068,#2007);
#1551=LINE('',#12070,#2008);
#1552=LINE('',#12117,#2009);
#1553=LINE('',#12119,#2010);
#1554=LINE('',#12166,#2011);
#1555=LINE('',#12168,#2012);
#1556=LINE('',#12215,#2013);
#1557=LINE('',#12217,#2014);
#1558=LINE('',#12264,#2015);
#1559=LINE('',#12266,#2016);
#1560=LINE('',#12313,#2017);
#1561=LINE('',#12315,#2018);
#1562=LINE('',#12362,#2019);
#1563=LINE('',#12364,#2020);
#1564=LINE('',#12411,#2021);
#1565=LINE('',#12413,#2022);
#1566=LINE('',#12460,#2023);
#1567=LINE('',#12462,#2024);
#1568=LINE('',#12509,#2025);
#1941=VECTOR('',#6888,7.);
#1942=VECTOR('',#6895,14.);
#1943=VECTOR('',#6902,7.);
#1944=VECTOR('',#6909,14.);
#1945=VECTOR('',#6916,2.5);
#1946=VECTOR('',#6923,1000.);
#1947=VECTOR('',#6926,1000.);
#1948=VECTOR('',#7091,1000.);
#1949=VECTOR('',#7092,1000.);
#1950=VECTOR('',#7095,1000.);
#1951=VECTOR('',#7096,1000.);
#1952=VECTOR('',#7099,1000.);
#1953=VECTOR('',#7100,1000.);
#1954=VECTOR('',#7103,1000.);
#1955=VECTOR('',#7104,1000.);
#1956=VECTOR('',#7107,1000.);
#1957=VECTOR('',#7108,1000.);
#1958=VECTOR('',#7111,1000.);
#1959=VECTOR('',#7112,1000.);
#1960=VECTOR('',#7115,1000.);
#1961=VECTOR('',#7116,1000.);
#1962=VECTOR('',#7119,1000.);
#1963=VECTOR('',#7120,1000.);
#1964=VECTOR('',#7123,1000.);
#1965=VECTOR('',#7124,1000.);
#1966=VECTOR('',#7127,1000.);
#1967=VECTOR('',#7128,1000.);
#1968=VECTOR('',#7131,1000.);
#1969=VECTOR('',#7132,1000.);
#1970=VECTOR('',#7135,1000.);
#1971=VECTOR('',#7136,1000.);
#1972=VECTOR('',#7139,1000.);
#1973=VECTOR('',#7140,1000.);
#1974=VECTOR('',#7143,1000.);
#1975=VECTOR('',#7144,1000.);
#1976=VECTOR('',#7147,1000.);
#1977=VECTOR('',#7148,1000.);
#1978=VECTOR('',#7151,1000.);
#1979=VECTOR('',#7152,1000.);
#1980=VECTOR('',#7155,1000.);
#1981=VECTOR('',#7156,1000.);
#1982=VECTOR('',#7159,1000.);
#1983=VECTOR('',#7160,1000.);
#1984=VECTOR('',#7163,1000.);
#1985=VECTOR('',#7164,1000.);
#1986=VECTOR('',#7167,1000.);
#1987=VECTOR('',#7168,1000.);
#1988=VECTOR('',#7171,1000.);
#1989=VECTOR('',#7172,1000.);
#1990=VECTOR('',#7175,1000.);
#1991=VECTOR('',#7176,1000.);
#1992=VECTOR('',#7179,1000.);
#1993=VECTOR('',#7180,1000.);
#1994=VECTOR('',#7183,1000.);
#1995=VECTOR('',#7184,1000.);
#1996=VECTOR('',#7187,1000.);
#1997=VECTOR('',#7188,1000.);
#1998=VECTOR('',#7191,1000.);
#1999=VECTOR('',#7192,1000.);
#2000=VECTOR('',#7195,1000.);
#2001=VECTOR('',#7196,1000.);
#2002=VECTOR('',#7199,1000.);
#2003=VECTOR('',#7200,1000.);
#2004=VECTOR('',#7203,1000.);
#2005=VECTOR('',#7204,1000.);
#2006=VECTOR('',#7207,1000.);
#2007=VECTOR('',#7208,1000.);
#2008=VECTOR('',#7211,1000.);
#2009=VECTOR('',#7212,1000.);
#2010=VECTOR('',#7215,1000.);
#2011=VECTOR('',#7216,1000.);
#2012=VECTOR('',#7219,1000.);
#2013=VECTOR('',#7220,1000.);
#2014=VECTOR('',#7223,1000.);
#2015=VECTOR('',#7224,1000.);
#2016=VECTOR('',#7227,1000.);
#2017=VECTOR('',#7228,1000.);
#2018=VECTOR('',#7231,1000.);
#2019=VECTOR('',#7232,1000.);
#2020=VECTOR('',#7235,1000.);
#2021=VECTOR('',#7236,1000.);
#2022=VECTOR('',#7239,1000.);
#2023=VECTOR('',#7240,1000.);
#2024=VECTOR('',#7243,1000.);
#2025=VECTOR('',#7244,1000.);
#2222=CIRCLE('',#5886,7.);
#2223=CIRCLE('',#5887,7.);
#2224=CIRCLE('',#5889,14.);
#2225=CIRCLE('',#5890,14.);
#2226=CIRCLE('',#5892,7.);
#2227=CIRCLE('',#5893,7.);
#2228=CIRCLE('',#5895,14.);
#2229=CIRCLE('',#5896,14.);
#2230=CIRCLE('',#5898,2.5);
#2231=CIRCLE('',#5899,2.5);
#2232=CIRCLE('',#5901,16.25);
#2233=CIRCLE('',#5902,16.25);
#2234=CIRCLE('',#5906,19.);
#2235=CIRCLE('',#5907,16.25);
#2236=CIRCLE('',#5908,19.);
#2237=CIRCLE('',#5909,16.25);
#2238=CIRCLE('',#5910,19.);
#2239=CIRCLE('',#5911,16.25);
#2240=CIRCLE('',#5912,19.);
#2241=CIRCLE('',#5913,16.25);
#2242=CIRCLE('',#5914,19.);
#2243=CIRCLE('',#5915,16.25);
#2244=CIRCLE('',#5916,19.);
#2245=CIRCLE('',#5917,16.25);
#2246=CIRCLE('',#5918,19.);
#2247=CIRCLE('',#5919,16.25);
#2248=CIRCLE('',#5920,19.);
#2249=CIRCLE('',#5921,16.25);
#2250=CIRCLE('',#5922,19.);
#2251=CIRCLE('',#5923,19.);
#2252=CIRCLE('',#5924,16.25);
#2253=CIRCLE('',#5925,19.);
#2254=CIRCLE('',#5926,16.25);
#2255=CIRCLE('',#5927,19.);
#2256=CIRCLE('',#5928,16.25);
#2257=CIRCLE('',#5929,19.);
#2258=CIRCLE('',#5930,16.25);
#2259=CIRCLE('',#5931,19.);
#2260=CIRCLE('',#5932,16.25);
#2261=CIRCLE('',#5933,19.);
#2262=CIRCLE('',#5934,16.25);
#2263=CIRCLE('',#5935,19.);
#2264=CIRCLE('',#5936,16.25);
#2265=CIRCLE('',#5937,19.);
#2266=CIRCLE('',#5938,16.25);
#2267=CIRCLE('',#5939,19.);
#2268=CIRCLE('',#5940,16.25);
#2269=CIRCLE('',#5941,19.);
#2270=CIRCLE('',#5942,16.25);
#2271=CIRCLE('',#5943,19.);
#2272=CIRCLE('',#5944,16.25);
#2273=CIRCLE('',#5946,16.25);
#2274=CIRCLE('',#5947,19.);
#2275=CIRCLE('',#5948,16.25);
#2276=CIRCLE('',#5949,19.);
#2277=CIRCLE('',#5950,16.25);
#2278=CIRCLE('',#5951,19.);
#2279=CIRCLE('',#5952,16.25);
#2280=CIRCLE('',#5953,19.);
#2281=CIRCLE('',#5954,16.25);
#2282=CIRCLE('',#5955,19.);
#2283=CIRCLE('',#5956,16.25);
#2284=CIRCLE('',#5957,19.);
#2285=CIRCLE('',#5958,16.25);
#2286=CIRCLE('',#5959,19.);
#2287=CIRCLE('',#5960,16.25);
#2288=CIRCLE('',#5961,19.);
#2289=CIRCLE('',#5962,16.25);
#2290=CIRCLE('',#5963,19.);
#2291=CIRCLE('',#5964,16.25);
#2292=CIRCLE('',#5965,19.);
#2293=CIRCLE('',#5966,16.25);
#2294=CIRCLE('',#5967,19.);
#2295=CIRCLE('',#5968,19.);
#2296=CIRCLE('',#5969,16.25);
#2297=CIRCLE('',#5970,19.);
#2298=CIRCLE('',#5971,16.25);
#2299=CIRCLE('',#5972,19.);
#2300=CIRCLE('',#5973,16.25);
#2301=CIRCLE('',#5974,19.);
#2302=CIRCLE('',#5975,16.25);
#2303=CIRCLE('',#5976,19.);
#2304=CIRCLE('',#5977,16.25);
#2305=CIRCLE('',#5978,19.);
#2306=CIRCLE('',#5979,16.25);
#2307=CIRCLE('',#5980,19.);
#2308=CIRCLE('',#5981,16.25);
#2309=CIRCLE('',#5982,19.);
#2310=CIRCLE('',#5983,16.25);
#2311=CIRCLE('',#5984,19.);
#2592=VERTEX_POINT('',#8438);
#2593=VERTEX_POINT('',#8440);
#2594=VERTEX_POINT('',#8444);
#2595=VERTEX_POINT('',#8446);
#2596=VERTEX_POINT('',#8450);
#2597=VERTEX_POINT('',#8452);
#2598=VERTEX_POINT('',#8456);
#2599=VERTEX_POINT('',#8458);
#2600=VERTEX_POINT('',#8462);
#2601=VERTEX_POINT('',#8464);
#2602=VERTEX_POINT('',#8468);
#2603=VERTEX_POINT('',#8469);
#2604=VERTEX_POINT('',#8471);
#2605=VERTEX_POINT('',#8473);
#2606=VERTEX_POINT('',#8479);
#2607=VERTEX_POINT('',#8480);
#2608=VERTEX_POINT('',#8504);
#2609=VERTEX_POINT('',#8506);
#2610=VERTEX_POINT('',#8530);
#2611=VERTEX_POINT('',#8532);
#2612=VERTEX_POINT('',#8556);
#2613=VERTEX_POINT('',#8558);
#2614=VERTEX_POINT('',#8582);
#2615=VERTEX_POINT('',#8584);
#2616=VERTEX_POINT('',#8608);
#2617=VERTEX_POINT('',#8610);
#2618=VERTEX_POINT('',#8634);
#2619=VERTEX_POINT('',#8636);
#2620=VERTEX_POINT('',#8660);
#2621=VERTEX_POINT('',#8662);
#2622=VERTEX_POINT('',#8686);
#2623=VERTEX_POINT('',#8688);
#2624=VERTEX_POINT('',#8712);
#2625=VERTEX_POINT('',#8714);
#2626=VERTEX_POINT('',#8738);
#2627=VERTEX_POINT('',#8740);
#2628=VERTEX_POINT('',#8764);
#2629=VERTEX_POINT('',#8766);
#2630=VERTEX_POINT('',#8790);
#2631=VERTEX_POINT('',#8792);
#2632=VERTEX_POINT('',#8816);
#2633=VERTEX_POINT('',#8818);
#2634=VERTEX_POINT('',#8842);
#2635=VERTEX_POINT('',#8844);
#2636=VERTEX_POINT('',#8868);
#2637=VERTEX_POINT('',#8870);
#2638=VERTEX_POINT('',#8894);
#2639=VERTEX_POINT('',#8896);
#2640=VERTEX_POINT('',#8920);
#2641=VERTEX_POINT('',#8945);
#2642=VERTEX_POINT('',#8969);
#2643=VERTEX_POINT('',#8971);
#2644=VERTEX_POINT('',#8995);
#2645=VERTEX_POINT('',#8997);
#2646=VERTEX_POINT('',#9021);
#2647=VERTEX_POINT('',#9023);
#2648=VERTEX_POINT('',#9047);
#2649=VERTEX_POINT('',#9049);
#2650=VERTEX_POINT('',#9073);
#2651=VERTEX_POINT('',#9075);
#2652=VERTEX_POINT('',#9099);
#2653=VERTEX_POINT('',#9101);
#2654=VERTEX_POINT('',#9125);
#2655=VERTEX_POINT('',#9127);
#2656=VERTEX_POINT('',#9151);
#2657=VERTEX_POINT('',#9153);
#2658=VERTEX_POINT('',#9177);
#2659=VERTEX_POINT('',#9179);
#2660=VERTEX_POINT('',#9203);
#2661=VERTEX_POINT('',#9205);
#2662=VERTEX_POINT('',#9229);
#2663=VERTEX_POINT('',#9231);
#2664=VERTEX_POINT('',#9255);
#2665=VERTEX_POINT('',#9257);
#2666=VERTEX_POINT('',#9281);
#2667=VERTEX_POINT('',#9283);
#2668=VERTEX_POINT('',#9307);
#2669=VERTEX_POINT('',#9309);
#2670=VERTEX_POINT('',#9333);
#2671=VERTEX_POINT('',#9335);
#2672=VERTEX_POINT('',#9359);
#2673=VERTEX_POINT('',#9361);
#2674=VERTEX_POINT('',#9385);
#2675=VERTEX_POINT('',#9387);
#2676=VERTEX_POINT('',#9411);
#2677=VERTEX_POINT('',#9413);
#2678=VERTEX_POINT('',#9437);
#2679=VERTEX_POINT('',#9439);
#2680=VERTEX_POINT('',#9463);
#2681=VERTEX_POINT('',#9465);
#2682=VERTEX_POINT('',#9489);
#2683=VERTEX_POINT('',#9491);
#2684=VERTEX_POINT('',#9517);
#2685=VERTEX_POINT('',#9518);
#2686=VERTEX_POINT('',#9542);
#2687=VERTEX_POINT('',#9544);
#2688=VERTEX_POINT('',#9568);
#2689=VERTEX_POINT('',#9570);
#2690=VERTEX_POINT('',#9594);
#2691=VERTEX_POINT('',#9596);
#2692=VERTEX_POINT('',#9620);
#2693=VERTEX_POINT('',#9622);
#2694=VERTEX_POINT('',#9646);
#2695=VERTEX_POINT('',#9648);
#2696=VERTEX_POINT('',#9672);
#2697=VERTEX_POINT('',#9674);
#2698=VERTEX_POINT('',#9698);
#2699=VERTEX_POINT('',#9700);
#2700=VERTEX_POINT('',#9724);
#2701=VERTEX_POINT('',#9726);
#2702=VERTEX_POINT('',#9750);
#2703=VERTEX_POINT('',#9752);
#2704=VERTEX_POINT('',#9776);
#2705=VERTEX_POINT('',#9778);
#2706=VERTEX_POINT('',#9802);
#2707=VERTEX_POINT('',#9804);
#2708=VERTEX_POINT('',#9828);
#2709=VERTEX_POINT('',#9830);
#2710=VERTEX_POINT('',#9854);
#2711=VERTEX_POINT('',#9856);
#2712=VERTEX_POINT('',#9880);
#2713=VERTEX_POINT('',#9882);
#2714=VERTEX_POINT('',#9906);
#2715=VERTEX_POINT('',#9908);
#2716=VERTEX_POINT('',#9932);
#2717=VERTEX_POINT('',#9934);
#2718=VERTEX_POINT('',#9958);
#2719=VERTEX_POINT('',#9960);
#2720=VERTEX_POINT('',#9984);
#2721=VERTEX_POINT('',#9986);
#2722=VERTEX_POINT('',#10010);
#2723=VERTEX_POINT('',#10012);
#2724=VERTEX_POINT('',#10036);
#2725=VERTEX_POINT('',#10038);
#2726=VERTEX_POINT('',#10062);
#2727=VERTEX_POINT('',#10064);
#2728=VERTEX_POINT('',#10088);
#2729=VERTEX_POINT('',#10113);
#2730=VERTEX_POINT('',#10137);
#2731=VERTEX_POINT('',#10139);
#2732=VERTEX_POINT('',#10163);
#2733=VERTEX_POINT('',#10165);
#2734=VERTEX_POINT('',#10189);
#2735=VERTEX_POINT('',#10191);
#2736=VERTEX_POINT('',#10215);
#2737=VERTEX_POINT('',#10217);
#2738=VERTEX_POINT('',#10241);
#2739=VERTEX_POINT('',#10243);
#2740=VERTEX_POINT('',#10267);
#2741=VERTEX_POINT('',#10269);
#2742=VERTEX_POINT('',#10293);
#2743=VERTEX_POINT('',#10295);
#2744=VERTEX_POINT('',#10319);
#2745=VERTEX_POINT('',#10321);
#2746=VERTEX_POINT('',#10345);
#2747=VERTEX_POINT('',#10347);
#2748=VERTEX_POINT('',#10371);
#2749=VERTEX_POINT('',#10373);
#2750=VERTEX_POINT('',#10397);
#2751=VERTEX_POINT('',#10399);
#2752=VERTEX_POINT('',#10423);
#2753=VERTEX_POINT('',#10425);
#2754=VERTEX_POINT('',#10449);
#2755=VERTEX_POINT('',#10451);
#2756=VERTEX_POINT('',#10475);
#2757=VERTEX_POINT('',#10477);
#2758=VERTEX_POINT('',#10501);
#2759=VERTEX_POINT('',#10503);
#2760=VERTEX_POINT('',#10527);
#2761=VERTEX_POINT('',#10529);
#3202=EDGE_CURVE('',#2592,#2592,#2222,.T.);
#3203=EDGE_CURVE('',#2592,#2593,#1484,.T.);
#3204=EDGE_CURVE('',#2593,#2593,#2223,.T.);
#3205=EDGE_CURVE('',#2594,#2594,#2224,.T.);
#3206=EDGE_CURVE('',#2594,#2595,#1485,.T.);
#3207=EDGE_CURVE('',#2595,#2595,#2225,.T.);
#3208=EDGE_CURVE('',#2596,#2596,#2226,.T.);
#3209=EDGE_CURVE('',#2596,#2597,#1486,.T.);
#3210=EDGE_CURVE('',#2597,#2597,#2227,.T.);
#3211=EDGE_CURVE('',#2598,#2598,#2228,.T.);
#3212=EDGE_CURVE('',#2598,#2599,#1487,.T.);
#3213=EDGE_CURVE('',#2599,#2599,#2229,.T.);
#3214=EDGE_CURVE('',#2600,#2600,#2230,.T.);
#3215=EDGE_CURVE('',#2600,#2601,#1488,.T.);
#3216=EDGE_CURVE('',#2601,#2601,#2231,.T.);
#3217=EDGE_CURVE('',#2602,#2603,#2232,.T.);
#3218=EDGE_CURVE('',#2602,#2604,#1489,.T.);
#3219=EDGE_CURVE('',#2604,#2605,#2233,.T.);
#3220=EDGE_CURVE('',#2603,#2605,#1490,.T.);
#3221=EDGE_CURVE('',#2606,#2607,#207,.T.);
#3222=EDGE_CURVE('',#2607,#2608,#2234,.T.);
#3223=EDGE_CURVE('',#2608,#2609,#208,.T.);
#3224=EDGE_CURVE('',#2609,#2610,#2235,.T.);
#3225=EDGE_CURVE('',#2610,#2611,#209,.T.);
#3226=EDGE_CURVE('',#2611,#2612,#2236,.T.);
#3227=EDGE_CURVE('',#2612,#2613,#210,.T.);
#3228=EDGE_CURVE('',#2613,#2614,#2237,.T.);
#3229=EDGE_CURVE('',#2614,#2615,#211,.T.);
#3230=EDGE_CURVE('',#2615,#2616,#2238,.T.);
#3231=EDGE_CURVE('',#2616,#2617,#212,.T.);
#3232=EDGE_CURVE('',#2617,#2618,#2239,.T.);
#3233=EDGE_CURVE('',#2618,#2619,#213,.T.);
#3234=EDGE_CURVE('',#2619,#2620,#2240,.T.);
#3235=EDGE_CURVE('',#2620,#2621,#214,.T.);
#3236=EDGE_CURVE('',#2621,#2622,#2241,.T.);
#3237=EDGE_CURVE('',#2622,#2623,#215,.T.);
#3238=EDGE_CURVE('',#2623,#2624,#2242,.T.);
#3239=EDGE_CURVE('',#2624,#2625,#216,.T.);
#3240=EDGE_CURVE('',#2625,#2626,#2243,.T.);
#3241=EDGE_CURVE('',#2626,#2627,#217,.T.);
#3242=EDGE_CURVE('',#2627,#2628,#2244,.T.);
#3243=EDGE_CURVE('',#2628,#2629,#218,.T.);
#3244=EDGE_CURVE('',#2629,#2630,#2245,.T.);
#3245=EDGE_CURVE('',#2630,#2631,#219,.T.);
#3246=EDGE_CURVE('',#2631,#2632,#2246,.T.);
#3247=EDGE_CURVE('',#2632,#2633,#220,.T.);
#3248=EDGE_CURVE('',#2633,#2634,#2247,.T.);
#3249=EDGE_CURVE('',#2634,#2635,#221,.T.);
#3250=EDGE_CURVE('',#2635,#2636,#2248,.T.);
#3251=EDGE_CURVE('',#2636,#2637,#222,.T.);
#3252=EDGE_CURVE('',#2637,#2638,#2249,.T.);
#3253=EDGE_CURVE('',#2638,#2639,#223,.T.);
#3254=EDGE_CURVE('',#2639,#2640,#2250,.T.);
#3255=EDGE_CURVE('',#2640,#2602,#224,.T.);
#3256=EDGE_CURVE('',#2603,#2641,#225,.T.);
#3257=EDGE_CURVE('',#2641,#2642,#2251,.T.);
#3258=EDGE_CURVE('',#2642,#2643,#226,.T.);
#3259=EDGE_CURVE('',#2643,#2644,#2252,.T.);
#3260=EDGE_CURVE('',#2644,#2645,#227,.T.);
#3261=EDGE_CURVE('',#2645,#2646,#2253,.T.);
#3262=EDGE_CURVE('',#2646,#2647,#228,.T.);
#3263=EDGE_CURVE('',#2647,#2648,#2254,.T.);
#3264=EDGE_CURVE('',#2648,#2649,#229,.T.);
#3265=EDGE_CURVE('',#2649,#2650,#2255,.T.);
#3266=EDGE_CURVE('',#2650,#2651,#230,.T.);
#3267=EDGE_CURVE('',#2651,#2652,#2256,.T.);
#3268=EDGE_CURVE('',#2652,#2653,#231,.T.);
#3269=EDGE_CURVE('',#2653,#2654,#2257,.T.);
#3270=EDGE_CURVE('',#2654,#2655,#232,.T.);
#3271=EDGE_CURVE('',#2655,#2656,#2258,.T.);
#3272=EDGE_CURVE('',#2656,#2657,#233,.T.);
#3273=EDGE_CURVE('',#2657,#2658,#2259,.T.);
#3274=EDGE_CURVE('',#2658,#2659,#234,.T.);
#3275=EDGE_CURVE('',#2659,#2660,#2260,.T.);
#3276=EDGE_CURVE('',#2660,#2661,#235,.T.);
#3277=EDGE_CURVE('',#2661,#2662,#2261,.T.);
#3278=EDGE_CURVE('',#2662,#2663,#236,.T.);
#3279=EDGE_CURVE('',#2663,#2664,#2262,.T.);
#3280=EDGE_CURVE('',#2664,#2665,#237,.T.);
#3281=EDGE_CURVE('',#2665,#2666,#2263,.T.);
#3282=EDGE_CURVE('',#2666,#2667,#238,.T.);
#3283=EDGE_CURVE('',#2667,#2668,#2264,.T.);
#3284=EDGE_CURVE('',#2668,#2669,#239,.T.);
#3285=EDGE_CURVE('',#2669,#2670,#2265,.T.);
#3286=EDGE_CURVE('',#2670,#2671,#240,.T.);
#3287=EDGE_CURVE('',#2671,#2672,#2266,.T.);
#3288=EDGE_CURVE('',#2672,#2673,#241,.T.);
#3289=EDGE_CURVE('',#2673,#2674,#2267,.T.);
#3290=EDGE_CURVE('',#2674,#2675,#242,.T.);
#3291=EDGE_CURVE('',#2675,#2676,#2268,.T.);
#3292=EDGE_CURVE('',#2676,#2677,#243,.T.);
#3293=EDGE_CURVE('',#2677,#2678,#2269,.T.);
#3294=EDGE_CURVE('',#2678,#2679,#244,.T.);
#3295=EDGE_CURVE('',#2679,#2680,#2270,.T.);
#3296=EDGE_CURVE('',#2680,#2681,#245,.T.);
#3297=EDGE_CURVE('',#2681,#2682,#2271,.T.);
#3298=EDGE_CURVE('',#2682,#2683,#246,.T.);
#3299=EDGE_CURVE('',#2683,#2606,#2272,.T.);
#3300=EDGE_CURVE('',#2684,#2685,#247,.T.);
#3301=EDGE_CURVE('',#2686,#2684,#2273,.T.);
#3302=EDGE_CURVE('',#2687,#2686,#248,.T.);
#3303=EDGE_CURVE('',#2688,#2687,#2274,.T.);
#3304=EDGE_CURVE('',#2689,#2688,#249,.T.);
#3305=EDGE_CURVE('',#2690,#2689,#2275,.T.);
#3306=EDGE_CURVE('',#2691,#2690,#250,.T.);
#3307=EDGE_CURVE('',#2692,#2691,#2276,.T.);
#3308=EDGE_CURVE('',#2693,#2692,#251,.T.);
#3309=EDGE_CURVE('',#2694,#2693,#2277,.T.);
#3310=EDGE_CURVE('',#2695,#2694,#252,.T.);
#3311=EDGE_CURVE('',#2696,#2695,#2278,.T.);
#3312=EDGE_CURVE('',#2697,#2696,#253,.T.);
#3313=EDGE_CURVE('',#2698,#2697,#2279,.T.);
#3314=EDGE_CURVE('',#2699,#2698,#254,.T.);
#3315=EDGE_CURVE('',#2700,#2699,#2280,.T.);
#3316=EDGE_CURVE('',#2701,#2700,#255,.T.);
#3317=EDGE_CURVE('',#2702,#2701,#2281,.T.);
#3318=EDGE_CURVE('',#2703,#2702,#256,.T.);
#3319=EDGE_CURVE('',#2704,#2703,#2282,.T.);
#3320=EDGE_CURVE('',#2705,#2704,#257,.T.);
#3321=EDGE_CURVE('',#2706,#2705,#2283,.T.);
#3322=EDGE_CURVE('',#2707,#2706,#258,.T.);
#3323=EDGE_CURVE('',#2708,#2707,#2284,.T.);
#3324=EDGE_CURVE('',#2709,#2708,#259,.T.);
#3325=EDGE_CURVE('',#2710,#2709,#2285,.T.);
#3326=EDGE_CURVE('',#2711,#2710,#260,.T.);
#3327=EDGE_CURVE('',#2712,#2711,#2286,.T.);
#3328=EDGE_CURVE('',#2713,#2712,#261,.T.);
#3329=EDGE_CURVE('',#2714,#2713,#2287,.T.);
#3330=EDGE_CURVE('',#2715,#2714,#262,.T.);
#3331=EDGE_CURVE('',#2716,#2715,#2288,.T.);
#3332=EDGE_CURVE('',#2717,#2716,#263,.T.);
#3333=EDGE_CURVE('',#2718,#2717,#2289,.T.);
#3334=EDGE_CURVE('',#2719,#2718,#264,.T.);
#3335=EDGE_CURVE('',#2720,#2719,#2290,.T.);
#3336=EDGE_CURVE('',#2721,#2720,#265,.T.);
#3337=EDGE_CURVE('',#2722,#2721,#2291,.T.);
#3338=EDGE_CURVE('',#2723,#2722,#266,.T.);
#3339=EDGE_CURVE('',#2724,#2723,#2292,.T.);
#3340=EDGE_CURVE('',#2725,#2724,#267,.T.);
#3341=EDGE_CURVE('',#2726,#2725,#2293,.T.);
#3342=EDGE_CURVE('',#2727,#2726,#268,.T.);
#3343=EDGE_CURVE('',#2728,#2727,#2294,.T.);
#3344=EDGE_CURVE('',#2605,#2728,#269,.T.);
#3345=EDGE_CURVE('',#2729,#2604,#270,.T.);
#3346=EDGE_CURVE('',#2730,#2729,#2295,.T.);
#3347=EDGE_CURVE('',#2731,#2730,#271,.T.);
#3348=EDGE_CURVE('',#2732,#2731,#2296,.T.);
#3349=EDGE_CURVE('',#2733,#2732,#272,.T.);
#3350=EDGE_CURVE('',#2734,#2733,#2297,.T.);
#3351=EDGE_CURVE('',#2735,#2734,#273,.T.);
#3352=EDGE_CURVE('',#2736,#2735,#2298,.T.);
#3353=EDGE_CURVE('',#2737,#2736,#274,.T.);
#3354=EDGE_CURVE('',#2738,#2737,#2299,.T.);
#3355=EDGE_CURVE('',#2739,#2738,#275,.T.);
#3356=EDGE_CURVE('',#2740,#2739,#2300,.T.);
#3357=EDGE_CURVE('',#2741,#2740,#276,.T.);
#3358=EDGE_CURVE('',#2742,#2741,#2301,.T.);
#3359=EDGE_CURVE('',#2743,#2742,#277,.T.);
#3360=EDGE_CURVE('',#2744,#2743,#2302,.T.);
#3361=EDGE_CURVE('',#2745,#2744,#278,.T.);
#3362=EDGE_CURVE('',#2746,#2745,#2303,.T.);
#3363=EDGE_CURVE('',#2747,#2746,#279,.T.);
#3364=EDGE_CURVE('',#2748,#2747,#2304,.T.);
#3365=EDGE_CURVE('',#2749,#2748,#280,.T.);
#3366=EDGE_CURVE('',#2750,#2749,#2305,.T.);
#3367=EDGE_CURVE('',#2751,#2750,#281,.T.);
#3368=EDGE_CURVE('',#2752,#2751,#2306,.T.);
#3369=EDGE_CURVE('',#2753,#2752,#282,.T.);
#3370=EDGE_CURVE('',#2754,#2753,#2307,.T.);
#3371=EDGE_CURVE('',#2755,#2754,#283,.T.);
#3372=EDGE_CURVE('',#2756,#2755,#2308,.T.);
#3373=EDGE_CURVE('',#2757,#2756,#284,.T.);
#3374=EDGE_CURVE('',#2758,#2757,#2309,.T.);
#3375=EDGE_CURVE('',#2759,#2758,#285,.T.);
#3376=EDGE_CURVE('',#2760,#2759,#2310,.T.);
#3377=EDGE_CURVE('',#2761,#2760,#286,.T.);
#3378=EDGE_CURVE('',#2685,#2761,#2311,.T.);
#3379=EDGE_CURVE('',#2607,#2685,#1491,.T.);
#3380=EDGE_CURVE('',#2606,#2684,#1492,.T.);
#3381=EDGE_CURVE('',#2608,#2761,#1493,.T.);
#3382=EDGE_CURVE('',#2609,#2760,#1494,.T.);
#3383=EDGE_CURVE('',#2610,#2759,#1495,.T.);
#3384=EDGE_CURVE('',#2611,#2758,#1496,.T.);
#3385=EDGE_CURVE('',#2612,#2757,#1497,.T.);
#3386=EDGE_CURVE('',#2613,#2756,#1498,.T.);
#3387=EDGE_CURVE('',#2614,#2755,#1499,.T.);
#3388=EDGE_CURVE('',#2615,#2754,#1500,.T.);
#3389=EDGE_CURVE('',#2616,#2753,#1501,.T.);
#3390=EDGE_CURVE('',#2617,#2752,#1502,.T.);
#3391=EDGE_CURVE('',#2618,#2751,#1503,.T.);
#3392=EDGE_CURVE('',#2619,#2750,#1504,.T.);
#3393=EDGE_CURVE('',#2620,#2749,#1505,.T.);
#3394=EDGE_CURVE('',#2621,#2748,#1506,.T.);
#3395=EDGE_CURVE('',#2622,#2747,#1507,.T.);
#3396=EDGE_CURVE('',#2623,#2746,#1508,.T.);
#3397=EDGE_CURVE('',#2624,#2745,#1509,.T.);
#3398=EDGE_CURVE('',#2625,#2744,#1510,.T.);
#3399=EDGE_CURVE('',#2626,#2743,#1511,.T.);
#3400=EDGE_CURVE('',#2627,#2742,#1512,.T.);
#3401=EDGE_CURVE('',#2628,#2741,#1513,.T.);
#3402=EDGE_CURVE('',#2629,#2740,#1514,.T.);
#3403=EDGE_CURVE('',#2630,#2739,#1515,.T.);
#3404=EDGE_CURVE('',#2631,#2738,#1516,.T.);
#3405=EDGE_CURVE('',#2632,#2737,#1517,.T.);
#3406=EDGE_CURVE('',#2633,#2736,#1518,.T.);
#3407=EDGE_CURVE('',#2634,#2735,#1519,.T.);
#3408=EDGE_CURVE('',#2635,#2734,#1520,.T.);
#3409=EDGE_CURVE('',#2636,#2733,#1521,.T.);
#3410=EDGE_CURVE('',#2637,#2732,#1522,.T.);
#3411=EDGE_CURVE('',#2638,#2731,#1523,.T.);
#3412=EDGE_CURVE('',#2639,#2730,#1524,.T.);
#3413=EDGE_CURVE('',#2640,#2729,#1525,.T.);
#3414=EDGE_CURVE('',#2641,#2728,#1526,.T.);
#3415=EDGE_CURVE('',#2642,#2727,#1527,.T.);
#3416=EDGE_CURVE('',#2643,#2726,#1528,.T.);
#3417=EDGE_CURVE('',#2644,#2725,#1529,.T.);
#3418=EDGE_CURVE('',#2645,#2724,#1530,.T.);
#3419=EDGE_CURVE('',#2646,#2723,#1531,.T.);
#3420=EDGE_CURVE('',#2647,#2722,#1532,.T.);
#3421=EDGE_CURVE('',#2648,#2721,#1533,.T.);
#3422=EDGE_CURVE('',#2649,#2720,#1534,.T.);
#3423=EDGE_CURVE('',#2650,#2719,#1535,.T.);
#3424=EDGE_CURVE('',#2651,#2718,#1536,.T.);
#3425=EDGE_CURVE('',#2652,#2717,#1537,.T.);
#3426=EDGE_CURVE('',#2653,#2716,#1538,.T.);
#3427=EDGE_CURVE('',#2654,#2715,#1539,.T.);
#3428=EDGE_CURVE('',#2655,#2714,#1540,.T.);
#3429=EDGE_CURVE('',#2656,#2713,#1541,.T.);
#3430=EDGE_CURVE('',#2657,#2712,#1542,.T.);
#3431=EDGE_CURVE('',#2658,#2711,#1543,.T.);
#3432=EDGE_CURVE('',#2659,#2710,#1544,.T.);
#3433=EDGE_CURVE('',#2660,#2709,#1545,.T.);
#3434=EDGE_CURVE('',#2661,#2708,#1546,.T.);
#3435=EDGE_CURVE('',#2662,#2707,#1547,.T.);
#3436=EDGE_CURVE('',#2663,#2706,#1548,.T.);
#3437=EDGE_CURVE('',#2664,#2705,#1549,.T.);
#3438=EDGE_CURVE('',#2665,#2704,#1550,.T.);
#3439=EDGE_CURVE('',#2666,#2703,#1551,.T.);
#3440=EDGE_CURVE('',#2667,#2702,#1552,.T.);
#3441=EDGE_CURVE('',#2668,#2701,#1553,.T.);
#3442=EDGE_CURVE('',#2669,#2700,#1554,.T.);
#3443=EDGE_CURVE('',#2670,#2699,#1555,.T.);
#3444=EDGE_CURVE('',#2671,#2698,#1556,.T.);
#3445=EDGE_CURVE('',#2672,#2697,#1557,.T.);
#3446=EDGE_CURVE('',#2673,#2696,#1558,.T.);
#3447=EDGE_CURVE('',#2674,#2695,#1559,.T.);
#3448=EDGE_CURVE('',#2675,#2694,#1560,.T.);
#3449=EDGE_CURVE('',#2676,#2693,#1561,.T.);
#3450=EDGE_CURVE('',#2677,#2692,#1562,.T.);
#3451=EDGE_CURVE('',#2678,#2691,#1563,.T.);
#3452=EDGE_CURVE('',#2679,#2690,#1564,.T.);
#3453=EDGE_CURVE('',#2680,#2689,#1565,.T.);
#3454=EDGE_CURVE('',#2681,#2688,#1566,.T.);
#3455=EDGE_CURVE('',#2682,#2687,#1567,.T.);
#3456=EDGE_CURVE('',#2683,#2686,#1568,.T.);
#4291=ORIENTED_EDGE('',*,*,#3202,.F.);
#4292=ORIENTED_EDGE('',*,*,#3203,.T.);
#4293=ORIENTED_EDGE('',*,*,#3204,.T.);
#4294=ORIENTED_EDGE('',*,*,#3203,.F.);
#4295=ORIENTED_EDGE('',*,*,#3205,.F.);
#4296=ORIENTED_EDGE('',*,*,#3206,.T.);
#4297=ORIENTED_EDGE('',*,*,#3207,.T.);
#4298=ORIENTED_EDGE('',*,*,#3206,.F.);
#4299=ORIENTED_EDGE('',*,*,#3208,.F.);
#4300=ORIENTED_EDGE('',*,*,#3209,.T.);
#4301=ORIENTED_EDGE('',*,*,#3210,.T.);
#4302=ORIENTED_EDGE('',*,*,#3209,.F.);
#4303=ORIENTED_EDGE('',*,*,#3211,.F.);
#4304=ORIENTED_EDGE('',*,*,#3212,.T.);
#4305=ORIENTED_EDGE('',*,*,#3213,.T.);
#4306=ORIENTED_EDGE('',*,*,#3212,.F.);
#4307=ORIENTED_EDGE('',*,*,#3214,.T.);
#4308=ORIENTED_EDGE('',*,*,#3215,.T.);
#4309=ORIENTED_EDGE('',*,*,#3216,.F.);
#4310=ORIENTED_EDGE('',*,*,#3215,.F.);
#4311=ORIENTED_EDGE('',*,*,#3217,.F.);
#4312=ORIENTED_EDGE('',*,*,#3218,.T.);
#4313=ORIENTED_EDGE('',*,*,#3219,.T.);
#4314=ORIENTED_EDGE('',*,*,#3220,.F.);
#4315=ORIENTED_EDGE('',*,*,#3202,.T.);
#4316=ORIENTED_EDGE('',*,*,#3216,.T.);
#4317=ORIENTED_EDGE('',*,*,#3208,.T.);
#4318=ORIENTED_EDGE('',*,*,#3214,.F.);
#4319=ORIENTED_EDGE('',*,*,#3221,.T.);
#4320=ORIENTED_EDGE('',*,*,#3222,.T.);
#4321=ORIENTED_EDGE('',*,*,#3223,.T.);
#4322=ORIENTED_EDGE('',*,*,#3224,.T.);
#4323=ORIENTED_EDGE('',*,*,#3225,.T.);
#4324=ORIENTED_EDGE('',*,*,#3226,.T.);
#4325=ORIENTED_EDGE('',*,*,#3227,.T.);
#4326=ORIENTED_EDGE('',*,*,#3228,.T.);
#4327=ORIENTED_EDGE('',*,*,#3229,.T.);
#4328=ORIENTED_EDGE('',*,*,#3230,.T.);
#4329=ORIENTED_EDGE('',*,*,#3231,.T.);
#4330=ORIENTED_EDGE('',*,*,#3232,.T.);
#4331=ORIENTED_EDGE('',*,*,#3233,.T.);
#4332=ORIENTED_EDGE('',*,*,#3234,.T.);
#4333=ORIENTED_EDGE('',*,*,#3235,.T.);
#4334=ORIENTED_EDGE('',*,*,#3236,.T.);
#4335=ORIENTED_EDGE('',*,*,#3237,.T.);
#4336=ORIENTED_EDGE('',*,*,#3238,.T.);
#4337=ORIENTED_EDGE('',*,*,#3239,.T.);
#4338=ORIENTED_EDGE('',*,*,#3240,.T.);
#4339=ORIENTED_EDGE('',*,*,#3241,.T.);
#4340=ORIENTED_EDGE('',*,*,#3242,.T.);
#4341=ORIENTED_EDGE('',*,*,#3243,.T.);
#4342=ORIENTED_EDGE('',*,*,#3244,.T.);
#4343=ORIENTED_EDGE('',*,*,#3245,.T.);
#4344=ORIENTED_EDGE('',*,*,#3246,.T.);
#4345=ORIENTED_EDGE('',*,*,#3247,.T.);
#4346=ORIENTED_EDGE('',*,*,#3248,.T.);
#4347=ORIENTED_EDGE('',*,*,#3249,.T.);
#4348=ORIENTED_EDGE('',*,*,#3250,.T.);
#4349=ORIENTED_EDGE('',*,*,#3251,.T.);
#4350=ORIENTED_EDGE('',*,*,#3252,.T.);
#4351=ORIENTED_EDGE('',*,*,#3253,.T.);
#4352=ORIENTED_EDGE('',*,*,#3254,.T.);
#4353=ORIENTED_EDGE('',*,*,#3255,.T.);
#4354=ORIENTED_EDGE('',*,*,#3217,.T.);
#4355=ORIENTED_EDGE('',*,*,#3256,.T.);
#4356=ORIENTED_EDGE('',*,*,#3257,.T.);
#4357=ORIENTED_EDGE('',*,*,#3258,.T.);
#4358=ORIENTED_EDGE('',*,*,#3259,.T.);
#4359=ORIENTED_EDGE('',*,*,#3260,.T.);
#4360=ORIENTED_EDGE('',*,*,#3261,.T.);
#4361=ORIENTED_EDGE('',*,*,#3262,.T.);
#4362=ORIENTED_EDGE('',*,*,#3263,.T.);
#4363=ORIENTED_EDGE('',*,*,#3264,.T.);
#4364=ORIENTED_EDGE('',*,*,#3265,.T.);
#4365=ORIENTED_EDGE('',*,*,#3266,.T.);
#4366=ORIENTED_EDGE('',*,*,#3267,.T.);
#4367=ORIENTED_EDGE('',*,*,#3268,.T.);
#4368=ORIENTED_EDGE('',*,*,#3269,.T.);
#4369=ORIENTED_EDGE('',*,*,#3270,.T.);
#4370=ORIENTED_EDGE('',*,*,#3271,.T.);
#4371=ORIENTED_EDGE('',*,*,#3272,.T.);
#4372=ORIENTED_EDGE('',*,*,#3273,.T.);
#4373=ORIENTED_EDGE('',*,*,#3274,.T.);
#4374=ORIENTED_EDGE('',*,*,#3275,.T.);
#4375=ORIENTED_EDGE('',*,*,#3276,.T.);
#4376=ORIENTED_EDGE('',*,*,#3277,.T.);
#4377=ORIENTED_EDGE('',*,*,#3278,.T.);
#4378=ORIENTED_EDGE('',*,*,#3279,.T.);
#4379=ORIENTED_EDGE('',*,*,#3280,.T.);
#4380=ORIENTED_EDGE('',*,*,#3281,.T.);
#4381=ORIENTED_EDGE('',*,*,#3282,.T.);
#4382=ORIENTED_EDGE('',*,*,#3283,.T.);
#4383=ORIENTED_EDGE('',*,*,#3284,.T.);
#4384=ORIENTED_EDGE('',*,*,#3285,.T.);
#4385=ORIENTED_EDGE('',*,*,#3286,.T.);
#4386=ORIENTED_EDGE('',*,*,#3287,.T.);
#4387=ORIENTED_EDGE('',*,*,#3288,.T.);
#4388=ORIENTED_EDGE('',*,*,#3289,.T.);
#4389=ORIENTED_EDGE('',*,*,#3290,.T.);
#4390=ORIENTED_EDGE('',*,*,#3291,.T.);
#4391=ORIENTED_EDGE('',*,*,#3292,.T.);
#4392=ORIENTED_EDGE('',*,*,#3293,.T.);
#4393=ORIENTED_EDGE('',*,*,#3294,.T.);
#4394=ORIENTED_EDGE('',*,*,#3295,.T.);
#4395=ORIENTED_EDGE('',*,*,#3296,.T.);
#4396=ORIENTED_EDGE('',*,*,#3297,.T.);
#4397=ORIENTED_EDGE('',*,*,#3298,.T.);
#4398=ORIENTED_EDGE('',*,*,#3299,.T.);
#4399=ORIENTED_EDGE('',*,*,#3213,.F.);
#4400=ORIENTED_EDGE('',*,*,#3300,.F.);
#4401=ORIENTED_EDGE('',*,*,#3301,.F.);
#4402=ORIENTED_EDGE('',*,*,#3302,.F.);
#4403=ORIENTED_EDGE('',*,*,#3303,.F.);
#4404=ORIENTED_EDGE('',*,*,#3304,.F.);
#4405=ORIENTED_EDGE('',*,*,#3305,.F.);
#4406=ORIENTED_EDGE('',*,*,#3306,.F.);
#4407=ORIENTED_EDGE('',*,*,#3307,.F.);
#4408=ORIENTED_EDGE('',*,*,#3308,.F.);
#4409=ORIENTED_EDGE('',*,*,#3309,.F.);
#4410=ORIENTED_EDGE('',*,*,#3310,.F.);
#4411=ORIENTED_EDGE('',*,*,#3311,.F.);
#4412=ORIENTED_EDGE('',*,*,#3312,.F.);
#4413=ORIENTED_EDGE('',*,*,#3313,.F.);
#4414=ORIENTED_EDGE('',*,*,#3314,.F.);
#4415=ORIENTED_EDGE('',*,*,#3315,.F.);
#4416=ORIENTED_EDGE('',*,*,#3316,.F.);
#4417=ORIENTED_EDGE('',*,*,#3317,.F.);
#4418=ORIENTED_EDGE('',*,*,#3318,.F.);
#4419=ORIENTED_EDGE('',*,*,#3319,.F.);
#4420=ORIENTED_EDGE('',*,*,#3320,.F.);
#4421=ORIENTED_EDGE('',*,*,#3321,.F.);
#4422=ORIENTED_EDGE('',*,*,#3322,.F.);
#4423=ORIENTED_EDGE('',*,*,#3323,.F.);
#4424=ORIENTED_EDGE('',*,*,#3324,.F.);
#4425=ORIENTED_EDGE('',*,*,#3325,.F.);
#4426=ORIENTED_EDGE('',*,*,#3326,.F.);
#4427=ORIENTED_EDGE('',*,*,#3327,.F.);
#4428=ORIENTED_EDGE('',*,*,#3328,.F.);
#4429=ORIENTED_EDGE('',*,*,#3329,.F.);
#4430=ORIENTED_EDGE('',*,*,#3330,.F.);
#4431=ORIENTED_EDGE('',*,*,#3331,.F.);
#4432=ORIENTED_EDGE('',*,*,#3332,.F.);
#4433=ORIENTED_EDGE('',*,*,#3333,.F.);
#4434=ORIENTED_EDGE('',*,*,#3334,.F.);
#4435=ORIENTED_EDGE('',*,*,#3335,.F.);
#4436=ORIENTED_EDGE('',*,*,#3336,.F.);
#4437=ORIENTED_EDGE('',*,*,#3337,.F.);
#4438=ORIENTED_EDGE('',*,*,#3338,.F.);
#4439=ORIENTED_EDGE('',*,*,#3339,.F.);
#4440=ORIENTED_EDGE('',*,*,#3340,.F.);
#4441=ORIENTED_EDGE('',*,*,#3341,.F.);
#4442=ORIENTED_EDGE('',*,*,#3342,.F.);
#4443=ORIENTED_EDGE('',*,*,#3343,.F.);
#4444=ORIENTED_EDGE('',*,*,#3344,.F.);
#4445=ORIENTED_EDGE('',*,*,#3219,.F.);
#4446=ORIENTED_EDGE('',*,*,#3345,.F.);
#4447=ORIENTED_EDGE('',*,*,#3346,.F.);
#4448=ORIENTED_EDGE('',*,*,#3347,.F.);
#4449=ORIENTED_EDGE('',*,*,#3348,.F.);
#4450=ORIENTED_EDGE('',*,*,#3349,.F.);
#4451=ORIENTED_EDGE('',*,*,#3350,.F.);
#4452=ORIENTED_EDGE('',*,*,#3351,.F.);
#4453=ORIENTED_EDGE('',*,*,#3352,.F.);
#4454=ORIENTED_EDGE('',*,*,#3353,.F.);
#4455=ORIENTED_EDGE('',*,*,#3354,.F.);
#4456=ORIENTED_EDGE('',*,*,#3355,.F.);
#4457=ORIENTED_EDGE('',*,*,#3356,.F.);
#4458=ORIENTED_EDGE('',*,*,#3357,.F.);
#4459=ORIENTED_EDGE('',*,*,#3358,.F.);
#4460=ORIENTED_EDGE('',*,*,#3359,.F.);
#4461=ORIENTED_EDGE('',*,*,#3360,.F.);
#4462=ORIENTED_EDGE('',*,*,#3361,.F.);
#4463=ORIENTED_EDGE('',*,*,#3362,.F.);
#4464=ORIENTED_EDGE('',*,*,#3363,.F.);
#4465=ORIENTED_EDGE('',*,*,#3364,.F.);
#4466=ORIENTED_EDGE('',*,*,#3365,.F.);
#4467=ORIENTED_EDGE('',*,*,#3366,.F.);
#4468=ORIENTED_EDGE('',*,*,#3367,.F.);
#4469=ORIENTED_EDGE('',*,*,#3368,.F.);
#4470=ORIENTED_EDGE('',*,*,#3369,.F.);
#4471=ORIENTED_EDGE('',*,*,#3370,.F.);
#4472=ORIENTED_EDGE('',*,*,#3371,.F.);
#4473=ORIENTED_EDGE('',*,*,#3372,.F.);
#4474=ORIENTED_EDGE('',*,*,#3373,.F.);
#4475=ORIENTED_EDGE('',*,*,#3374,.F.);
#4476=ORIENTED_EDGE('',*,*,#3375,.F.);
#4477=ORIENTED_EDGE('',*,*,#3376,.F.);
#4478=ORIENTED_EDGE('',*,*,#3377,.F.);
#4479=ORIENTED_EDGE('',*,*,#3378,.F.);
#4480=ORIENTED_EDGE('',*,*,#3207,.F.);
#4481=ORIENTED_EDGE('',*,*,#3300,.T.);
#4482=ORIENTED_EDGE('',*,*,#3379,.F.);
#4483=ORIENTED_EDGE('',*,*,#3221,.F.);
#4484=ORIENTED_EDGE('',*,*,#3380,.T.);
#4485=ORIENTED_EDGE('',*,*,#3378,.T.);
#4486=ORIENTED_EDGE('',*,*,#3381,.F.);
#4487=ORIENTED_EDGE('',*,*,#3222,.F.);
#4488=ORIENTED_EDGE('',*,*,#3379,.T.);
#4489=ORIENTED_EDGE('',*,*,#3377,.T.);
#4490=ORIENTED_EDGE('',*,*,#3382,.F.);
#4491=ORIENTED_EDGE('',*,*,#3223,.F.);
#4492=ORIENTED_EDGE('',*,*,#3381,.T.);
#4493=ORIENTED_EDGE('',*,*,#3376,.T.);
#4494=ORIENTED_EDGE('',*,*,#3383,.F.);
#4495=ORIENTED_EDGE('',*,*,#3224,.F.);
#4496=ORIENTED_EDGE('',*,*,#3382,.T.);
#4497=ORIENTED_EDGE('',*,*,#3375,.T.);
#4498=ORIENTED_EDGE('',*,*,#3384,.F.);
#4499=ORIENTED_EDGE('',*,*,#3225,.F.);
#4500=ORIENTED_EDGE('',*,*,#3383,.T.);
#4501=ORIENTED_EDGE('',*,*,#3374,.T.);
#4502=ORIENTED_EDGE('',*,*,#3385,.F.);
#4503=ORIENTED_EDGE('',*,*,#3226,.F.);
#4504=ORIENTED_EDGE('',*,*,#3384,.T.);
#4505=ORIENTED_EDGE('',*,*,#3373,.T.);
#4506=ORIENTED_EDGE('',*,*,#3386,.F.);
#4507=ORIENTED_EDGE('',*,*,#3227,.F.);
#4508=ORIENTED_EDGE('',*,*,#3385,.T.);
#4509=ORIENTED_EDGE('',*,*,#3372,.T.);
#4510=ORIENTED_EDGE('',*,*,#3387,.F.);
#4511=ORIENTED_EDGE('',*,*,#3228,.F.);
#4512=ORIENTED_EDGE('',*,*,#3386,.T.);
#4513=ORIENTED_EDGE('',*,*,#3371,.T.);
#4514=ORIENTED_EDGE('',*,*,#3388,.F.);
#4515=ORIENTED_EDGE('',*,*,#3229,.F.);
#4516=ORIENTED_EDGE('',*,*,#3387,.T.);
#4517=ORIENTED_EDGE('',*,*,#3370,.T.);
#4518=ORIENTED_EDGE('',*,*,#3389,.F.);
#4519=ORIENTED_EDGE('',*,*,#3230,.F.);
#4520=ORIENTED_EDGE('',*,*,#3388,.T.);
#4521=ORIENTED_EDGE('',*,*,#3369,.T.);
#4522=ORIENTED_EDGE('',*,*,#3390,.F.);
#4523=ORIENTED_EDGE('',*,*,#3231,.F.);
#4524=ORIENTED_EDGE('',*,*,#3389,.T.);
#4525=ORIENTED_EDGE('',*,*,#3368,.T.);
#4526=ORIENTED_EDGE('',*,*,#3391,.F.);
#4527=ORIENTED_EDGE('',*,*,#3232,.F.);
#4528=ORIENTED_EDGE('',*,*,#3390,.T.);
#4529=ORIENTED_EDGE('',*,*,#3367,.T.);
#4530=ORIENTED_EDGE('',*,*,#3392,.F.);
#4531=ORIENTED_EDGE('',*,*,#3233,.F.);
#4532=ORIENTED_EDGE('',*,*,#3391,.T.);
#4533=ORIENTED_EDGE('',*,*,#3366,.T.);
#4534=ORIENTED_EDGE('',*,*,#3393,.F.);
#4535=ORIENTED_EDGE('',*,*,#3234,.F.);
#4536=ORIENTED_EDGE('',*,*,#3392,.T.);
#4537=ORIENTED_EDGE('',*,*,#3365,.T.);
#4538=ORIENTED_EDGE('',*,*,#3394,.F.);
#4539=ORIENTED_EDGE('',*,*,#3235,.F.);
#4540=ORIENTED_EDGE('',*,*,#3393,.T.);
#4541=ORIENTED_EDGE('',*,*,#3364,.T.);
#4542=ORIENTED_EDGE('',*,*,#3395,.F.);
#4543=ORIENTED_EDGE('',*,*,#3236,.F.);
#4544=ORIENTED_EDGE('',*,*,#3394,.T.);
#4545=ORIENTED_EDGE('',*,*,#3363,.T.);
#4546=ORIENTED_EDGE('',*,*,#3396,.F.);
#4547=ORIENTED_EDGE('',*,*,#3237,.F.);
#4548=ORIENTED_EDGE('',*,*,#3395,.T.);
#4549=ORIENTED_EDGE('',*,*,#3362,.T.);
#4550=ORIENTED_EDGE('',*,*,#3397,.F.);
#4551=ORIENTED_EDGE('',*,*,#3238,.F.);
#4552=ORIENTED_EDGE('',*,*,#3396,.T.);
#4553=ORIENTED_EDGE('',*,*,#3361,.T.);
#4554=ORIENTED_EDGE('',*,*,#3398,.F.);
#4555=ORIENTED_EDGE('',*,*,#3239,.F.);
#4556=ORIENTED_EDGE('',*,*,#3397,.T.);
#4557=ORIENTED_EDGE('',*,*,#3360,.T.);
#4558=ORIENTED_EDGE('',*,*,#3399,.F.);
#4559=ORIENTED_EDGE('',*,*,#3240,.F.);
#4560=ORIENTED_EDGE('',*,*,#3398,.T.);
#4561=ORIENTED_EDGE('',*,*,#3359,.T.);
#4562=ORIENTED_EDGE('',*,*,#3400,.F.);
#4563=ORIENTED_EDGE('',*,*,#3241,.F.);
#4564=ORIENTED_EDGE('',*,*,#3399,.T.);
#4565=ORIENTED_EDGE('',*,*,#3358,.T.);
#4566=ORIENTED_EDGE('',*,*,#3401,.F.);
#4567=ORIENTED_EDGE('',*,*,#3242,.F.);
#4568=ORIENTED_EDGE('',*,*,#3400,.T.);
#4569=ORIENTED_EDGE('',*,*,#3357,.T.);
#4570=ORIENTED_EDGE('',*,*,#3402,.F.);
#4571=ORIENTED_EDGE('',*,*,#3243,.F.);
#4572=ORIENTED_EDGE('',*,*,#3401,.T.);
#4573=ORIENTED_EDGE('',*,*,#3356,.T.);
#4574=ORIENTED_EDGE('',*,*,#3403,.F.);
#4575=ORIENTED_EDGE('',*,*,#3244,.F.);
#4576=ORIENTED_EDGE('',*,*,#3402,.T.);
#4577=ORIENTED_EDGE('',*,*,#3355,.T.);
#4578=ORIENTED_EDGE('',*,*,#3404,.F.);
#4579=ORIENTED_EDGE('',*,*,#3245,.F.);
#4580=ORIENTED_EDGE('',*,*,#3403,.T.);
#4581=ORIENTED_EDGE('',*,*,#3354,.T.);
#4582=ORIENTED_EDGE('',*,*,#3405,.F.);
#4583=ORIENTED_EDGE('',*,*,#3246,.F.);
#4584=ORIENTED_EDGE('',*,*,#3404,.T.);
#4585=ORIENTED_EDGE('',*,*,#3353,.T.);
#4586=ORIENTED_EDGE('',*,*,#3406,.F.);
#4587=ORIENTED_EDGE('',*,*,#3247,.F.);
#4588=ORIENTED_EDGE('',*,*,#3405,.T.);
#4589=ORIENTED_EDGE('',*,*,#3352,.T.);
#4590=ORIENTED_EDGE('',*,*,#3407,.F.);
#4591=ORIENTED_EDGE('',*,*,#3248,.F.);
#4592=ORIENTED_EDGE('',*,*,#3406,.T.);
#4593=ORIENTED_EDGE('',*,*,#3351,.T.);
#4594=ORIENTED_EDGE('',*,*,#3408,.F.);
#4595=ORIENTED_EDGE('',*,*,#3249,.F.);
#4596=ORIENTED_EDGE('',*,*,#3407,.T.);
#4597=ORIENTED_EDGE('',*,*,#3350,.T.);
#4598=ORIENTED_EDGE('',*,*,#3409,.F.);
#4599=ORIENTED_EDGE('',*,*,#3250,.F.);
#4600=ORIENTED_EDGE('',*,*,#3408,.T.);
#4601=ORIENTED_EDGE('',*,*,#3349,.T.);
#4602=ORIENTED_EDGE('',*,*,#3410,.F.);
#4603=ORIENTED_EDGE('',*,*,#3251,.F.);
#4604=ORIENTED_EDGE('',*,*,#3409,.T.);
#4605=ORIENTED_EDGE('',*,*,#3348,.T.);
#4606=ORIENTED_EDGE('',*,*,#3411,.F.);
#4607=ORIENTED_EDGE('',*,*,#3252,.F.);
#4608=ORIENTED_EDGE('',*,*,#3410,.T.);
#4609=ORIENTED_EDGE('',*,*,#3347,.T.);
#4610=ORIENTED_EDGE('',*,*,#3412,.F.);
#4611=ORIENTED_EDGE('',*,*,#3253,.F.);
#4612=ORIENTED_EDGE('',*,*,#3411,.T.);
#4613=ORIENTED_EDGE('',*,*,#3346,.T.);
#4614=ORIENTED_EDGE('',*,*,#3413,.F.);
#4615=ORIENTED_EDGE('',*,*,#3254,.F.);
#4616=ORIENTED_EDGE('',*,*,#3412,.T.);
#4617=ORIENTED_EDGE('',*,*,#3345,.T.);
#4618=ORIENTED_EDGE('',*,*,#3218,.F.);
#4619=ORIENTED_EDGE('',*,*,#3255,.F.);
#4620=ORIENTED_EDGE('',*,*,#3413,.T.);
#4621=ORIENTED_EDGE('',*,*,#3344,.T.);
#4622=ORIENTED_EDGE('',*,*,#3414,.F.);
#4623=ORIENTED_EDGE('',*,*,#3256,.F.);
#4624=ORIENTED_EDGE('',*,*,#3220,.T.);
#4625=ORIENTED_EDGE('',*,*,#3343,.T.);
#4626=ORIENTED_EDGE('',*,*,#3415,.F.);
#4627=ORIENTED_EDGE('',*,*,#3257,.F.);
#4628=ORIENTED_EDGE('',*,*,#3414,.T.);
#4629=ORIENTED_EDGE('',*,*,#3342,.T.);
#4630=ORIENTED_EDGE('',*,*,#3416,.F.);
#4631=ORIENTED_EDGE('',*,*,#3258,.F.);
#4632=ORIENTED_EDGE('',*,*,#3415,.T.);
#4633=ORIENTED_EDGE('',*,*,#3341,.T.);
#4634=ORIENTED_EDGE('',*,*,#3417,.F.);
#4635=ORIENTED_EDGE('',*,*,#3259,.F.);
#4636=ORIENTED_EDGE('',*,*,#3416,.T.);
#4637=ORIENTED_EDGE('',*,*,#3340,.T.);
#4638=ORIENTED_EDGE('',*,*,#3418,.F.);
#4639=ORIENTED_EDGE('',*,*,#3260,.F.);
#4640=ORIENTED_EDGE('',*,*,#3417,.T.);
#4641=ORIENTED_EDGE('',*,*,#3339,.T.);
#4642=ORIENTED_EDGE('',*,*,#3419,.F.);
#4643=ORIENTED_EDGE('',*,*,#3261,.F.);
#4644=ORIENTED_EDGE('',*,*,#3418,.T.);
#4645=ORIENTED_EDGE('',*,*,#3338,.T.);
#4646=ORIENTED_EDGE('',*,*,#3420,.F.);
#4647=ORIENTED_EDGE('',*,*,#3262,.F.);
#4648=ORIENTED_EDGE('',*,*,#3419,.T.);
#4649=ORIENTED_EDGE('',*,*,#3337,.T.);
#4650=ORIENTED_EDGE('',*,*,#3421,.F.);
#4651=ORIENTED_EDGE('',*,*,#3263,.F.);
#4652=ORIENTED_EDGE('',*,*,#3420,.T.);
#4653=ORIENTED_EDGE('',*,*,#3336,.T.);
#4654=ORIENTED_EDGE('',*,*,#3422,.F.);
#4655=ORIENTED_EDGE('',*,*,#3264,.F.);
#4656=ORIENTED_EDGE('',*,*,#3421,.T.);
#4657=ORIENTED_EDGE('',*,*,#3335,.T.);
#4658=ORIENTED_EDGE('',*,*,#3423,.F.);
#4659=ORIENTED_EDGE('',*,*,#3265,.F.);
#4660=ORIENTED_EDGE('',*,*,#3422,.T.);
#4661=ORIENTED_EDGE('',*,*,#3334,.T.);
#4662=ORIENTED_EDGE('',*,*,#3424,.F.);
#4663=ORIENTED_EDGE('',*,*,#3266,.F.);
#4664=ORIENTED_EDGE('',*,*,#3423,.T.);
#4665=ORIENTED_EDGE('',*,*,#3333,.T.);
#4666=ORIENTED_EDGE('',*,*,#3425,.F.);
#4667=ORIENTED_EDGE('',*,*,#3267,.F.);
#4668=ORIENTED_EDGE('',*,*,#3424,.T.);
#4669=ORIENTED_EDGE('',*,*,#3332,.T.);
#4670=ORIENTED_EDGE('',*,*,#3426,.F.);
#4671=ORIENTED_EDGE('',*,*,#3268,.F.);
#4672=ORIENTED_EDGE('',*,*,#3425,.T.);
#4673=ORIENTED_EDGE('',*,*,#3331,.T.);
#4674=ORIENTED_EDGE('',*,*,#3427,.F.);
#4675=ORIENTED_EDGE('',*,*,#3269,.F.);
#4676=ORIENTED_EDGE('',*,*,#3426,.T.);
#4677=ORIENTED_EDGE('',*,*,#3330,.T.);
#4678=ORIENTED_EDGE('',*,*,#3428,.F.);
#4679=ORIENTED_EDGE('',*,*,#3270,.F.);
#4680=ORIENTED_EDGE('',*,*,#3427,.T.);
#4681=ORIENTED_EDGE('',*,*,#3329,.T.);
#4682=ORIENTED_EDGE('',*,*,#3429,.F.);
#4683=ORIENTED_EDGE('',*,*,#3271,.F.);
#4684=ORIENTED_EDGE('',*,*,#3428,.T.);
#4685=ORIENTED_EDGE('',*,*,#3328,.T.);
#4686=ORIENTED_EDGE('',*,*,#3430,.F.);
#4687=ORIENTED_EDGE('',*,*,#3272,.F.);
#4688=ORIENTED_EDGE('',*,*,#3429,.T.);
#4689=ORIENTED_EDGE('',*,*,#3327,.T.);
#4690=ORIENTED_EDGE('',*,*,#3431,.F.);
#4691=ORIENTED_EDGE('',*,*,#3273,.F.);
#4692=ORIENTED_EDGE('',*,*,#3430,.T.);
#4693=ORIENTED_EDGE('',*,*,#3326,.T.);
#4694=ORIENTED_EDGE('',*,*,#3432,.F.);
#4695=ORIENTED_EDGE('',*,*,#3274,.F.);
#4696=ORIENTED_EDGE('',*,*,#3431,.T.);
#4697=ORIENTED_EDGE('',*,*,#3325,.T.);
#4698=ORIENTED_EDGE('',*,*,#3433,.F.);
#4699=ORIENTED_EDGE('',*,*,#3275,.F.);
#4700=ORIENTED_EDGE('',*,*,#3432,.T.);
#4701=ORIENTED_EDGE('',*,*,#3324,.T.);
#4702=ORIENTED_EDGE('',*,*,#3434,.F.);
#4703=ORIENTED_EDGE('',*,*,#3276,.F.);
#4704=ORIENTED_EDGE('',*,*,#3433,.T.);
#4705=ORIENTED_EDGE('',*,*,#3323,.T.);
#4706=ORIENTED_EDGE('',*,*,#3435,.F.);
#4707=ORIENTED_EDGE('',*,*,#3277,.F.);
#4708=ORIENTED_EDGE('',*,*,#3434,.T.);
#4709=ORIENTED_EDGE('',*,*,#3322,.T.);
#4710=ORIENTED_EDGE('',*,*,#3436,.F.);
#4711=ORIENTED_EDGE('',*,*,#3278,.F.);
#4712=ORIENTED_EDGE('',*,*,#3435,.T.);
#4713=ORIENTED_EDGE('',*,*,#3321,.T.);
#4714=ORIENTED_EDGE('',*,*,#3437,.F.);
#4715=ORIENTED_EDGE('',*,*,#3279,.F.);
#4716=ORIENTED_EDGE('',*,*,#3436,.T.);
#4717=ORIENTED_EDGE('',*,*,#3320,.T.);
#4718=ORIENTED_EDGE('',*,*,#3438,.F.);
#4719=ORIENTED_EDGE('',*,*,#3280,.F.);
#4720=ORIENTED_EDGE('',*,*,#3437,.T.);
#4721=ORIENTED_EDGE('',*,*,#3319,.T.);
#4722=ORIENTED_EDGE('',*,*,#3439,.F.);
#4723=ORIENTED_EDGE('',*,*,#3281,.F.);
#4724=ORIENTED_EDGE('',*,*,#3438,.T.);
#4725=ORIENTED_EDGE('',*,*,#3318,.T.);
#4726=ORIENTED_EDGE('',*,*,#3440,.F.);
#4727=ORIENTED_EDGE('',*,*,#3282,.F.);
#4728=ORIENTED_EDGE('',*,*,#3439,.T.);
#4729=ORIENTED_EDGE('',*,*,#3317,.T.);
#4730=ORIENTED_EDGE('',*,*,#3441,.F.);
#4731=ORIENTED_EDGE('',*,*,#3283,.F.);
#4732=ORIENTED_EDGE('',*,*,#3440,.T.);
#4733=ORIENTED_EDGE('',*,*,#3316,.T.);
#4734=ORIENTED_EDGE('',*,*,#3442,.F.);
#4735=ORIENTED_EDGE('',*,*,#3284,.F.);
#4736=ORIENTED_EDGE('',*,*,#3441,.T.);
#4737=ORIENTED_EDGE('',*,*,#3315,.T.);
#4738=ORIENTED_EDGE('',*,*,#3443,.F.);
#4739=ORIENTED_EDGE('',*,*,#3285,.F.);
#4740=ORIENTED_EDGE('',*,*,#3442,.T.);
#4741=ORIENTED_EDGE('',*,*,#3314,.T.);
#4742=ORIENTED_EDGE('',*,*,#3444,.F.);
#4743=ORIENTED_EDGE('',*,*,#3286,.F.);
#4744=ORIENTED_EDGE('',*,*,#3443,.T.);
#4745=ORIENTED_EDGE('',*,*,#3313,.T.);
#4746=ORIENTED_EDGE('',*,*,#3445,.F.);
#4747=ORIENTED_EDGE('',*,*,#3287,.F.);
#4748=ORIENTED_EDGE('',*,*,#3444,.T.);
#4749=ORIENTED_EDGE('',*,*,#3312,.T.);
#4750=ORIENTED_EDGE('',*,*,#3446,.F.);
#4751=ORIENTED_EDGE('',*,*,#3288,.F.);
#4752=ORIENTED_EDGE('',*,*,#3445,.T.);
#4753=ORIENTED_EDGE('',*,*,#3311,.T.);
#4754=ORIENTED_EDGE('',*,*,#3447,.F.);
#4755=ORIENTED_EDGE('',*,*,#3289,.F.);
#4756=ORIENTED_EDGE('',*,*,#3446,.T.);
#4757=ORIENTED_EDGE('',*,*,#3310,.T.);
#4758=ORIENTED_EDGE('',*,*,#3448,.F.);
#4759=ORIENTED_EDGE('',*,*,#3290,.F.);
#4760=ORIENTED_EDGE('',*,*,#3447,.T.);
#4761=ORIENTED_EDGE('',*,*,#3309,.T.);
#4762=ORIENTED_EDGE('',*,*,#3449,.F.);
#4763=ORIENTED_EDGE('',*,*,#3291,.F.);
#4764=ORIENTED_EDGE('',*,*,#3448,.T.);
#4765=ORIENTED_EDGE('',*,*,#3308,.T.);
#4766=ORIENTED_EDGE('',*,*,#3450,.F.);
#4767=ORIENTED_EDGE('',*,*,#3292,.F.);
#4768=ORIENTED_EDGE('',*,*,#3449,.T.);
#4769=ORIENTED_EDGE('',*,*,#3307,.T.);
#4770=ORIENTED_EDGE('',*,*,#3451,.F.);
#4771=ORIENTED_EDGE('',*,*,#3293,.F.);
#4772=ORIENTED_EDGE('',*,*,#3450,.T.);
#4773=ORIENTED_EDGE('',*,*,#3306,.T.);
#4774=ORIENTED_EDGE('',*,*,#3452,.F.);
#4775=ORIENTED_EDGE('',*,*,#3294,.F.);
#4776=ORIENTED_EDGE('',*,*,#3451,.T.);
#4777=ORIENTED_EDGE('',*,*,#3305,.T.);
#4778=ORIENTED_EDGE('',*,*,#3453,.F.);
#4779=ORIENTED_EDGE('',*,*,#3295,.F.);
#4780=ORIENTED_EDGE('',*,*,#3452,.T.);
#4781=ORIENTED_EDGE('',*,*,#3304,.T.);
#4782=ORIENTED_EDGE('',*,*,#3454,.F.);
#4783=ORIENTED_EDGE('',*,*,#3296,.F.);
#4784=ORIENTED_EDGE('',*,*,#3453,.T.);
#4785=ORIENTED_EDGE('',*,*,#3303,.T.);
#4786=ORIENTED_EDGE('',*,*,#3455,.F.);
#4787=ORIENTED_EDGE('',*,*,#3297,.F.);
#4788=ORIENTED_EDGE('',*,*,#3454,.T.);
#4789=ORIENTED_EDGE('',*,*,#3302,.T.);
#4790=ORIENTED_EDGE('',*,*,#3456,.F.);
#4791=ORIENTED_EDGE('',*,*,#3298,.F.);
#4792=ORIENTED_EDGE('',*,*,#3455,.T.);
#4793=ORIENTED_EDGE('',*,*,#3301,.T.);
#4794=ORIENTED_EDGE('',*,*,#3380,.F.);
#4795=ORIENTED_EDGE('',*,*,#3299,.F.);
#4796=ORIENTED_EDGE('',*,*,#3456,.T.);
#4797=ORIENTED_EDGE('',*,*,#3211,.T.);
#4798=ORIENTED_EDGE('',*,*,#3210,.F.);
#4799=ORIENTED_EDGE('',*,*,#3205,.T.);
#4800=ORIENTED_EDGE('',*,*,#3204,.F.);
#5210=CYLINDRICAL_SURFACE('',#5885,7.);
#5211=CYLINDRICAL_SURFACE('',#5888,14.);
#5212=CYLINDRICAL_SURFACE('',#5891,7.);
#5213=CYLINDRICAL_SURFACE('',#5894,14.);
#5214=CYLINDRICAL_SURFACE('',#5897,2.5);
#5215=CYLINDRICAL_SURFACE('',#5900,16.25);
#5216=CYLINDRICAL_SURFACE('',#5985,19.);
#5217=CYLINDRICAL_SURFACE('',#5986,16.25);
#5218=CYLINDRICAL_SURFACE('',#5987,19.);
#5219=CYLINDRICAL_SURFACE('',#5988,16.25);
#5220=CYLINDRICAL_SURFACE('',#5989,19.);
#5221=CYLINDRICAL_SURFACE('',#5990,16.25);
#5222=CYLINDRICAL_SURFACE('',#5991,19.);
#5223=CYLINDRICAL_SURFACE('',#5992,16.25);
#5224=CYLINDRICAL_SURFACE('',#5993,19.);
#5225=CYLINDRICAL_SURFACE('',#5994,16.25);
#5226=CYLINDRICAL_SURFACE('',#5995,19.);
#5227=CYLINDRICAL_SURFACE('',#5996,16.25);
#5228=CYLINDRICAL_SURFACE('',#5997,19.);
#5229=CYLINDRICAL_SURFACE('',#5998,16.25);
#5230=CYLINDRICAL_SURFACE('',#5999,19.);
#5231=CYLINDRICAL_SURFACE('',#6000,16.25);
#5232=CYLINDRICAL_SURFACE('',#6001,19.);
#5233=CYLINDRICAL_SURFACE('',#6002,19.);
#5234=CYLINDRICAL_SURFACE('',#6003,16.25);
#5235=CYLINDRICAL_SURFACE('',#6004,19.);
#5236=CYLINDRICAL_SURFACE('',#6005,16.25);
#5237=CYLINDRICAL_SURFACE('',#6006,19.);
#5238=CYLINDRICAL_SURFACE('',#6007,16.25);
#5239=CYLINDRICAL_SURFACE('',#6008,19.);
#5240=CYLINDRICAL_SURFACE('',#6009,16.25);
#5241=CYLINDRICAL_SURFACE('',#6010,19.);
#5242=CYLINDRICAL_SURFACE('',#6011,16.25);
#5243=CYLINDRICAL_SURFACE('',#6012,19.);
#5244=CYLINDRICAL_SURFACE('',#6013,16.25);
#5245=CYLINDRICAL_SURFACE('',#6014,19.);
#5246=CYLINDRICAL_SURFACE('',#6015,16.25);
#5247=CYLINDRICAL_SURFACE('',#6016,19.);
#5248=CYLINDRICAL_SURFACE('',#6017,16.25);
#5249=CYLINDRICAL_SURFACE('',#6018,19.);
#5250=CYLINDRICAL_SURFACE('',#6019,16.25);
#5251=CYLINDRICAL_SURFACE('',#6020,19.);
#5252=CYLINDRICAL_SURFACE('',#6021,16.25);
#5253=CYLINDRICAL_SURFACE('',#6022,19.);
#5254=CYLINDRICAL_SURFACE('',#6023,16.25);
#5395=ADVANCED_FACE('',(#678),#5210,.T.);
#5396=ADVANCED_FACE('',(#679),#5211,.F.);
#5397=ADVANCED_FACE('',(#680),#5212,.T.);
#5398=ADVANCED_FACE('',(#681),#5213,.F.);
#5399=ADVANCED_FACE('',(#682),#5214,.F.);
#5400=ADVANCED_FACE('',(#683),#5215,.T.);
#5401=ADVANCED_FACE('',(#684,#367),#480,.F.);
#5402=ADVANCED_FACE('',(#685,#368),#481,.T.);
#5403=ADVANCED_FACE('',(#686,#369),#482,.T.);
#5404=ADVANCED_FACE('',(#687,#370),#483,.F.);
#5405=ADVANCED_FACE('',(#688),#167,.F.);
#5406=ADVANCED_FACE('',(#689),#5216,.T.);
#5407=ADVANCED_FACE('',(#690),#168,.F.);
#5408=ADVANCED_FACE('',(#691),#5217,.T.);
#5409=ADVANCED_FACE('',(#692),#169,.F.);
#5410=ADVANCED_FACE('',(#693),#5218,.T.);
#5411=ADVANCED_FACE('',(#694),#170,.F.);
#5412=ADVANCED_FACE('',(#695),#5219,.T.);
#5413=ADVANCED_FACE('',(#696),#171,.F.);
#5414=ADVANCED_FACE('',(#697),#5220,.T.);
#5415=ADVANCED_FACE('',(#698),#172,.F.);
#5416=ADVANCED_FACE('',(#699),#5221,.T.);
#5417=ADVANCED_FACE('',(#700),#173,.F.);
#5418=ADVANCED_FACE('',(#701),#5222,.T.);
#5419=ADVANCED_FACE('',(#702),#174,.F.);
#5420=ADVANCED_FACE('',(#703),#5223,.T.);
#5421=ADVANCED_FACE('',(#704),#175,.F.);
#5422=ADVANCED_FACE('',(#705),#5224,.T.);
#5423=ADVANCED_FACE('',(#706),#176,.F.);
#5424=ADVANCED_FACE('',(#707),#5225,.T.);
#5425=ADVANCED_FACE('',(#708),#177,.F.);
#5426=ADVANCED_FACE('',(#709),#5226,.T.);
#5427=ADVANCED_FACE('',(#710),#178,.F.);
#5428=ADVANCED_FACE('',(#711),#5227,.T.);
#5429=ADVANCED_FACE('',(#712),#179,.F.);
#5430=ADVANCED_FACE('',(#713),#5228,.T.);
#5431=ADVANCED_FACE('',(#714),#180,.F.);
#5432=ADVANCED_FACE('',(#715),#5229,.T.);
#5433=ADVANCED_FACE('',(#716),#181,.F.);
#5434=ADVANCED_FACE('',(#717),#5230,.T.);
#5435=ADVANCED_FACE('',(#718),#182,.F.);
#5436=ADVANCED_FACE('',(#719),#5231,.T.);
#5437=ADVANCED_FACE('',(#720),#183,.F.);
#5438=ADVANCED_FACE('',(#721),#5232,.T.);
#5439=ADVANCED_FACE('',(#722),#184,.F.);
#5440=ADVANCED_FACE('',(#723),#185,.F.);
#5441=ADVANCED_FACE('',(#724),#5233,.T.);
#5442=ADVANCED_FACE('',(#725),#186,.F.);
#5443=ADVANCED_FACE('',(#726),#5234,.T.);
#5444=ADVANCED_FACE('',(#727),#187,.F.);
#5445=ADVANCED_FACE('',(#728),#5235,.T.);
#5446=ADVANCED_FACE('',(#729),#188,.F.);
#5447=ADVANCED_FACE('',(#730),#5236,.T.);
#5448=ADVANCED_FACE('',(#731),#189,.F.);
#5449=ADVANCED_FACE('',(#732),#5237,.T.);
#5450=ADVANCED_FACE('',(#733),#190,.F.);
#5451=ADVANCED_FACE('',(#734),#5238,.T.);
#5452=ADVANCED_FACE('',(#735),#191,.F.);
#5453=ADVANCED_FACE('',(#736),#5239,.T.);
#5454=ADVANCED_FACE('',(#737),#192,.F.);
#5455=ADVANCED_FACE('',(#738),#5240,.T.);
#5456=ADVANCED_FACE('',(#739),#193,.F.);
#5457=ADVANCED_FACE('',(#740),#5241,.T.);
#5458=ADVANCED_FACE('',(#741),#194,.F.);
#5459=ADVANCED_FACE('',(#742),#5242,.T.);
#5460=ADVANCED_FACE('',(#743),#195,.F.);
#5461=ADVANCED_FACE('',(#744),#5243,.T.);
#5462=ADVANCED_FACE('',(#745),#196,.F.);
#5463=ADVANCED_FACE('',(#746),#5244,.T.);
#5464=ADVANCED_FACE('',(#747),#197,.F.);
#5465=ADVANCED_FACE('',(#748),#5245,.T.);
#5466=ADVANCED_FACE('',(#749),#198,.F.);
#5467=ADVANCED_FACE('',(#750),#5246,.T.);
#5468=ADVANCED_FACE('',(#751),#199,.F.);
#5469=ADVANCED_FACE('',(#752),#5247,.T.);
#5470=ADVANCED_FACE('',(#753),#200,.F.);
#5471=ADVANCED_FACE('',(#754),#5248,.T.);
#5472=ADVANCED_FACE('',(#755),#201,.F.);
#5473=ADVANCED_FACE('',(#756),#5249,.T.);
#5474=ADVANCED_FACE('',(#757),#202,.F.);
#5475=ADVANCED_FACE('',(#758),#5250,.T.);
#5476=ADVANCED_FACE('',(#759),#203,.F.);
#5477=ADVANCED_FACE('',(#760),#5251,.T.);
#5478=ADVANCED_FACE('',(#761),#204,.F.);
#5479=ADVANCED_FACE('',(#762),#5252,.T.);
#5480=ADVANCED_FACE('',(#763),#205,.F.);
#5481=ADVANCED_FACE('',(#764),#5253,.T.);
#5482=ADVANCED_FACE('',(#765),#206,.F.);
#5483=ADVANCED_FACE('',(#766),#5254,.T.);
#5484=ADVANCED_FACE('',(#767,#371),#484,.T.);
#5485=ADVANCED_FACE('',(#768,#372),#485,.T.);
#5584=CLOSED_SHELL('',(#5395,#5396,#5397,#5398,#5399,#5400,#5401,#5402,
#5403,#5404,#5405,#5406,#5407,#5408,#5409,#5410,#5411,#5412,#5413,#5414,
#5415,#5416,#5417,#5418,#5419,#5420,#5421,#5422,#5423,#5424,#5425,#5426,
#5427,#5428,#5429,#5430,#5431,#5432,#5433,#5434,#5435,#5436,#5437,#5438,
#5439,#5440,#5441,#5442,#5443,#5444,#5445,#5446,#5447,#5448,#5449,#5450,
#5451,#5452,#5453,#5454,#5455,#5456,#5457,#5458,#5459,#5460,#5461,#5462,
#5463,#5464,#5465,#5466,#5467,#5468,#5469,#5470,#5471,#5472,#5473,#5474,
#5475,#5476,#5477,#5478,#5479,#5480,#5481,#5482,#5483,#5484,#5485));
#5884=AXIS2_PLACEMENT_3D('',#8436,#6882,#6883);
#5885=AXIS2_PLACEMENT_3D('',#8437,#6884,#6885);
#5886=AXIS2_PLACEMENT_3D('',#8439,#6886,#6887);
#5887=AXIS2_PLACEMENT_3D('',#8442,#6889,#6890);
#5888=AXIS2_PLACEMENT_3D('',#8443,#6891,#6892);
#5889=AXIS2_PLACEMENT_3D('',#8445,#6893,#6894);
#5890=AXIS2_PLACEMENT_3D('',#8448,#6896,#6897);
#5891=AXIS2_PLACEMENT_3D('',#8449,#6898,#6899);
#5892=AXIS2_PLACEMENT_3D('',#8451,#6900,#6901);
#5893=AXIS2_PLACEMENT_3D('',#8454,#6903,#6904);
#5894=AXIS2_PLACEMENT_3D('',#8455,#6905,#6906);
#5895=AXIS2_PLACEMENT_3D('',#8457,#6907,#6908);
#5896=AXIS2_PLACEMENT_3D('',#8460,#6910,#6911);
#5897=AXIS2_PLACEMENT_3D('',#8461,#6912,#6913);
#5898=AXIS2_PLACEMENT_3D('',#8463,#6914,#6915);
#5899=AXIS2_PLACEMENT_3D('',#8466,#6917,#6918);
#5900=AXIS2_PLACEMENT_3D('',#8467,#6919,#6920);
#5901=AXIS2_PLACEMENT_3D('',#8470,#6921,#6922);
#5902=AXIS2_PLACEMENT_3D('',#8474,#6924,#6925);
#5903=AXIS2_PLACEMENT_3D('',#8476,#6927,#6928);
#5904=AXIS2_PLACEMENT_3D('',#8477,#6929,#6930);
#5905=AXIS2_PLACEMENT_3D('',#8478,#6931,#6932);
#5906=AXIS2_PLACEMENT_3D('',#8505,#6933,#6934);
#5907=AXIS2_PLACEMENT_3D('',#8531,#6935,#6936);
#5908=AXIS2_PLACEMENT_3D('',#8557,#6937,#6938);
#5909=AXIS2_PLACEMENT_3D('',#8583,#6939,#6940);
#5910=AXIS2_PLACEMENT_3D('',#8609,#6941,#6942);
#5911=AXIS2_PLACEMENT_3D('',#8635,#6943,#6944);
#5912=AXIS2_PLACEMENT_3D('',#8661,#6945,#6946);
#5913=AXIS2_PLACEMENT_3D('',#8687,#6947,#6948);
#5914=AXIS2_PLACEMENT_3D('',#8713,#6949,#6950);
#5915=AXIS2_PLACEMENT_3D('',#8739,#6951,#6952);
#5916=AXIS2_PLACEMENT_3D('',#8765,#6953,#6954);
#5917=AXIS2_PLACEMENT_3D('',#8791,#6955,#6956);
#5918=AXIS2_PLACEMENT_3D('',#8817,#6957,#6958);
#5919=AXIS2_PLACEMENT_3D('',#8843,#6959,#6960);
#5920=AXIS2_PLACEMENT_3D('',#8869,#6961,#6962);
#5921=AXIS2_PLACEMENT_3D('',#8895,#6963,#6964);
#5922=AXIS2_PLACEMENT_3D('',#8921,#6965,#6966);
#5923=AXIS2_PLACEMENT_3D('',#8970,#6967,#6968);
#5924=AXIS2_PLACEMENT_3D('',#8996,#6969,#6970);
#5925=AXIS2_PLACEMENT_3D('',#9022,#6971,#6972);
#5926=AXIS2_PLACEMENT_3D('',#9048,#6973,#6974);
#5927=AXIS2_PLACEMENT_3D('',#9074,#6975,#6976);
#5928=AXIS2_PLACEMENT_3D('',#9100,#6977,#6978);
#5929=AXIS2_PLACEMENT_3D('',#9126,#6979,#6980);
#5930=AXIS2_PLACEMENT_3D('',#9152,#6981,#6982);
#5931=AXIS2_PLACEMENT_3D('',#9178,#6983,#6984);
#5932=AXIS2_PLACEMENT_3D('',#9204,#6985,#6986);
#5933=AXIS2_PLACEMENT_3D('',#9230,#6987,#6988);
#5934=AXIS2_PLACEMENT_3D('',#9256,#6989,#6990);
#5935=AXIS2_PLACEMENT_3D('',#9282,#6991,#6992);
#5936=AXIS2_PLACEMENT_3D('',#9308,#6993,#6994);
#5937=AXIS2_PLACEMENT_3D('',#9334,#6995,#6996);
#5938=AXIS2_PLACEMENT_3D('',#9360,#6997,#6998);
#5939=AXIS2_PLACEMENT_3D('',#9386,#6999,#7000);
#5940=AXIS2_PLACEMENT_3D('',#9412,#7001,#7002);
#5941=AXIS2_PLACEMENT_3D('',#9438,#7003,#7004);
#5942=AXIS2_PLACEMENT_3D('',#9464,#7005,#7006);
#5943=AXIS2_PLACEMENT_3D('',#9490,#7007,#7008);
#5944=AXIS2_PLACEMENT_3D('',#9515,#7009,#7010);
#5945=AXIS2_PLACEMENT_3D('',#9516,#7011,#7012);
#5946=AXIS2_PLACEMENT_3D('',#9543,#7013,#7014);
#5947=AXIS2_PLACEMENT_3D('',#9569,#7015,#7016);
#5948=AXIS2_PLACEMENT_3D('',#9595,#7017,#7018);
#5949=AXIS2_PLACEMENT_3D('',#9621,#7019,#7020);
#5950=AXIS2_PLACEMENT_3D('',#9647,#7021,#7022);
#5951=AXIS2_PLACEMENT_3D('',#9673,#7023,#7024);
#5952=AXIS2_PLACEMENT_3D('',#9699,#7025,#7026);
#5953=AXIS2_PLACEMENT_3D('',#9725,#7027,#7028);
#5954=AXIS2_PLACEMENT_3D('',#9751,#7029,#7030);
#5955=AXIS2_PLACEMENT_3D('',#9777,#7031,#7032);
#5956=AXIS2_PLACEMENT_3D('',#9803,#7033,#7034);
#5957=AXIS2_PLACEMENT_3D('',#9829,#7035,#7036);
#5958=AXIS2_PLACEMENT_3D('',#9855,#7037,#7038);
#5959=AXIS2_PLACEMENT_3D('',#9881,#7039,#7040);
#5960=AXIS2_PLACEMENT_3D('',#9907,#7041,#7042);
#5961=AXIS2_PLACEMENT_3D('',#9933,#7043,#7044);
#5962=AXIS2_PLACEMENT_3D('',#9959,#7045,#7046);
#5963=AXIS2_PLACEMENT_3D('',#9985,#7047,#7048);
#5964=AXIS2_PLACEMENT_3D('',#10011,#7049,#7050);
#5965=AXIS2_PLACEMENT_3D('',#10037,#7051,#7052);
#5966=AXIS2_PLACEMENT_3D('',#10063,#7053,#7054);
#5967=AXIS2_PLACEMENT_3D('',#10089,#7055,#7056);
#5968=AXIS2_PLACEMENT_3D('',#10138,#7057,#7058);
#5969=AXIS2_PLACEMENT_3D('',#10164,#7059,#7060);
#5970=AXIS2_PLACEMENT_3D('',#10190,#7061,#7062);
#5971=AXIS2_PLACEMENT_3D('',#10216,#7063,#7064);
#5972=AXIS2_PLACEMENT_3D('',#10242,#7065,#7066);
#5973=AXIS2_PLACEMENT_3D('',#10268,#7067,#7068);
#5974=AXIS2_PLACEMENT_3D('',#10294,#7069,#7070);
#5975=AXIS2_PLACEMENT_3D('',#10320,#7071,#7072);
#5976=AXIS2_PLACEMENT_3D('',#10346,#7073,#7074);
#5977=AXIS2_PLACEMENT_3D('',#10372,#7075,#7076);
#5978=AXIS2_PLACEMENT_3D('',#10398,#7077,#7078);
#5979=AXIS2_PLACEMENT_3D('',#10424,#7079,#7080);
#5980=AXIS2_PLACEMENT_3D('',#10450,#7081,#7082);
#5981=AXIS2_PLACEMENT_3D('',#10476,#7083,#7084);
#5982=AXIS2_PLACEMENT_3D('',#10502,#7085,#7086);
#5983=AXIS2_PLACEMENT_3D('',#10528,#7087,#7088);
#5984=AXIS2_PLACEMENT_3D('',#10553,#7089,#7090);
#5985=AXIS2_PLACEMENT_3D('',#10602,#7093,#7094);
#5986=AXIS2_PLACEMENT_3D('',#10651,#7097,#7098);
#5987=AXIS2_PLACEMENT_3D('',#10700,#7101,#7102);
#5988=AXIS2_PLACEMENT_3D('',#10749,#7105,#7106);
#5989=AXIS2_PLACEMENT_3D('',#10798,#7109,#7110);
#5990=AXIS2_PLACEMENT_3D('',#10847,#7113,#7114);
#5991=AXIS2_PLACEMENT_3D('',#10896,#7117,#7118);
#5992=AXIS2_PLACEMENT_3D('',#10945,#7121,#7122);
#5993=AXIS2_PLACEMENT_3D('',#10994,#7125,#7126);
#5994=AXIS2_PLACEMENT_3D('',#11043,#7129,#7130);
#5995=AXIS2_PLACEMENT_3D('',#11092,#7133,#7134);
#5996=AXIS2_PLACEMENT_3D('',#11141,#7137,#7138);
#5997=AXIS2_PLACEMENT_3D('',#11190,#7141,#7142);
#5998=AXIS2_PLACEMENT_3D('',#11239,#7145,#7146);
#5999=AXIS2_PLACEMENT_3D('',#11288,#7149,#7150);
#6000=AXIS2_PLACEMENT_3D('',#11337,#7153,#7154);
#6001=AXIS2_PLACEMENT_3D('',#11386,#7157,#7158);
#6002=AXIS2_PLACEMENT_3D('',#11481,#7161,#7162);
#6003=AXIS2_PLACEMENT_3D('',#11530,#7165,#7166);
#6004=AXIS2_PLACEMENT_3D('',#11579,#7169,#7170);
#6005=AXIS2_PLACEMENT_3D('',#11628,#7173,#7174);
#6006=AXIS2_PLACEMENT_3D('',#11677,#7177,#7178);
#6007=AXIS2_PLACEMENT_3D('',#11726,#7181,#7182);
#6008=AXIS2_PLACEMENT_3D('',#11775,#7185,#7186);
#6009=AXIS2_PLACEMENT_3D('',#11824,#7189,#7190);
#6010=AXIS2_PLACEMENT_3D('',#11873,#7193,#7194);
#6011=AXIS2_PLACEMENT_3D('',#11922,#7197,#7198);
#6012=AXIS2_PLACEMENT_3D('',#11971,#7201,#7202);
#6013=AXIS2_PLACEMENT_3D('',#12020,#7205,#7206);
#6014=AXIS2_PLACEMENT_3D('',#12069,#7209,#7210);
#6015=AXIS2_PLACEMENT_3D('',#12118,#7213,#7214);
#6016=AXIS2_PLACEMENT_3D('',#12167,#7217,#7218);
#6017=AXIS2_PLACEMENT_3D('',#12216,#7221,#7222);
#6018=AXIS2_PLACEMENT_3D('',#12265,#7225,#7226);
#6019=AXIS2_PLACEMENT_3D('',#12314,#7229,#7230);
#6020=AXIS2_PLACEMENT_3D('',#12363,#7233,#7234);
#6021=AXIS2_PLACEMENT_3D('',#12412,#7237,#7238);
#6022=AXIS2_PLACEMENT_3D('',#12461,#7241,#7242);
#6023=AXIS2_PLACEMENT_3D('',#12510,#7245,#7246);
#6024=AXIS2_PLACEMENT_3D('',#12511,#7247,#7248);
#6025=AXIS2_PLACEMENT_3D('',#12512,#7249,#7250);
#6882=DIRECTION('axis',(0.,0.,1.));
#6883=DIRECTION('refdir',(1.,0.,0.));
#6884=DIRECTION('center_axis',(0.,0.,-1.));
#6885=DIRECTION('ref_axis',(-1.,0.,0.));
#6886=DIRECTION('center_axis',(0.,0.,-1.));
#6887=DIRECTION('ref_axis',(-1.,0.,0.));
#6888=DIRECTION('',(0.,0.,1.));
#6889=DIRECTION('center_axis',(0.,0.,-1.));
#6890=DIRECTION('ref_axis',(-1.,0.,0.));
#6891=DIRECTION('center_axis',(0.,0.,-1.));
#6892=DIRECTION('ref_axis',(-1.,0.,0.));
#6893=DIRECTION('center_axis',(0.,0.,-1.));
#6894=DIRECTION('ref_axis',(-1.,0.,0.));
#6895=DIRECTION('',(0.,0.,-1.));
#6896=DIRECTION('center_axis',(0.,0.,-1.));
#6897=DIRECTION('ref_axis',(-1.,0.,0.));
#6898=DIRECTION('center_axis',(0.,0.,1.));
#6899=DIRECTION('ref_axis',(1.,0.,0.));
#6900=DIRECTION('center_axis',(0.,0.,1.));
#6901=DIRECTION('ref_axis',(1.,0.,0.));
#6902=DIRECTION('',(0.,0.,-1.));
#6903=DIRECTION('center_axis',(0.,0.,1.));
#6904=DIRECTION('ref_axis',(1.,0.,0.));
#6905=DIRECTION('center_axis',(0.,0.,1.));
#6906=DIRECTION('ref_axis',(1.,0.,0.));
#6907=DIRECTION('center_axis',(0.,0.,1.));
#6908=DIRECTION('ref_axis',(1.,0.,0.));
#6909=DIRECTION('',(0.,0.,1.));
#6910=DIRECTION('center_axis',(0.,0.,1.));
#6911=DIRECTION('ref_axis',(1.,0.,0.));
#6912=DIRECTION('center_axis',(0.,0.,-1.));
#6913=DIRECTION('ref_axis',(-1.,0.,0.));
#6914=DIRECTION('center_axis',(0.,0.,1.));
#6915=DIRECTION('ref_axis',(1.,0.,0.));
#6916=DIRECTION('',(0.,0.,-1.));
#6917=DIRECTION('center_axis',(0.,0.,1.));
#6918=DIRECTION('ref_axis',(1.,0.,0.));
#6919=DIRECTION('center_axis',(0.,0.,-1.));
#6920=DIRECTION('ref_axis',(-1.,0.,0.));
#6921=DIRECTION('center_axis',(0.,0.,1.));
#6922=DIRECTION('ref_axis',(1.,0.,0.));
#6923=DIRECTION('',(0.,0.,-1.));
#6924=DIRECTION('center_axis',(0.,0.,1.));
#6925=DIRECTION('ref_axis',(1.,0.,0.));
#6926=DIRECTION('',(0.,0.,-1.));
#6927=DIRECTION('center_axis',(0.,0.,1.));
#6928=DIRECTION('ref_axis',(1.,0.,0.));
#6929=DIRECTION('center_axis',(0.,0.,1.));
#6930=DIRECTION('ref_axis',(1.,0.,0.));
#6931=DIRECTION('center_axis',(0.,0.,1.));
#6932=DIRECTION('ref_axis',(1.,0.,0.));
#6933=DIRECTION('center_axis',(0.,0.,1.));
#6934=DIRECTION('ref_axis',(1.,0.,0.));
#6935=DIRECTION('center_axis',(0.,0.,1.));
#6936=DIRECTION('ref_axis',(1.,0.,0.));
#6937=DIRECTION('center_axis',(0.,0.,1.));
#6938=DIRECTION('ref_axis',(1.,0.,0.));
#6939=DIRECTION('center_axis',(0.,0.,1.));
#6940=DIRECTION('ref_axis',(1.,0.,0.));
#6941=DIRECTION('center_axis',(0.,0.,1.));
#6942=DIRECTION('ref_axis',(1.,0.,0.));
#6943=DIRECTION('center_axis',(0.,0.,1.));
#6944=DIRECTION('ref_axis',(1.,0.,0.));
#6945=DIRECTION('center_axis',(0.,0.,1.));
#6946=DIRECTION('ref_axis',(1.,0.,0.));
#6947=DIRECTION('center_axis',(0.,0.,1.));
#6948=DIRECTION('ref_axis',(1.,0.,0.));
#6949=DIRECTION('center_axis',(0.,0.,1.));
#6950=DIRECTION('ref_axis',(1.,0.,0.));
#6951=DIRECTION('center_axis',(0.,0.,1.));
#6952=DIRECTION('ref_axis',(1.,0.,0.));
#6953=DIRECTION('center_axis',(0.,0.,1.));
#6954=DIRECTION('ref_axis',(1.,0.,0.));
#6955=DIRECTION('center_axis',(0.,0.,1.));
#6956=DIRECTION('ref_axis',(1.,0.,0.));
#6957=DIRECTION('center_axis',(0.,0.,1.));
#6958=DIRECTION('ref_axis',(1.,0.,0.));
#6959=DIRECTION('center_axis',(0.,0.,1.));
#6960=DIRECTION('ref_axis',(1.,0.,0.));
#6961=DIRECTION('center_axis',(0.,0.,1.));
#6962=DIRECTION('ref_axis',(1.,0.,0.));
#6963=DIRECTION('center_axis',(0.,0.,1.));
#6964=DIRECTION('ref_axis',(1.,0.,0.));
#6965=DIRECTION('center_axis',(0.,0.,1.));
#6966=DIRECTION('ref_axis',(1.,0.,0.));
#6967=DIRECTION('center_axis',(0.,0.,1.));
#6968=DIRECTION('ref_axis',(1.,0.,0.));
#6969=DIRECTION('center_axis',(0.,0.,1.));
#6970=DIRECTION('ref_axis',(1.,0.,0.));
#6971=DIRECTION('center_axis',(0.,0.,1.));
#6972=DIRECTION('ref_axis',(1.,0.,0.));
#6973=DIRECTION('center_axis',(0.,0.,1.));
#6974=DIRECTION('ref_axis',(1.,0.,0.));
#6975=DIRECTION('center_axis',(0.,0.,1.));
#6976=DIRECTION('ref_axis',(1.,0.,0.));
#6977=DIRECTION('center_axis',(0.,0.,1.));
#6978=DIRECTION('ref_axis',(1.,0.,0.));
#6979=DIRECTION('center_axis',(0.,0.,1.));
#6980=DIRECTION('ref_axis',(1.,0.,0.));
#6981=DIRECTION('center_axis',(0.,0.,1.));
#6982=DIRECTION('ref_axis',(1.,0.,0.));
#6983=DIRECTION('center_axis',(0.,0.,1.));
#6984=DIRECTION('ref_axis',(1.,0.,0.));
#6985=DIRECTION('center_axis',(0.,0.,1.));
#6986=DIRECTION('ref_axis',(1.,0.,0.));
#6987=DIRECTION('center_axis',(0.,0.,1.));
#6988=DIRECTION('ref_axis',(1.,0.,0.));
#6989=DIRECTION('center_axis',(0.,0.,1.));
#6990=DIRECTION('ref_axis',(1.,0.,0.));
#6991=DIRECTION('center_axis',(0.,0.,1.));
#6992=DIRECTION('ref_axis',(1.,0.,0.));
#6993=DIRECTION('center_axis',(0.,0.,1.));
#6994=DIRECTION('ref_axis',(1.,0.,0.));
#6995=DIRECTION('center_axis',(0.,0.,1.));
#6996=DIRECTION('ref_axis',(1.,0.,0.));
#6997=DIRECTION('center_axis',(0.,0.,1.));
#6998=DIRECTION('ref_axis',(1.,0.,0.));
#6999=DIRECTION('center_axis',(0.,0.,1.));
#7000=DIRECTION('ref_axis',(1.,0.,0.));
#7001=DIRECTION('center_axis',(0.,0.,1.));
#7002=DIRECTION('ref_axis',(1.,0.,0.));
#7003=DIRECTION('center_axis',(0.,0.,1.));
#7004=DIRECTION('ref_axis',(1.,0.,0.));
#7005=DIRECTION('center_axis',(0.,0.,1.));
#7006=DIRECTION('ref_axis',(1.,0.,0.));
#7007=DIRECTION('center_axis',(0.,0.,1.));
#7008=DIRECTION('ref_axis',(1.,0.,0.));
#7009=DIRECTION('center_axis',(0.,0.,1.));
#7010=DIRECTION('ref_axis',(1.,0.,0.));
#7011=DIRECTION('center_axis',(0.,0.,1.));
#7012=DIRECTION('ref_axis',(1.,0.,0.));
#7013=DIRECTION('center_axis',(0.,0.,1.));
#7014=DIRECTION('ref_axis',(1.,0.,0.));
#7015=DIRECTION('center_axis',(0.,0.,1.));
#7016=DIRECTION('ref_axis',(1.,0.,0.));
#7017=DIRECTION('center_axis',(0.,0.,1.));
#7018=DIRECTION('ref_axis',(1.,0.,0.));
#7019=DIRECTION('center_axis',(0.,0.,1.));
#7020=DIRECTION('ref_axis',(1.,0.,0.));
#7021=DIRECTION('center_axis',(0.,0.,1.));
#7022=DIRECTION('ref_axis',(1.,0.,0.));
#7023=DIRECTION('center_axis',(0.,0.,1.));
#7024=DIRECTION('ref_axis',(1.,0.,0.));
#7025=DIRECTION('center_axis',(0.,0.,1.));
#7026=DIRECTION('ref_axis',(1.,0.,0.));
#7027=DIRECTION('center_axis',(0.,0.,1.));
#7028=DIRECTION('ref_axis',(1.,0.,0.));
#7029=DIRECTION('center_axis',(0.,0.,1.));
#7030=DIRECTION('ref_axis',(1.,0.,0.));
#7031=DIRECTION('center_axis',(0.,0.,1.));
#7032=DIRECTION('ref_axis',(1.,0.,0.));
#7033=DIRECTION('center_axis',(0.,0.,1.));
#7034=DIRECTION('ref_axis',(1.,0.,0.));
#7035=DIRECTION('center_axis',(0.,0.,1.));
#7036=DIRECTION('ref_axis',(1.,0.,0.));
#7037=DIRECTION('center_axis',(0.,0.,1.));
#7038=DIRECTION('ref_axis',(1.,0.,0.));
#7039=DIRECTION('center_axis',(0.,0.,1.));
#7040=DIRECTION('ref_axis',(1.,0.,0.));
#7041=DIRECTION('center_axis',(0.,0.,1.));
#7042=DIRECTION('ref_axis',(1.,0.,0.));
#7043=DIRECTION('center_axis',(0.,0.,1.));
#7044=DIRECTION('ref_axis',(1.,0.,0.));
#7045=DIRECTION('center_axis',(0.,0.,1.));
#7046=DIRECTION('ref_axis',(1.,0.,0.));
#7047=DIRECTION('center_axis',(0.,0.,1.));
#7048=DIRECTION('ref_axis',(1.,0.,0.));
#7049=DIRECTION('center_axis',(0.,0.,1.));
#7050=DIRECTION('ref_axis',(1.,0.,0.));
#7051=DIRECTION('center_axis',(0.,0.,1.));
#7052=DIRECTION('ref_axis',(1.,0.,0.));
#7053=DIRECTION('center_axis',(0.,0.,1.));
#7054=DIRECTION('ref_axis',(1.,0.,0.));
#7055=DIRECTION('center_axis',(0.,0.,1.));
#7056=DIRECTION('ref_axis',(1.,0.,0.));
#7057=DIRECTION('center_axis',(0.,0.,1.));
#7058=DIRECTION('ref_axis',(1.,0.,0.));
#7059=DIRECTION('center_axis',(0.,0.,1.));
#7060=DIRECTION('ref_axis',(1.,0.,0.));
#7061=DIRECTION('center_axis',(0.,0.,1.));
#7062=DIRECTION('ref_axis',(1.,0.,0.));
#7063=DIRECTION('center_axis',(0.,0.,1.));
#7064=DIRECTION('ref_axis',(1.,0.,0.));
#7065=DIRECTION('center_axis',(0.,0.,1.));
#7066=DIRECTION('ref_axis',(1.,0.,0.));
#7067=DIRECTION('center_axis',(0.,0.,1.));
#7068=DIRECTION('ref_axis',(1.,0.,0.));
#7069=DIRECTION('center_axis',(0.,0.,1.));
#7070=DIRECTION('ref_axis',(1.,0.,0.));
#7071=DIRECTION('center_axis',(0.,0.,1.));
#7072=DIRECTION('ref_axis',(1.,0.,0.));
#7073=DIRECTION('center_axis',(0.,0.,1.));
#7074=DIRECTION('ref_axis',(1.,0.,0.));
#7075=DIRECTION('center_axis',(0.,0.,1.));
#7076=DIRECTION('ref_axis',(1.,0.,0.));
#7077=DIRECTION('center_axis',(0.,0.,1.));
#7078=DIRECTION('ref_axis',(1.,0.,0.));
#7079=DIRECTION('center_axis',(0.,0.,1.));
#7080=DIRECTION('ref_axis',(1.,0.,0.));
#7081=DIRECTION('center_axis',(0.,0.,1.));
#7082=DIRECTION('ref_axis',(1.,0.,0.));
#7083=DIRECTION('center_axis',(0.,0.,1.));
#7084=DIRECTION('ref_axis',(1.,0.,0.));
#7085=DIRECTION('center_axis',(0.,0.,1.));
#7086=DIRECTION('ref_axis',(1.,0.,0.));
#7087=DIRECTION('center_axis',(0.,0.,1.));
#7088=DIRECTION('ref_axis',(1.,0.,0.));
#7089=DIRECTION('center_axis',(0.,0.,1.));
#7090=DIRECTION('ref_axis',(1.,0.,0.));
#7091=DIRECTION('',(0.,0.,-1.));
#7092=DIRECTION('',(0.,0.,-1.));
#7093=DIRECTION('center_axis',(0.,0.,-1.));
#7094=DIRECTION('ref_axis',(-1.,0.,0.));
#7095=DIRECTION('',(0.,0.,-1.));
#7096=DIRECTION('',(0.,0.,-1.));
#7097=DIRECTION('center_axis',(0.,0.,-1.));
#7098=DIRECTION('ref_axis',(-1.,0.,0.));
#7099=DIRECTION('',(0.,0.,-1.));
#7100=DIRECTION('',(0.,0.,-1.));
#7101=DIRECTION('center_axis',(0.,0.,-1.));
#7102=DIRECTION('ref_axis',(-1.,0.,0.));
#7103=DIRECTION('',(0.,0.,-1.));
#7104=DIRECTION('',(0.,0.,-1.));
#7105=DIRECTION('center_axis',(0.,0.,-1.));
#7106=DIRECTION('ref_axis',(-1.,0.,0.));
#7107=DIRECTION('',(0.,0.,-1.));
#7108=DIRECTION('',(0.,0.,-1.));
#7109=DIRECTION('center_axis',(0.,0.,-1.));
#7110=DIRECTION('ref_axis',(-1.,0.,0.));
#7111=DIRECTION('',(0.,0.,-1.));
#7112=DIRECTION('',(0.,0.,-1.));
#7113=DIRECTION('center_axis',(0.,0.,-1.));
#7114=DIRECTION('ref_axis',(-1.,0.,0.));
#7115=DIRECTION('',(0.,0.,-1.));
#7116=DIRECTION('',(0.,0.,-1.));
#7117=DIRECTION('center_axis',(0.,0.,-1.));
#7118=DIRECTION('ref_axis',(-1.,0.,0.));
#7119=DIRECTION('',(0.,0.,-1.));
#7120=DIRECTION('',(0.,0.,-1.));
#7121=DIRECTION('center_axis',(0.,0.,-1.));
#7122=DIRECTION('ref_axis',(-1.,0.,0.));
#7123=DIRECTION('',(0.,0.,-1.));
#7124=DIRECTION('',(0.,0.,-1.));
#7125=DIRECTION('center_axis',(0.,0.,-1.));
#7126=DIRECTION('ref_axis',(-1.,0.,0.));
#7127=DIRECTION('',(0.,0.,-1.));
#7128=DIRECTION('',(0.,0.,-1.));
#7129=DIRECTION('center_axis',(0.,0.,-1.));
#7130=DIRECTION('ref_axis',(-1.,0.,0.));
#7131=DIRECTION('',(0.,0.,-1.));
#7132=DIRECTION('',(0.,0.,-1.));
#7133=DIRECTION('center_axis',(0.,0.,-1.));
#7134=DIRECTION('ref_axis',(-1.,0.,0.));
#7135=DIRECTION('',(0.,0.,-1.));
#7136=DIRECTION('',(0.,0.,-1.));
#7137=DIRECTION('center_axis',(0.,0.,-1.));
#7138=DIRECTION('ref_axis',(-1.,0.,0.));
#7139=DIRECTION('',(0.,0.,-1.));
#7140=DIRECTION('',(0.,0.,-1.));
#7141=DIRECTION('center_axis',(0.,0.,-1.));
#7142=DIRECTION('ref_axis',(-1.,0.,0.));
#7143=DIRECTION('',(0.,0.,-1.));
#7144=DIRECTION('',(0.,0.,-1.));
#7145=DIRECTION('center_axis',(0.,0.,-1.));
#7146=DIRECTION('ref_axis',(-1.,0.,0.));
#7147=DIRECTION('',(0.,0.,-1.));
#7148=DIRECTION('',(0.,0.,-1.));
#7149=DIRECTION('center_axis',(0.,0.,-1.));
#7150=DIRECTION('ref_axis',(-1.,0.,0.));
#7151=DIRECTION('',(0.,0.,-1.));
#7152=DIRECTION('',(0.,0.,-1.));
#7153=DIRECTION('center_axis',(0.,0.,-1.));
#7154=DIRECTION('ref_axis',(-1.,0.,0.));
#7155=DIRECTION('',(0.,0.,-1.));
#7156=DIRECTION('',(0.,0.,-1.));
#7157=DIRECTION('center_axis',(0.,0.,-1.));
#7158=DIRECTION('ref_axis',(-1.,0.,0.));
#7159=DIRECTION('',(0.,0.,-1.));
#7160=DIRECTION('',(0.,0.,-1.));
#7161=DIRECTION('center_axis',(0.,0.,-1.));
#7162=DIRECTION('ref_axis',(-1.,0.,0.));
#7163=DIRECTION('',(0.,0.,-1.));
#7164=DIRECTION('',(0.,0.,-1.));
#7165=DIRECTION('center_axis',(0.,0.,-1.));
#7166=DIRECTION('ref_axis',(-1.,0.,0.));
#7167=DIRECTION('',(0.,0.,-1.));
#7168=DIRECTION('',(0.,0.,-1.));
#7169=DIRECTION('center_axis',(0.,0.,-1.));
#7170=DIRECTION('ref_axis',(-1.,0.,0.));
#7171=DIRECTION('',(0.,0.,-1.));
#7172=DIRECTION('',(0.,0.,-1.));
#7173=DIRECTION('center_axis',(0.,0.,-1.));
#7174=DIRECTION('ref_axis',(-1.,0.,0.));
#7175=DIRECTION('',(0.,0.,-1.));
#7176=DIRECTION('',(0.,0.,-1.));
#7177=DIRECTION('center_axis',(0.,0.,-1.));
#7178=DIRECTION('ref_axis',(-1.,0.,0.));
#7179=DIRECTION('',(0.,0.,-1.));
#7180=DIRECTION('',(0.,0.,-1.));
#7181=DIRECTION('center_axis',(0.,0.,-1.));
#7182=DIRECTION('ref_axis',(-1.,0.,0.));
#7183=DIRECTION('',(0.,0.,-1.));
#7184=DIRECTION('',(0.,0.,-1.));
#7185=DIRECTION('center_axis',(0.,0.,-1.));
#7186=DIRECTION('ref_axis',(-1.,0.,0.));
#7187=DIRECTION('',(0.,0.,-1.));
#7188=DIRECTION('',(0.,0.,-1.));
#7189=DIRECTION('center_axis',(0.,0.,-1.));
#7190=DIRECTION('ref_axis',(-1.,0.,0.));
#7191=DIRECTION('',(0.,0.,-1.));
#7192=DIRECTION('',(0.,0.,-1.));
#7193=DIRECTION('center_axis',(0.,0.,-1.));
#7194=DIRECTION('ref_axis',(-1.,0.,0.));
#7195=DIRECTION('',(0.,0.,-1.));
#7196=DIRECTION('',(0.,0.,-1.));
#7197=DIRECTION('center_axis',(0.,0.,-1.));
#7198=DIRECTION('ref_axis',(-1.,0.,0.));
#7199=DIRECTION('',(0.,0.,-1.));
#7200=DIRECTION('',(0.,0.,-1.));
#7201=DIRECTION('center_axis',(0.,0.,-1.));
#7202=DIRECTION('ref_axis',(-1.,0.,0.));
#7203=DIRECTION('',(0.,0.,-1.));
#7204=DIRECTION('',(0.,0.,-1.));
#7205=DIRECTION('center_axis',(0.,0.,-1.));
#7206=DIRECTION('ref_axis',(-1.,0.,0.));
#7207=DIRECTION('',(0.,0.,-1.));
#7208=DIRECTION('',(0.,0.,-1.));
#7209=DIRECTION('center_axis',(0.,0.,-1.));
#7210=DIRECTION('ref_axis',(-1.,0.,0.));
#7211=DIRECTION('',(0.,0.,-1.));
#7212=DIRECTION('',(0.,0.,-1.));
#7213=DIRECTION('center_axis',(0.,0.,-1.));
#7214=DIRECTION('ref_axis',(-1.,0.,0.));
#7215=DIRECTION('',(0.,0.,-1.));
#7216=DIRECTION('',(0.,0.,-1.));
#7217=DIRECTION('center_axis',(0.,0.,-1.));
#7218=DIRECTION('ref_axis',(-1.,0.,0.));
#7219=DIRECTION('',(0.,0.,-1.));
#7220=DIRECTION('',(0.,0.,-1.));
#7221=DIRECTION('center_axis',(0.,0.,-1.));
#7222=DIRECTION('ref_axis',(-1.,0.,0.));
#7223=DIRECTION('',(0.,0.,-1.));
#7224=DIRECTION('',(0.,0.,-1.));
#7225=DIRECTION('center_axis',(0.,0.,-1.));
#7226=DIRECTION('ref_axis',(-1.,0.,0.));
#7227=DIRECTION('',(0.,0.,-1.));
#7228=DIRECTION('',(0.,0.,-1.));
#7229=DIRECTION('center_axis',(0.,0.,-1.));
#7230=DIRECTION('ref_axis',(-1.,0.,0.));
#7231=DIRECTION('',(0.,0.,-1.));
#7232=DIRECTION('',(0.,0.,-1.));
#7233=DIRECTION('center_axis',(0.,0.,-1.));
#7234=DIRECTION('ref_axis',(-1.,0.,0.));
#7235=DIRECTION('',(0.,0.,-1.));
#7236=DIRECTION('',(0.,0.,-1.));
#7237=DIRECTION('center_axis',(0.,0.,-1.));
#7238=DIRECTION('ref_axis',(1.,-3.21624529935327E-16,0.));
#7239=DIRECTION('',(0.,0.,-1.));
#7240=DIRECTION('',(0.,0.,-1.));
#7241=DIRECTION('center_axis',(0.,0.,-1.));
#7242=DIRECTION('ref_axis',(-1.,0.,0.));
#7243=DIRECTION('',(0.,0.,-1.));
#7244=DIRECTION('',(0.,0.,-1.));
#7245=DIRECTION('center_axis',(0.,0.,-1.));
#7246=DIRECTION('ref_axis',(-1.,0.,0.));
#7247=DIRECTION('center_axis',(0.,0.,1.));
#7248=DIRECTION('ref_axis',(1.,0.,0.));
#7249=DIRECTION('center_axis',(0.,0.,-1.));
#7250=DIRECTION('ref_axis',(-1.,0.,0.));
#8436=CARTESIAN_POINT('',(0.,0.,0.));
#8437=CARTESIAN_POINT('Origin',(0.,0.,1.));
#8438=CARTESIAN_POINT('',(7.,-8.57252759403147E-16,0.));
#8439=CARTESIAN_POINT('Origin',(0.,0.,0.));
#8440=CARTESIAN_POINT('',(7.,-8.57252759403147E-16,1.));
#8441=CARTESIAN_POINT('',(7.,-8.57252759403147E-16,1.));
#8442=CARTESIAN_POINT('Origin',(0.,0.,1.));
#8443=CARTESIAN_POINT('Origin',(0.,0.,1.));
#8444=CARTESIAN_POINT('',(14.,-1.71450551880629E-15,1.));
#8445=CARTESIAN_POINT('Origin',(0.,0.,1.));
#8446=CARTESIAN_POINT('',(14.,-1.71450551880629E-15,0.));
#8447=CARTESIAN_POINT('',(14.,-1.71450551880629E-15,1.));
#8448=CARTESIAN_POINT('Origin',(0.,0.,0.));
#8449=CARTESIAN_POINT('Origin',(0.,0.,6.));
#8450=CARTESIAN_POINT('',(-7.,-8.57252759403147E-16,7.));
#8451=CARTESIAN_POINT('Origin',(0.,0.,7.));
#8452=CARTESIAN_POINT('',(-7.,-8.57252759403147E-16,6.));
#8453=CARTESIAN_POINT('',(-7.,-8.57252759403147E-16,6.));
#8454=CARTESIAN_POINT('Origin',(0.,0.,6.));
#8455=CARTESIAN_POINT('Origin',(0.,0.,6.));
#8456=CARTESIAN_POINT('',(-14.,-1.71450551880629E-15,6.));
#8457=CARTESIAN_POINT('Origin',(0.,0.,6.));
#8458=CARTESIAN_POINT('',(-14.,-1.71450551880629E-15,7.));
#8459=CARTESIAN_POINT('',(-14.,-1.71450551880629E-15,6.));
#8460=CARTESIAN_POINT('Origin',(0.,0.,7.));
#8461=CARTESIAN_POINT('Origin',(0.,-2.16840434497101E-15,7.));
#8462=CARTESIAN_POINT('',(2.5,-2.47456604475785E-15,7.));
#8463=CARTESIAN_POINT('Origin',(0.,-2.16840434497101E-15,7.));
#8464=CARTESIAN_POINT('',(2.5,-2.47456604475785E-15,0.));
#8465=CARTESIAN_POINT('',(2.5,-2.47456604475785E-15,7.));
#8466=CARTESIAN_POINT('Origin',(0.,-2.16840434497101E-15,0.));
#8467=CARTESIAN_POINT('Origin',(0.,0.,7.));
#8468=CARTESIAN_POINT('',(-16.2160625265911,1.04967429885986,7.));
#8469=CARTESIAN_POINT('',(-16.2160625265912,-1.04967429885971,7.));
#8470=CARTESIAN_POINT('Origin',(0.,0.,7.));
#8471=CARTESIAN_POINT('',(-16.2160625265911,1.04967429885986,0.));
#8472=CARTESIAN_POINT('',(-16.2160625265911,1.04967429885986,7.));
#8473=CARTESIAN_POINT('',(-16.2160625265912,-1.04967429885971,0.));
#8474=CARTESIAN_POINT('Origin',(0.,0.,0.));
#8475=CARTESIAN_POINT('',(-16.2160625265912,-1.04967429885971,7.));
#8476=CARTESIAN_POINT('Origin',(16.0675296603332,7.07348467874013,0.));
#8477=CARTESIAN_POINT('Origin',(16.0675296603332,7.07348467874013,7.));
#8478=CARTESIAN_POINT('Origin',(16.0675296603332,7.07348467874013,7.));
#8479=CARTESIAN_POINT('',(15.0980247376579,6.00933848448158,7.));
#8480=CARTESIAN_POINT('',(17.1502563092004,8.17732893607278,7.));
#8481=CARTESIAN_POINT('Ctrl Pts',(15.0980247376579,6.00933848448158,7.));
#8482=CARTESIAN_POINT('Ctrl Pts',(15.0769402326058,6.07637133495396,7.));
#8483=CARTESIAN_POINT('Ctrl Pts',(15.0680440207731,6.1960413432609,7.));
#8484=CARTESIAN_POINT('Ctrl Pts',(15.1168047097502,6.34385243988821,7.));
#8485=CARTESIAN_POINT('Ctrl Pts',(15.1795880240196,6.44397890908497,7.));
#8486=CARTESIAN_POINT('Ctrl Pts',(15.2506809503975,6.52246995302229,7.));
#8487=CARTESIAN_POINT('Ctrl Pts',(15.3282076647862,6.58832104206024,7.));
#8488=CARTESIAN_POINT('Ctrl Pts',(15.3933171197393,6.63306845520277,7.));
#8489=CARTESIAN_POINT('Ctrl Pts',(15.4424051151807,6.66297054550544,7.));
#8490=CARTESIAN_POINT('Ctrl Pts',(15.4733031879166,6.68074830397728,7.));
#8491=CARTESIAN_POINT('Ctrl Pts',(15.5083268912119,6.69953551835471,7.));
#8492=CARTESIAN_POINT('Ctrl Pts',(15.5619248294191,6.72790031412625,7.));
#8493=CARTESIAN_POINT('Ctrl Pts',(15.6387111659832,6.77211692048664,7.));
#8494=CARTESIAN_POINT('Ctrl Pts',(15.7406883947778,6.83570676658069,7.));
#8495=CARTESIAN_POINT('Ctrl Pts',(15.8583036897433,6.91534043556371,7.));
#8496=CARTESIAN_POINT('Ctrl Pts',(15.9905219781863,7.01217619187965,7.));
#8497=CARTESIAN_POINT('Ctrl Pts',(16.1361838672874,7.12742326811382,7.));
#8498=CARTESIAN_POINT('Ctrl Pts',(16.2940809887434,7.2621916599568,7.));
#8499=CARTESIAN_POINT('Ctrl Pts',(16.4629349257385,7.41753779118422,7.));
#8500=CARTESIAN_POINT('Ctrl Pts',(16.6414085620714,7.59444470905136,7.));
#8501=CARTESIAN_POINT('Ctrl Pts',(16.8766905033057,7.84571320523309,7.));
#8502=CARTESIAN_POINT('Ctrl Pts',(17.0448123137865,8.04476736935674,7.));
#8503=CARTESIAN_POINT('Ctrl Pts',(17.1502563092004,8.17732893607278,7.));
#8504=CARTESIAN_POINT('',(16.6962658094608,9.06833546026115,7.));
#8505=CARTESIAN_POINT('Origin',(2.16840434497101E-15,0.,7.));
#8506=CARTESIAN_POINT('',(13.7360532384392,8.6823580570467,7.));
#8507=CARTESIAN_POINT('Ctrl Pts',(16.6962658094608,9.06833546026115,7.));
#8508=CARTESIAN_POINT('Ctrl Pts',(16.5270428237395,9.06094720995301,7.));
#8509=CARTESIAN_POINT('Ctrl Pts',(16.267185101373,9.0419349102283,7.));
#8510=CARTESIAN_POINT('Ctrl Pts',(15.9256093626227,8.9992797377215,7.));
#8511=CARTESIAN_POINT('Ctrl Pts',(15.6775844882862,8.95887481023115,7.));
#8512=CARTESIAN_POINT('Ctrl Pts',(15.4526569741556,8.9135792705712,7.));
#8513=CARTESIAN_POINT('Ctrl Pts',(15.2508174554787,8.86505268915081,7.));
#8514=CARTESIAN_POINT('Ctrl Pts',(15.0719627020186,8.8149502772156,7.));
#8515=CARTESIAN_POINT('Ctrl Pts',(14.9159049694657,8.76490206435509,7.));
#8516=CARTESIAN_POINT('Ctrl Pts',(14.7823474421092,8.71655678814372,7.));
#8517=CARTESIAN_POINT('Ctrl Pts',(14.6709614647943,8.67143265073928,7.));
#8518=CARTESIAN_POINT('Ctrl Pts',(14.5900556026053,8.63530106864818,7.));
#8519=CARTESIAN_POINT('Ctrl Pts',(14.5356039231526,8.60861183441388,7.));
#8520=CARTESIAN_POINT('Ctrl Pts',(14.4998183311667,8.59131991078479,7.));
#8521=CARTESIAN_POINT('Ctrl Pts',(14.4672743909626,8.57677234909658,7.));
#8522=CARTESIAN_POINT('Ctrl Pts',(14.4142298919554,8.55463533425733,7.));
#8523=CARTESIAN_POINT('Ctrl Pts',(14.3397580968625,8.52826254822916,7.));
#8524=CARTESIAN_POINT('Ctrl Pts',(14.2409143873564,8.50424841775457,7.));
#8525=CARTESIAN_POINT('Ctrl Pts',(14.1356264252376,8.49286891019843,7.));
#8526=CARTESIAN_POINT('Ctrl Pts',(14.0177193038531,8.5009290039492,7.));
#8527=CARTESIAN_POINT('Ctrl Pts',(13.8694768008521,8.54836196063209,7.));
#8528=CARTESIAN_POINT('Ctrl Pts',(13.7778907925312,8.62589941321481,7.));
#8529=CARTESIAN_POINT('Ctrl Pts',(13.7360532384392,8.6823580570467,7.));
#8530=CARTESIAN_POINT('',(12.5020870932787,10.3807667497191,7.));
#8531=CARTESIAN_POINT('Origin',(0.,0.,7.));
#8532=CARTESIAN_POINT('',(13.7839294091566,13.07682262797,7.));
#8533=CARTESIAN_POINT('Ctrl Pts',(12.5020870932787,10.3807667497191,7.));
#8534=CARTESIAN_POINT('Ctrl Pts',(12.4613202473788,10.4380033085876,7.));
#8535=CARTESIAN_POINT('Ctrl Pts',(12.4158793808611,10.5490671691512,7.));
#8536=CARTESIAN_POINT('Ctrl Pts',(12.4165774110367,10.7047117573306,7.));
#8537=CARTESIAN_POINT('Ctrl Pts',(12.4453471106188,10.8193387993863,7.));
#8538=CARTESIAN_POINT('Ctrl Pts',(12.48870543503,10.9159571406243,7.));
#8539=CARTESIAN_POINT('Ctrl Pts',(12.5420886163255,11.0025423202231,7.));
#8540=CARTESIAN_POINT('Ctrl Pts',(12.5901836766158,11.0652195671547,7.));
#8541=CARTESIAN_POINT('Ctrl Pts',(12.6276288804813,11.1088271697991,7.));
#8542=CARTESIAN_POINT('Ctrl Pts',(12.651521064408,11.1352828524077,7.));
#8543=CARTESIAN_POINT('Ctrl Pts',(12.6790250171322,11.1639734745885,7.));
#8544=CARTESIAN_POINT('Ctrl Pts',(12.7212344815888,11.2075126722099,7.));
#8545=CARTESIAN_POINT('Ctrl Pts',(12.7805989445416,11.2732934467515,7.));
#8546=CARTESIAN_POINT('Ctrl Pts',(12.8579347093876,11.3652836809863,7.));
#8547=CARTESIAN_POINT('Ctrl Pts',(12.9451853450404,11.4773649257318,7.));
#8548=CARTESIAN_POINT('Ctrl Pts',(13.0410085154727,11.6103189008825,7.));
#8549=CARTESIAN_POINT('Ctrl Pts',(13.1439278991698,11.764937382884,7.));
#8550=CARTESIAN_POINT('Ctrl Pts',(13.2524512620507,11.9419026340297,7.));
#8551=CARTESIAN_POINT('Ctrl Pts',(13.3650363045724,12.1418243205134,7.));
#8552=CARTESIAN_POINT('Ctrl Pts',(13.4801075753502,12.3652241842034,7.));
#8553=CARTESIAN_POINT('Ctrl Pts',(13.6262277632565,12.6769008431476,7.));
#8554=CARTESIAN_POINT('Ctrl Pts',(13.7246099871303,12.9181650995967,7.));
#8555=CARTESIAN_POINT('Ctrl Pts',(13.7839294091566,13.07682262797,7.));
#8556=CARTESIAN_POINT('',(13.07682262797,13.7839294091566,7.));
#8557=CARTESIAN_POINT('Origin',(0.,0.,7.));
#8558=CARTESIAN_POINT('',(10.3807667497191,12.5020870932787,7.));
#8559=CARTESIAN_POINT('Ctrl Pts',(13.07682262797,13.7839294091566,7.));
#8560=CARTESIAN_POINT('Ctrl Pts',(12.9181650995967,13.7246099871302,7.));
#8561=CARTESIAN_POINT('Ctrl Pts',(12.6769008431476,13.6262277632565,7.));
#8562=CARTESIAN_POINT('Ctrl Pts',(12.3652241842033,13.4801075753502,7.));
#8563=CARTESIAN_POINT('Ctrl Pts',(12.1418243205134,13.3650363045723,7.));
#8564=CARTESIAN_POINT('Ctrl Pts',(11.9419026340297,13.2524512620508,7.));
#8565=CARTESIAN_POINT('Ctrl Pts',(11.764937382884,13.1439278991698,7.));
#8566=CARTESIAN_POINT('Ctrl Pts',(11.6103189008825,13.0410085154728,7.));
#8567=CARTESIAN_POINT('Ctrl Pts',(11.4773649257318,12.9451853450404,7.));
#8568=CARTESIAN_POINT('Ctrl Pts',(11.3652836809863,12.8579347093876,7.));
#8569=CARTESIAN_POINT('Ctrl Pts',(11.2732934467515,12.7805989445416,7.));
#8570=CARTESIAN_POINT('Ctrl Pts',(11.2075126722099,12.7212344815888,7.));
#8571=CARTESIAN_POINT('Ctrl Pts',(11.1639734745885,12.6790250171322,7.));
#8572=CARTESIAN_POINT('Ctrl Pts',(11.1352828524076,12.6515210644081,7.));
#8573=CARTESIAN_POINT('Ctrl Pts',(11.108827169799,12.6276288804813,7.));
#8574=CARTESIAN_POINT('Ctrl Pts',(11.0652195671547,12.5901836766158,7.));
#8575=CARTESIAN_POINT('Ctrl Pts',(11.0025423202231,12.5420886163255,7.));
#8576=CARTESIAN_POINT('Ctrl Pts',(10.9159571406242,12.48870543503,7.));
#8577=CARTESIAN_POINT('Ctrl Pts',(10.8193387993863,12.4453471106187,7.));
#8578=CARTESIAN_POINT('Ctrl Pts',(10.7047117573306,12.4165774110367,7.));
#8579=CARTESIAN_POINT('Ctrl Pts',(10.5490671691512,12.4158793808611,7.));
#8580=CARTESIAN_POINT('Ctrl Pts',(10.4380033085876,12.4613202473787,7.));
#8581=CARTESIAN_POINT('Ctrl Pts',(10.3807667497191,12.5020870932787,7.));
#8582=CARTESIAN_POINT('',(8.68235805704686,13.7360532384391,7.));
#8583=CARTESIAN_POINT('Origin',(0.,0.,7.));
#8584=CARTESIAN_POINT('',(9.06833546026116,16.6962658094608,7.));
#8585=CARTESIAN_POINT('Ctrl Pts',(8.68235805704686,13.7360532384391,7.));
#8586=CARTESIAN_POINT('Ctrl Pts',(8.62589941321482,13.7778907925313,7.));
#8587=CARTESIAN_POINT('Ctrl Pts',(8.54836196063209,13.8694768008521,7.));
#8588=CARTESIAN_POINT('Ctrl Pts',(8.50092900394922,14.0177193038531,7.));
#8589=CARTESIAN_POINT('Ctrl Pts',(8.49286891019844,14.1356264252377,7.));
#8590=CARTESIAN_POINT('Ctrl Pts',(8.50424841775457,14.2409143873564,7.));
#8591=CARTESIAN_POINT('Ctrl Pts',(8.52826254822916,14.3397580968626,7.));
#8592=CARTESIAN_POINT('Ctrl Pts',(8.55463533425733,14.4142298919554,7.));
#8593=CARTESIAN_POINT('Ctrl Pts',(8.57677234909656,14.4672743909627,7.));
#8594=CARTESIAN_POINT('Ctrl Pts',(8.59131991078476,14.4998183311667,7.));
#8595=CARTESIAN_POINT('Ctrl Pts',(8.6086118344139,14.5356039231527,7.));
#8596=CARTESIAN_POINT('Ctrl Pts',(8.63530106864819,14.5900556026053,7.));
#8597=CARTESIAN_POINT('Ctrl Pts',(8.67143265073928,14.6709614647944,7.));
#8598=CARTESIAN_POINT('Ctrl Pts',(8.71655678814373,14.7823474421093,7.));
#8599=CARTESIAN_POINT('Ctrl Pts',(8.76490206435509,14.9159049694657,7.));
#8600=CARTESIAN_POINT('Ctrl Pts',(8.81495027721557,15.0719627020186,7.));
#8601=CARTESIAN_POINT('Ctrl Pts',(8.86505268915084,15.2508174554788,7.));
#8602=CARTESIAN_POINT('Ctrl Pts',(8.91357927057117,15.4526569741556,7.));
#8603=CARTESIAN_POINT('Ctrl Pts',(8.95887481023115,15.6775844882862,7.));
#8604=CARTESIAN_POINT('Ctrl Pts',(8.99927973772153,15.9256093626227,7.));
#8605=CARTESIAN_POINT('Ctrl Pts',(9.04193491022831,16.2671851013731,7.));
#8606=CARTESIAN_POINT('Ctrl Pts',(9.06094720995305,16.5270428237395,7.));
#8607=CARTESIAN_POINT('Ctrl Pts',(9.06833546026116,16.6962658094608,7.));
#8608=CARTESIAN_POINT('',(8.17732893607301,17.1502563092002,7.));
#8609=CARTESIAN_POINT('Origin',(0.,-2.16840434497101E-15,7.));
#8610=CARTESIAN_POINT('',(6.00933848448158,15.0980247376579,7.));
#8611=CARTESIAN_POINT('Ctrl Pts',(8.17732893607301,17.1502563092002,7.));
#8612=CARTESIAN_POINT('Ctrl Pts',(8.04476736935673,17.0448123137865,7.));
#8613=CARTESIAN_POINT('Ctrl Pts',(7.84571320523309,16.8766905033057,7.));
#8614=CARTESIAN_POINT('Ctrl Pts',(7.59444470905135,16.6414085620714,7.));
#8615=CARTESIAN_POINT('Ctrl Pts',(7.4175377911842,16.4629349257385,7.));
#8616=CARTESIAN_POINT('Ctrl Pts',(7.26219165995678,16.2940809887434,7.));
#8617=CARTESIAN_POINT('Ctrl Pts',(7.12742326811382,16.1361838672874,7.));
#8618=CARTESIAN_POINT('Ctrl Pts',(7.01217619187961,15.9905219781863,7.));
#8619=CARTESIAN_POINT('Ctrl Pts',(6.91534043556368,15.8583036897433,7.));
#8620=CARTESIAN_POINT('Ctrl Pts',(6.83570676658068,15.7406883947777,7.));
#8621=CARTESIAN_POINT('Ctrl Pts',(6.77211692048662,15.6387111659832,7.));
#8622=CARTESIAN_POINT('Ctrl Pts',(6.72790031412623,15.5619248294191,7.));
#8623=CARTESIAN_POINT('Ctrl Pts',(6.69953551835472,15.5083268912119,7.));
#8624=CARTESIAN_POINT('Ctrl Pts',(6.68074830397725,15.4733031879166,7.));
#8625=CARTESIAN_POINT('Ctrl Pts',(6.66297054550541,15.4424051151807,7.));
#8626=CARTESIAN_POINT('Ctrl Pts',(6.63306845520275,15.3933171197393,7.));
#8627=CARTESIAN_POINT('Ctrl Pts',(6.58832104206022,15.3282076647862,7.));
#8628=CARTESIAN_POINT('Ctrl Pts',(6.52246995302225,15.2506809503975,7.));
#8629=CARTESIAN_POINT('Ctrl Pts',(6.44397890908495,15.1795880240196,7.));
#8630=CARTESIAN_POINT('Ctrl Pts',(6.34385243988822,15.1168047097501,7.));
#8631=CARTESIAN_POINT('Ctrl Pts',(6.19604134326089,15.0680440207731,7.));
#8632=CARTESIAN_POINT('Ctrl Pts',(6.07637133495393,15.0769402326058,7.));
#8633=CARTESIAN_POINT('Ctrl Pts',(6.00933848448158,15.0980247376579,7.));
#8634=CARTESIAN_POINT('',(4.01273932064543,15.7467591314704,7.));
#8635=CARTESIAN_POINT('Origin',(0.,0.,7.));
#8636=CARTESIAN_POINT('',(3.46506965370702,18.6813621637974,7.));
#8637=CARTESIAN_POINT('Ctrl Pts',(4.01273932064543,15.7467591314704,7.));
#8638=CARTESIAN_POINT('Ctrl Pts',(3.94611544431017,15.7691023294921,7.));
#8639=CARTESIAN_POINT('Ctrl Pts',(3.84407131175635,15.8322454089585,7.));
#8640=CARTESIAN_POINT('Ctrl Pts',(3.75315043649997,15.9585748177211,7.));
#8641=CARTESIAN_POINT('Ctrl Pts',(3.70904952755068,16.0682204478862,7.));
#8642=CARTESIAN_POINT('Ctrl Pts',(3.68733631276637,16.1718717115691,7.));
#8643=CARTESIAN_POINT('Ctrl Pts',(3.67963072201293,16.2732984400116,7.));
#8644=CARTESIAN_POINT('Ctrl Pts',(3.68169968173257,16.3522749650866,7.));
#8645=CARTESIAN_POINT('Ctrl Pts',(3.68636158229542,16.409563995311,7.));
#8646=CARTESIAN_POINT('Ctrl Pts',(3.69014050504822,16.4450105654964,7.));
#8647=CARTESIAN_POINT('Ctrl Pts',(3.69552774561756,16.4843881842109,7.));
#8648=CARTESIAN_POINT('Ctrl Pts',(3.70408422142788,16.5444222357228,7.));
#8649=CARTESIAN_POINT('Ctrl Pts',(3.71344611165869,16.632533556064,7.));
#8650=CARTESIAN_POINT('Ctrl Pts',(3.72194155665403,16.7524120409277,7.));
#8651=CARTESIAN_POINT('Ctrl Pts',(3.7266491009471,16.8943723095674,7.));
#8652=CARTESIAN_POINT('Ctrl Pts',(3.72602328845452,17.0582577813421,7.));
#8653=CARTESIAN_POINT('Ctrl Pts',(3.71840435546373,17.2438412568379,7.));
#8654=CARTESIAN_POINT('Ctrl Pts',(3.70218403552947,17.4507975846592,7.));
#8655=CARTESIAN_POINT('Ctrl Pts',(3.67575622931333,17.6787134541915,7.));
#8656=CARTESIAN_POINT('Ctrl Pts',(3.63753969769581,17.9270849363835,7.));
#8657=CARTESIAN_POINT('Ctrl Pts',(3.57255446932205,18.265123941733,7.));
#8658=CARTESIAN_POINT('Ctrl Pts',(3.51033578853423,18.5181384456163,7.));
#8659=CARTESIAN_POINT('Ctrl Pts',(3.46506965370702,18.6813621637974,7.));
#8660=CARTESIAN_POINT('',(2.47738131311212,18.8377966288375,7.));
#8661=CARTESIAN_POINT('Origin',(0.,8.67361737988404E-16,7.));
#8662=CARTESIAN_POINT('',(1.04967429885989,16.2160625265911,7.));
#8663=CARTESIAN_POINT('Ctrl Pts',(2.47738131311212,18.8377966288375,7.));
#8664=CARTESIAN_POINT('Ctrl Pts',(2.38389175781397,18.6965496529788,7.));
#8665=CARTESIAN_POINT('Ctrl Pts',(2.24653249449213,18.4751451900744,7.));
#8666=CARTESIAN_POINT('Ctrl Pts',(2.08026807216976,18.1737325312257,7.));
#8667=CARTESIAN_POINT('Ctrl Pts',(1.96717098182927,17.949326772361,7.));
#8668=CARTESIAN_POINT('Ctrl Pts',(1.87160676754279,17.7407325407201,7.));
#8669=CARTESIAN_POINT('Ctrl Pts',(1.79222730418274,17.548917731071,7.));
#8670=CARTESIAN_POINT('Ctrl Pts',(1.72763282051121,17.3747717371572,7.));
#8671=CARTESIAN_POINT('Ctrl Pts',(1.67639424155266,17.2191007779952,7.));
#8672=CARTESIAN_POINT('Ctrl Pts',(1.63700324669265,17.0826338282621,7.));
#8673=CARTESIAN_POINT('Ctrl Pts',(1.60803840593148,16.9659973771906,7.));
#8674=CARTESIAN_POINT('Ctrl Pts',(1.58971419725808,16.8793055486399,7.));
#8675=CARTESIAN_POINT('Ctrl Pts',(1.57930034717568,16.8195656763126,7.));
#8676=CARTESIAN_POINT('Ctrl Pts',(1.57225556404314,16.7804505865492,7.));
#8677=CARTESIAN_POINT('Ctrl Pts',(1.5648959405722,16.7455711436431,7.));
#8678=CARTESIAN_POINT('Ctrl Pts',(1.5516263875502,16.6896454316358,7.));
#8679=CARTESIAN_POINT('Ctrl Pts',(1.52918899676866,16.6138949491149,7.));
#8680=CARTESIAN_POINT('Ctrl Pts',(1.49051796169813,16.5198135565977,7.));
#8681=CARTESIAN_POINT('Ctrl Pts',(1.43783746532136,16.4279450992207,7.));
#8682=CARTESIAN_POINT('Ctrl Pts',(1.36201264541063,16.3372938385016,7.));
#8683=CARTESIAN_POINT('Ctrl Pts',(1.23650382033381,16.2452435266959,7.));
#8684=CARTESIAN_POINT('Ctrl Pts',(1.11994179848653,16.2167242606458,7.));
#8685=CARTESIAN_POINT('Ctrl Pts',(1.04967429885989,16.2160625265911,7.));
#8686=CARTESIAN_POINT('',(-1.04967429885962,16.2160625265911,7.));
#8687=CARTESIAN_POINT('Origin',(0.,0.,7.));
#8688=CARTESIAN_POINT('',(-2.47738131311187,18.8377966288376,7.));
#8689=CARTESIAN_POINT('Ctrl Pts',(-1.04967429885962,16.2160625265911,7.));
#8690=CARTESIAN_POINT('Ctrl Pts',(-1.11994179848651,16.2167242606459,7.));
#8691=CARTESIAN_POINT('Ctrl Pts',(-1.23650382033378,16.2452435266959,7.));
#8692=CARTESIAN_POINT('Ctrl Pts',(-1.36201264541058,16.3372938385016,7.));
#8693=CARTESIAN_POINT('Ctrl Pts',(-1.43783746532133,16.4279450992208,7.));
#8694=CARTESIAN_POINT('Ctrl Pts',(-1.49051796169812,16.5198135565978,7.));
#8695=CARTESIAN_POINT('Ctrl Pts',(-1.52918899676864,16.6138949491149,7.));
#8696=CARTESIAN_POINT('Ctrl Pts',(-1.55162638755018,16.6896454316359,7.));
#8697=CARTESIAN_POINT('Ctrl Pts',(-1.5648959405722,16.7455711436431,7.));
#8698=CARTESIAN_POINT('Ctrl Pts',(-1.57225556404314,16.7804505865492,7.));
#8699=CARTESIAN_POINT('Ctrl Pts',(-1.57930034717564,16.8195656763126,7.));
#8700=CARTESIAN_POINT('Ctrl Pts',(-1.58971419725806,16.8793055486399,7.));
#8701=CARTESIAN_POINT('Ctrl Pts',(-1.60803840593146,16.9659973771906,7.));
#8702=CARTESIAN_POINT('Ctrl Pts',(-1.63700324669262,17.0826338282622,7.));
#8703=CARTESIAN_POINT('Ctrl Pts',(-1.67639424155265,17.2191007779953,7.));
#8704=CARTESIAN_POINT('Ctrl Pts',(-1.72763282051122,17.3747717371572,7.));
#8705=CARTESIAN_POINT('Ctrl Pts',(-1.7922273041827,17.548917731071,7.));
#8706=CARTESIAN_POINT('Ctrl Pts',(-1.87160676754278,17.7407325407201,7.));
#8707=CARTESIAN_POINT('Ctrl Pts',(-1.96717098182926,17.949326772361,7.));
#8708=CARTESIAN_POINT('Ctrl Pts',(-2.08026807216973,18.1737325312257,7.));
#8709=CARTESIAN_POINT('Ctrl Pts',(-2.24653249449211,18.4751451900744,7.));
#8710=CARTESIAN_POINT('Ctrl Pts',(-2.38389175781394,18.6965496529788,7.));
#8711=CARTESIAN_POINT('Ctrl Pts',(-2.47738131311187,18.8377966288376,7.));
#8712=CARTESIAN_POINT('',(-3.46506965370679,18.6813621637974,7.));
#8713=CARTESIAN_POINT('Origin',(-1.73472347597681E-15,0.,7.));
#8714=CARTESIAN_POINT('',(-4.01273932064518,15.7467591314705,7.));
#8715=CARTESIAN_POINT('Ctrl Pts',(-3.46506965370679,18.6813621637974,7.));
#8716=CARTESIAN_POINT('Ctrl Pts',(-3.51033578853418,18.5181384456162,7.));
#8717=CARTESIAN_POINT('Ctrl Pts',(-3.57255446932203,18.265123941733,7.));
#8718=CARTESIAN_POINT('Ctrl Pts',(-3.63753969769577,17.9270849363835,7.));
#8719=CARTESIAN_POINT('Ctrl Pts',(-3.67575622931332,17.6787134541915,7.));
#8720=CARTESIAN_POINT('Ctrl Pts',(-3.70218403552948,17.4507975846592,7.));
#8721=CARTESIAN_POINT('Ctrl Pts',(-3.7184043554637,17.2438412568379,7.));
#8722=CARTESIAN_POINT('Ctrl Pts',(-3.72602328845454,17.0582577813421,7.));
#8723=CARTESIAN_POINT('Ctrl Pts',(-3.72664910094709,16.8943723095674,7.));
#8724=CARTESIAN_POINT('Ctrl Pts',(-3.72194155665401,16.7524120409277,7.));
#8725=CARTESIAN_POINT('Ctrl Pts',(-3.71344611165868,16.632533556064,7.));
#8726=CARTESIAN_POINT('Ctrl Pts',(-3.70408422142788,16.5444222357228,7.));
#8727=CARTESIAN_POINT('Ctrl Pts',(-3.69552774561753,16.4843881842109,7.));
#8728=CARTESIAN_POINT('Ctrl Pts',(-3.69014050504823,16.4450105654964,7.));
#8729=CARTESIAN_POINT('Ctrl Pts',(-3.68636158229542,16.409563995311,7.));
#8730=CARTESIAN_POINT('Ctrl Pts',(-3.68169968173256,16.3522749650865,7.));
#8731=CARTESIAN_POINT('Ctrl Pts',(-3.67963072201293,16.2732984400115,7.));
#8732=CARTESIAN_POINT('Ctrl Pts',(-3.68733631276638,16.1718717115691,7.));
#8733=CARTESIAN_POINT('Ctrl Pts',(-3.70904952755066,16.0682204478862,7.));
#8734=CARTESIAN_POINT('Ctrl Pts',(-3.75315043649994,15.958574817721,7.));
#8735=CARTESIAN_POINT('Ctrl Pts',(-3.84407131175633,15.8322454089585,7.));
#8736=CARTESIAN_POINT('Ctrl Pts',(-3.94611544431016,15.7691023294921,7.));
#8737=CARTESIAN_POINT('Ctrl Pts',(-4.01273932064518,15.7467591314705,7.));
#8738=CARTESIAN_POINT('',(-6.00933848448141,15.0980247376579,7.));
#8739=CARTESIAN_POINT('Origin',(0.,0.,7.));
#8740=CARTESIAN_POINT('',(-8.1773289360728,17.1502563092004,7.));
#8741=CARTESIAN_POINT('Ctrl Pts',(-6.00933848448141,15.0980247376579,7.));
#8742=CARTESIAN_POINT('Ctrl Pts',(-6.076371334954,15.0769402326058,7.));
#8743=CARTESIAN_POINT('Ctrl Pts',(-6.19604134326094,15.0680440207731,7.));
#8744=CARTESIAN_POINT('Ctrl Pts',(-6.34385243988825,15.1168047097501,7.));
#8745=CARTESIAN_POINT('Ctrl Pts',(-6.44397890908501,15.1795880240196,7.));
#8746=CARTESIAN_POINT('Ctrl Pts',(-6.52246995302233,15.2506809503975,7.));
#8747=CARTESIAN_POINT('Ctrl Pts',(-6.58832104206028,15.3282076647862,7.));
#8748=CARTESIAN_POINT('Ctrl Pts',(-6.63306845520281,15.3933171197393,7.));
#8749=CARTESIAN_POINT('Ctrl Pts',(-6.66297054550547,15.4424051151807,7.));
#8750=CARTESIAN_POINT('Ctrl Pts',(-6.68074830397731,15.4733031879166,7.));
#8751=CARTESIAN_POINT('Ctrl Pts',(-6.69953551835474,15.5083268912119,7.));
#8752=CARTESIAN_POINT('Ctrl Pts',(-6.72790031412628,15.5619248294191,7.));
#8753=CARTESIAN_POINT('Ctrl Pts',(-6.77211692048667,15.6387111659832,7.));
#8754=CARTESIAN_POINT('Ctrl Pts',(-6.83570676658072,15.7406883947778,7.));
#8755=CARTESIAN_POINT('Ctrl Pts',(-6.91534043556374,15.8583036897433,7.));
#8756=CARTESIAN_POINT('Ctrl Pts',(-7.01217619187967,15.9905219781863,7.));
#8757=CARTESIAN_POINT('Ctrl Pts',(-7.12742326811385,16.1361838672874,7.));
#8758=CARTESIAN_POINT('Ctrl Pts',(-7.26219165995682,16.2940809887434,7.));
#8759=CARTESIAN_POINT('Ctrl Pts',(-7.41753779118424,16.4629349257385,7.));
#8760=CARTESIAN_POINT('Ctrl Pts',(-7.59444470905137,16.6414085620714,7.));
#8761=CARTESIAN_POINT('Ctrl Pts',(-7.8457132052331,16.8766905033058,7.));
#8762=CARTESIAN_POINT('Ctrl Pts',(-8.04476736935674,17.0448123137865,7.));
#8763=CARTESIAN_POINT('Ctrl Pts',(-8.1773289360728,17.1502563092004,7.));
#8764=CARTESIAN_POINT('',(-9.06833546026097,16.6962658094609,7.));
#8765=CARTESIAN_POINT('Origin',(1.73472347597681E-15,0.,7.));
#8766=CARTESIAN_POINT('',(-8.68235805704666,13.7360532384392,7.));
#8767=CARTESIAN_POINT('Ctrl Pts',(-9.06833546026097,16.6962658094609,7.));
#8768=CARTESIAN_POINT('Ctrl Pts',(-9.06094720995302,16.5270428237395,7.));
#8769=CARTESIAN_POINT('Ctrl Pts',(-9.04193491022831,16.2671851013731,7.));
#8770=CARTESIAN_POINT('Ctrl Pts',(-8.9992797377215,15.9256093626227,7.));
#8771=CARTESIAN_POINT('Ctrl Pts',(-8.95887481023115,15.6775844882862,7.));
#8772=CARTESIAN_POINT('Ctrl Pts',(-8.91357927057119,15.4526569741556,7.));
#8773=CARTESIAN_POINT('Ctrl Pts',(-8.8650526891508,15.2508174554788,7.));
#8774=CARTESIAN_POINT('Ctrl Pts',(-8.81495027721559,15.0719627020186,7.));
#8775=CARTESIAN_POINT('Ctrl Pts',(-8.76490206435507,14.9159049694657,7.));
#8776=CARTESIAN_POINT('Ctrl Pts',(-8.71655678814369,14.7823474421093,7.));
#8777=CARTESIAN_POINT('Ctrl Pts',(-8.67143265073926,14.6709614647944,7.));
#8778=CARTESIAN_POINT('Ctrl Pts',(-8.63530106864816,14.5900556026053,7.));
#8779=CARTESIAN_POINT('Ctrl Pts',(-8.60861183441386,14.5356039231527,7.));
#8780=CARTESIAN_POINT('Ctrl Pts',(-8.59131991078476,14.4998183311667,7.));
#8781=CARTESIAN_POINT('Ctrl Pts',(-8.57677234909655,14.4672743909627,7.));
#8782=CARTESIAN_POINT('Ctrl Pts',(-8.55463533425729,14.4142298919554,7.));
#8783=CARTESIAN_POINT('Ctrl Pts',(-8.52826254822913,14.3397580968626,7.));
#8784=CARTESIAN_POINT('Ctrl Pts',(-8.50424841775454,14.2409143873564,7.));
#8785=CARTESIAN_POINT('Ctrl Pts',(-8.49286891019839,14.1356264252377,7.));
#8786=CARTESIAN_POINT('Ctrl Pts',(-8.50092900394916,14.0177193038531,7.));
#8787=CARTESIAN_POINT('Ctrl Pts',(-8.54836196063204,13.8694768008521,7.));
#8788=CARTESIAN_POINT('Ctrl Pts',(-8.62589941321477,13.7778907925313,7.));
#8789=CARTESIAN_POINT('Ctrl Pts',(-8.68235805704666,13.7360532384392,7.));
#8790=CARTESIAN_POINT('',(-10.380766749719,12.5020870932788,7.));
#8791=CARTESIAN_POINT('Origin',(0.,0.,7.));
#8792=CARTESIAN_POINT('',(-13.07682262797,13.7839294091566,7.));
#8793=CARTESIAN_POINT('Ctrl Pts',(-10.380766749719,12.5020870932788,7.));
#8794=CARTESIAN_POINT('Ctrl Pts',(-10.4380033085876,12.4613202473787,7.));
#8795=CARTESIAN_POINT('Ctrl Pts',(-10.5490671691512,12.4158793808611,7.));
#8796=CARTESIAN_POINT('Ctrl Pts',(-10.7047117573307,12.4165774110367,7.));
#8797=CARTESIAN_POINT('Ctrl Pts',(-10.8193387993863,12.4453471106187,7.));
#8798=CARTESIAN_POINT('Ctrl Pts',(-10.9159571406243,12.48870543503,7.));
#8799=CARTESIAN_POINT('Ctrl Pts',(-11.0025423202232,12.5420886163255,7.));
#8800=CARTESIAN_POINT('Ctrl Pts',(-11.0652195671547,12.5901836766158,7.));
#8801=CARTESIAN_POINT('Ctrl Pts',(-11.1088271697991,12.6276288804813,7.));
#8802=CARTESIAN_POINT('Ctrl Pts',(-11.1352828524077,12.651521064408,7.));
#8803=CARTESIAN_POINT('Ctrl Pts',(-11.1639734745886,12.6790250171322,7.));
#8804=CARTESIAN_POINT('Ctrl Pts',(-11.20751267221,12.7212344815888,7.));
#8805=CARTESIAN_POINT('Ctrl Pts',(-11.2732934467516,12.7805989445416,7.));
#8806=CARTESIAN_POINT('Ctrl Pts',(-11.3652836809863,12.8579347093876,7.));
#8807=CARTESIAN_POINT('Ctrl Pts',(-11.4773649257319,12.9451853450404,7.));
#8808=CARTESIAN_POINT('Ctrl Pts',(-11.6103189008826,13.0410085154727,7.));
#8809=CARTESIAN_POINT('Ctrl Pts',(-11.764937382884,13.1439278991698,7.));
#8810=CARTESIAN_POINT('Ctrl Pts',(-11.9419026340297,13.2524512620507,7.));
#8811=CARTESIAN_POINT('Ctrl Pts',(-12.1418243205134,13.3650363045724,7.));
#8812=CARTESIAN_POINT('Ctrl Pts',(-12.3652241842034,13.4801075753502,7.));
#8813=CARTESIAN_POINT('Ctrl Pts',(-12.6769008431476,13.6262277632565,7.));
#8814=CARTESIAN_POINT('Ctrl Pts',(-12.9181650995968,13.7246099871303,7.));
#8815=CARTESIAN_POINT('Ctrl Pts',(-13.07682262797,13.7839294091566,7.));
#8816=CARTESIAN_POINT('',(-13.7839294091564,13.0768226279702,7.));
#8817=CARTESIAN_POINT('Origin',(1.57723797680727E-16,0.,7.));
#8818=CARTESIAN_POINT('',(-12.5020870932787,10.3807667497191,7.));
#8819=CARTESIAN_POINT('Ctrl Pts',(-13.7839294091564,13.0768226279702,7.));
#8820=CARTESIAN_POINT('Ctrl Pts',(-13.7246099871302,12.9181650995968,7.));
#8821=CARTESIAN_POINT('Ctrl Pts',(-13.6262277632565,12.6769008431476,7.));
#8822=CARTESIAN_POINT('Ctrl Pts',(-13.4801075753502,12.3652241842034,7.));
#8823=CARTESIAN_POINT('Ctrl Pts',(-13.3650363045723,12.1418243205134,7.));
#8824=CARTESIAN_POINT('Ctrl Pts',(-13.2524512620508,11.9419026340297,7.));
#8825=CARTESIAN_POINT('Ctrl Pts',(-13.1439278991698,11.764937382884,7.));
#8826=CARTESIAN_POINT('Ctrl Pts',(-13.0410085154728,11.6103189008826,7.));
#8827=CARTESIAN_POINT('Ctrl Pts',(-12.9451853450404,11.4773649257318,7.));
#8828=CARTESIAN_POINT('Ctrl Pts',(-12.8579347093876,11.3652836809863,7.));
#8829=CARTESIAN_POINT('Ctrl Pts',(-12.7805989445416,11.2732934467516,7.));
#8830=CARTESIAN_POINT('Ctrl Pts',(-12.7212344815888,11.2075126722099,7.));
#8831=CARTESIAN_POINT('Ctrl Pts',(-12.6790250171322,11.1639734745886,7.));
#8832=CARTESIAN_POINT('Ctrl Pts',(-12.651521064408,11.1352828524077,7.));
#8833=CARTESIAN_POINT('Ctrl Pts',(-12.6276288804813,11.1088271697991,7.));
#8834=CARTESIAN_POINT('Ctrl Pts',(-12.5901836766158,11.0652195671547,7.));
#8835=CARTESIAN_POINT('Ctrl Pts',(-12.5420886163255,11.0025423202231,7.));
#8836=CARTESIAN_POINT('Ctrl Pts',(-12.48870543503,10.9159571406243,7.));
#8837=CARTESIAN_POINT('Ctrl Pts',(-12.4453471106187,10.8193387993863,7.));
#8838=CARTESIAN_POINT('Ctrl Pts',(-12.4165774110367,10.7047117573307,7.));
#8839=CARTESIAN_POINT('Ctrl Pts',(-12.4158793808611,10.5490671691512,7.));
#8840=CARTESIAN_POINT('Ctrl Pts',(-12.4613202473787,10.4380033085876,7.));
#8841=CARTESIAN_POINT('Ctrl Pts',(-12.5020870932787,10.3807667497191,7.));
#8842=CARTESIAN_POINT('',(-13.7360532384391,8.68235805704682,7.));
#8843=CARTESIAN_POINT('Origin',(0.,0.,7.));
#8844=CARTESIAN_POINT('',(-16.6962658094608,9.06833546026117,7.));
#8845=CARTESIAN_POINT('Ctrl Pts',(-13.7360532384391,8.68235805704682,7.));
#8846=CARTESIAN_POINT('Ctrl Pts',(-13.7778907925313,8.62589941321479,7.));
#8847=CARTESIAN_POINT('Ctrl Pts',(-13.8694768008521,8.54836196063206,7.));
#8848=CARTESIAN_POINT('Ctrl Pts',(-14.0177193038531,8.50092900394919,7.));
#8849=CARTESIAN_POINT('Ctrl Pts',(-14.1356264252377,8.49286891019842,7.));
#8850=CARTESIAN_POINT('Ctrl Pts',(-14.2409143873564,8.50424841775455,7.));
#8851=CARTESIAN_POINT('Ctrl Pts',(-14.3397580968626,8.52826254822914,7.));
#8852=CARTESIAN_POINT('Ctrl Pts',(-14.4142298919555,8.55463533425731,7.));
#8853=CARTESIAN_POINT('Ctrl Pts',(-14.4672743909627,8.57677234909655,7.));
#8854=CARTESIAN_POINT('Ctrl Pts',(-14.4998183311667,8.59131991078475,7.));
#8855=CARTESIAN_POINT('Ctrl Pts',(-14.5356039231527,8.60861183441388,7.));
#8856=CARTESIAN_POINT('Ctrl Pts',(-14.5900556026053,8.63530106864817,7.));
#8857=CARTESIAN_POINT('Ctrl Pts',(-14.6709614647944,8.67143265073926,7.));
#8858=CARTESIAN_POINT('Ctrl Pts',(-14.7823474421093,8.71655678814371,7.));
#8859=CARTESIAN_POINT('Ctrl Pts',(-14.9159049694657,8.76490206435508,7.));
#8860=CARTESIAN_POINT('Ctrl Pts',(-15.0719627020186,8.81495027721556,7.));
#8861=CARTESIAN_POINT('Ctrl Pts',(-15.2508174554788,8.86505268915083,7.));
#8862=CARTESIAN_POINT('Ctrl Pts',(-15.4526569741556,8.91357927057117,7.));
#8863=CARTESIAN_POINT('Ctrl Pts',(-15.6775844882863,8.95887481023116,7.));
#8864=CARTESIAN_POINT('Ctrl Pts',(-15.9256093626227,8.99927973772153,7.));
#8865=CARTESIAN_POINT('Ctrl Pts',(-16.2671851013731,9.04193491022832,7.));
#8866=CARTESIAN_POINT('Ctrl Pts',(-16.5270428237395,9.06094720995306,7.));
#8867=CARTESIAN_POINT('Ctrl Pts',(-16.6962658094608,9.06833546026117,7.));
#8868=CARTESIAN_POINT('',(-17.1502563092003,8.17732893607296,7.));
#8869=CARTESIAN_POINT('Origin',(-1.73472347597681E-15,0.,7.));
#8870=CARTESIAN_POINT('',(-15.0980247376578,6.00933848448163,7.));
#8871=CARTESIAN_POINT('Ctrl Pts',(-17.1502563092003,8.17732893607296,7.));
#8872=CARTESIAN_POINT('Ctrl Pts',(-17.0448123137865,8.04476736935675,7.));
#8873=CARTESIAN_POINT('Ctrl Pts',(-16.8766905033057,7.8457132052331,7.));
#8874=CARTESIAN_POINT('Ctrl Pts',(-16.6414085620714,7.59444470905138,7.));
#8875=CARTESIAN_POINT('Ctrl Pts',(-16.4629349257385,7.41753779118423,7.));
#8876=CARTESIAN_POINT('Ctrl Pts',(-16.2940809887434,7.26219165995682,7.));
#8877=CARTESIAN_POINT('Ctrl Pts',(-16.1361838672874,7.12742326811386,7.));
#8878=CARTESIAN_POINT('Ctrl Pts',(-15.9905219781863,7.01217619187965,7.));
#8879=CARTESIAN_POINT('Ctrl Pts',(-15.8583036897432,6.91534043556372,7.));
#8880=CARTESIAN_POINT('Ctrl Pts',(-15.7406883947777,6.83570676658073,7.));
#8881=CARTESIAN_POINT('Ctrl Pts',(-15.6387111659832,6.77211692048666,7.));
#8882=CARTESIAN_POINT('Ctrl Pts',(-15.5619248294191,6.72790031412627,7.));
#8883=CARTESIAN_POINT('Ctrl Pts',(-15.5083268912118,6.69953551835476,7.));
#8884=CARTESIAN_POINT('Ctrl Pts',(-15.4733031879166,6.68074830397729,7.));
#8885=CARTESIAN_POINT('Ctrl Pts',(-15.4424051151807,6.66297054550545,7.));
#8886=CARTESIAN_POINT('Ctrl Pts',(-15.3933171197393,6.6330684552028,7.));
#8887=CARTESIAN_POINT('Ctrl Pts',(-15.3282076647861,6.58832104206026,7.));
#8888=CARTESIAN_POINT('Ctrl Pts',(-15.2506809503975,6.5224699530223,7.));
#8889=CARTESIAN_POINT('Ctrl Pts',(-15.1795880240196,6.443978909085,7.));
#8890=CARTESIAN_POINT('Ctrl Pts',(-15.1168047097501,6.34385243988827,7.));
#8891=CARTESIAN_POINT('Ctrl Pts',(-15.0680440207731,6.19604134326095,7.));
#8892=CARTESIAN_POINT('Ctrl Pts',(-15.0769402326058,6.07637133495398,7.));
#8893=CARTESIAN_POINT('Ctrl Pts',(-15.0980247376578,6.00933848448163,7.));
#8894=CARTESIAN_POINT('',(-15.7467591314704,4.01273932064536,7.));
#8895=CARTESIAN_POINT('Origin',(0.,0.,7.));
#8896=CARTESIAN_POINT('',(-18.6813621637973,3.46506965370702,7.));
#8897=CARTESIAN_POINT('Ctrl Pts',(-15.7467591314704,4.01273932064536,7.));
#8898=CARTESIAN_POINT('Ctrl Pts',(-15.7691023294921,3.94611544431018,7.));
#8899=CARTESIAN_POINT('Ctrl Pts',(-15.8322454089585,3.84407131175636,7.));
#8900=CARTESIAN_POINT('Ctrl Pts',(-15.958574817721,3.75315043649999,7.));
#8901=CARTESIAN_POINT('Ctrl Pts',(-16.0682204478862,3.7090495275507,7.));
#8902=CARTESIAN_POINT('Ctrl Pts',(-16.1718717115691,3.68733631276638,7.));
#8903=CARTESIAN_POINT('Ctrl Pts',(-16.2732984400115,3.67963072201295,7.));
#8904=CARTESIAN_POINT('Ctrl Pts',(-16.3522749650865,3.68169968173258,7.));
#8905=CARTESIAN_POINT('Ctrl Pts',(-16.409563995311,3.68636158229543,7.));
#8906=CARTESIAN_POINT('Ctrl Pts',(-16.4450105654964,3.69014050504823,7.));
#8907=CARTESIAN_POINT('Ctrl Pts',(-16.4843881842109,3.69552774561757,7.));
#8908=CARTESIAN_POINT('Ctrl Pts',(-16.5444222357228,3.70408422142789,7.));
#8909=CARTESIAN_POINT('Ctrl Pts',(-16.632533556064,3.7134461116587,7.));
#8910=CARTESIAN_POINT('Ctrl Pts',(-16.7524120409277,3.72194155665404,7.));
#8911=CARTESIAN_POINT('Ctrl Pts',(-16.8943723095674,3.72664910094711,7.));
#8912=CARTESIAN_POINT('Ctrl Pts',(-17.0582577813421,3.72602328845453,7.));
#8913=CARTESIAN_POINT('Ctrl Pts',(-17.2438412568379,3.71840435546374,7.));
#8914=CARTESIAN_POINT('Ctrl Pts',(-17.4507975846592,3.70218403552947,7.));
#8915=CARTESIAN_POINT('Ctrl Pts',(-17.6787134541915,3.67575622931334,7.));
#8916=CARTESIAN_POINT('Ctrl Pts',(-17.9270849363835,3.63753969769581,7.));
#8917=CARTESIAN_POINT('Ctrl Pts',(-18.265123941733,3.57255446932205,7.));
#8918=CARTESIAN_POINT('Ctrl Pts',(-18.5181384456163,3.51033578853423,7.));
#8919=CARTESIAN_POINT('Ctrl Pts',(-18.6813621637973,3.46506965370702,7.));
#8920=CARTESIAN_POINT('',(-18.8377966288375,2.47738131311205,7.));
#8921=CARTESIAN_POINT('Origin',(0.,0.,7.));
#8922=CARTESIAN_POINT('Ctrl Pts',(-18.8377966288375,2.47738131311205,7.));
#8923=CARTESIAN_POINT('Ctrl Pts',(-18.6965496529788,2.38389175781397,7.));
#8924=CARTESIAN_POINT('Ctrl Pts',(-18.4751451900744,2.24653249449212,7.));
#8925=CARTESIAN_POINT('Ctrl Pts',(-18.1737325312257,2.08026807216975,7.));
#8926=CARTESIAN_POINT('Ctrl Pts',(-17.949326772361,1.96717098182926,7.));
#8927=CARTESIAN_POINT('Ctrl Pts',(-17.7407325407201,1.87160676754277,7.));
#8928=CARTESIAN_POINT('Ctrl Pts',(-17.548917731071,1.79222730418272,7.));
#8929=CARTESIAN_POINT('Ctrl Pts',(-17.3747717371572,1.72763282051119,7.));
#8930=CARTESIAN_POINT('Ctrl Pts',(-17.2191007779952,1.67639424155264,7.));
#8931=CARTESIAN_POINT('Ctrl Pts',(-17.0826338282621,1.63700324669263,7.));
#8932=CARTESIAN_POINT('Ctrl Pts',(-16.9659973771906,1.60803840593145,7.));
#8933=CARTESIAN_POINT('Ctrl Pts',(-16.8793055486399,1.58971419725805,7.));
#8934=CARTESIAN_POINT('Ctrl Pts',(-16.8195656763126,1.57930034717566,7.));
#8935=CARTESIAN_POINT('Ctrl Pts',(-16.7804505865492,1.57225556404312,7.));
#8936=CARTESIAN_POINT('Ctrl Pts',(-16.7455711436431,1.56489594057218,7.));
#8937=CARTESIAN_POINT('Ctrl Pts',(-16.6896454316358,1.55162638755017,7.));
#8938=CARTESIAN_POINT('Ctrl Pts',(-16.6138949491149,1.52918899676863,7.));
#8939=CARTESIAN_POINT('Ctrl Pts',(-16.5198135565977,1.4905179616981,7.));
#8940=CARTESIAN_POINT('Ctrl Pts',(-16.4279450992207,1.43783746532133,7.));
#8941=CARTESIAN_POINT('Ctrl Pts',(-16.3372938385016,1.3620126454106,7.));
#8942=CARTESIAN_POINT('Ctrl Pts',(-16.2452435266959,1.23650382033378,7.));
#8943=CARTESIAN_POINT('Ctrl Pts',(-16.2167242606458,1.1199417984865,7.));
#8944=CARTESIAN_POINT('Ctrl Pts',(-16.2160625265911,1.04967429885986,7.));
#8945=CARTESIAN_POINT('',(-18.8377966288376,-2.47738131311187,7.));
#8946=CARTESIAN_POINT('Ctrl Pts',(-16.2160625265912,-1.04967429885971,7.));
#8947=CARTESIAN_POINT('Ctrl Pts',(-16.2167242606459,-1.11994179848649,7.));
#8948=CARTESIAN_POINT('Ctrl Pts',(-16.2452435266959,-1.23650382033376,7.));
#8949=CARTESIAN_POINT('Ctrl Pts',(-16.3372938385016,-1.36201264541056,7.));
#8950=CARTESIAN_POINT('Ctrl Pts',(-16.4279450992208,-1.43783746532131,7.));
#8951=CARTESIAN_POINT('Ctrl Pts',(-16.5198135565978,-1.49051796169811,7.));
#8952=CARTESIAN_POINT('Ctrl Pts',(-16.6138949491149,-1.52918899676863,7.));
#8953=CARTESIAN_POINT('Ctrl Pts',(-16.6896454316359,-1.55162638755017,7.));
#8954=CARTESIAN_POINT('Ctrl Pts',(-16.7455711436431,-1.56489594057219,7.));
#8955=CARTESIAN_POINT('Ctrl Pts',(-16.7804505865492,-1.57225556404312,7.));
#8956=CARTESIAN_POINT('Ctrl Pts',(-16.8195656763126,-1.57930034717562,7.));
#8957=CARTESIAN_POINT('Ctrl Pts',(-16.8793055486399,-1.58971419725805,7.));
#8958=CARTESIAN_POINT('Ctrl Pts',(-16.9659973771906,-1.60803840593145,7.));
#8959=CARTESIAN_POINT('Ctrl Pts',(-17.0826338282621,-1.63700324669261,7.));
#8960=CARTESIAN_POINT('Ctrl Pts',(-17.2191007779953,-1.67639424155264,7.));
#8961=CARTESIAN_POINT('Ctrl Pts',(-17.3747717371572,-1.72763282051121,7.));
#8962=CARTESIAN_POINT('Ctrl Pts',(-17.548917731071,-1.79222730418269,7.));
#8963=CARTESIAN_POINT('Ctrl Pts',(-17.7407325407201,-1.87160676754278,7.));
#8964=CARTESIAN_POINT('Ctrl Pts',(-17.949326772361,-1.96717098182925,7.));
#8965=CARTESIAN_POINT('Ctrl Pts',(-18.1737325312258,-2.08026807216972,7.));
#8966=CARTESIAN_POINT('Ctrl Pts',(-18.4751451900744,-2.2465324944921,7.));
#8967=CARTESIAN_POINT('Ctrl Pts',(-18.6965496529788,-2.38389175781394,7.));
#8968=CARTESIAN_POINT('Ctrl Pts',(-18.8377966288376,-2.47738131311187,7.));
#8969=CARTESIAN_POINT('',(-18.6813621637974,-3.46506965370684,7.));
#8970=CARTESIAN_POINT('Origin',(0.,0.,7.));
#8971=CARTESIAN_POINT('',(-15.7467591314705,-4.0127393206452,7.));
#8972=CARTESIAN_POINT('Ctrl Pts',(-18.6813621637974,-3.46506965370684,7.));
#8973=CARTESIAN_POINT('Ctrl Pts',(-18.5181384456162,-3.51033578853419,7.));
#8974=CARTESIAN_POINT('Ctrl Pts',(-18.265123941733,-3.57255446932203,7.));
#8975=CARTESIAN_POINT('Ctrl Pts',(-17.9270849363835,-3.63753969769578,7.));
#8976=CARTESIAN_POINT('Ctrl Pts',(-17.6787134541915,-3.67575622931333,7.));
#8977=CARTESIAN_POINT('Ctrl Pts',(-17.4507975846592,-3.70218403552949,7.));
#8978=CARTESIAN_POINT('Ctrl Pts',(-17.2438412568379,-3.71840435546371,7.));
#8979=CARTESIAN_POINT('Ctrl Pts',(-17.0582577813421,-3.72602328845455,7.));
#8980=CARTESIAN_POINT('Ctrl Pts',(-16.8943723095674,-3.7266491009471,7.));
#8981=CARTESIAN_POINT('Ctrl Pts',(-16.7524120409277,-3.72194155665402,7.));
#8982=CARTESIAN_POINT('Ctrl Pts',(-16.632533556064,-3.7134461116587,7.));
#8983=CARTESIAN_POINT('Ctrl Pts',(-16.5444222357228,-3.70408422142789,7.));
#8984=CARTESIAN_POINT('Ctrl Pts',(-16.4843881842109,-3.69552774561754,7.));
#8985=CARTESIAN_POINT('Ctrl Pts',(-16.4450105654964,-3.69014050504824,7.));
#8986=CARTESIAN_POINT('Ctrl Pts',(-16.409563995311,-3.68636158229544,7.));
#8987=CARTESIAN_POINT('Ctrl Pts',(-16.3522749650865,-3.68169968173258,7.));
#8988=CARTESIAN_POINT('Ctrl Pts',(-16.2732984400115,-3.67963072201294,7.));
#8989=CARTESIAN_POINT('Ctrl Pts',(-16.1718717115691,-3.68733631276639,7.));
#8990=CARTESIAN_POINT('Ctrl Pts',(-16.0682204478862,-3.70904952755068,7.));
#8991=CARTESIAN_POINT('Ctrl Pts',(-15.958574817721,-3.75315043649995,7.));
#8992=CARTESIAN_POINT('Ctrl Pts',(-15.8322454089585,-3.84407131175635,7.));
#8993=CARTESIAN_POINT('Ctrl Pts',(-15.7691023294921,-3.94611544431017,7.));
#8994=CARTESIAN_POINT('Ctrl Pts',(-15.7467591314705,-4.0127393206452,7.));
#8995=CARTESIAN_POINT('',(-15.0980247376579,-6.00933848448149,7.));
#8996=CARTESIAN_POINT('Origin',(0.,0.,7.));
#8997=CARTESIAN_POINT('',(-17.1502563092004,-8.1773289360728,7.));
#8998=CARTESIAN_POINT('Ctrl Pts',(-15.0980247376579,-6.00933848448149,7.));
#8999=CARTESIAN_POINT('Ctrl Pts',(-15.0769402326058,-6.07637133495397,7.));
#9000=CARTESIAN_POINT('Ctrl Pts',(-15.0680440207731,-6.19604134326091,7.));
#9001=CARTESIAN_POINT('Ctrl Pts',(-15.1168047097502,-6.34385243988823,7.));
#9002=CARTESIAN_POINT('Ctrl Pts',(-15.1795880240196,-6.44397890908498,7.));
#9003=CARTESIAN_POINT('Ctrl Pts',(-15.2506809503975,-6.52246995302231,7.));
#9004=CARTESIAN_POINT('Ctrl Pts',(-15.3282076647862,-6.58832104206025,7.));
#9005=CARTESIAN_POINT('Ctrl Pts',(-15.3933171197393,-6.63306845520279,7.));
#9006=CARTESIAN_POINT('Ctrl Pts',(-15.4424051151807,-6.66297054550545,7.));
#9007=CARTESIAN_POINT('Ctrl Pts',(-15.4733031879166,-6.68074830397729,7.));
#9008=CARTESIAN_POINT('Ctrl Pts',(-15.5083268912119,-6.69953551835472,7.));
#9009=CARTESIAN_POINT('Ctrl Pts',(-15.5619248294191,-6.72790031412626,7.));
#9010=CARTESIAN_POINT('Ctrl Pts',(-15.6387111659832,-6.77211692048665,7.));
#9011=CARTESIAN_POINT('Ctrl Pts',(-15.7406883947778,-6.8357067665807,7.));
#9012=CARTESIAN_POINT('Ctrl Pts',(-15.8583036897433,-6.91534043556372,7.));
#9013=CARTESIAN_POINT('Ctrl Pts',(-15.9905219781863,-7.01217619187965,7.));
#9014=CARTESIAN_POINT('Ctrl Pts',(-16.1361838672874,-7.12742326811382,7.));
#9015=CARTESIAN_POINT('Ctrl Pts',(-16.2940809887434,-7.26219165995681,7.));
#9016=CARTESIAN_POINT('Ctrl Pts',(-16.4629349257385,-7.41753779118423,7.));
#9017=CARTESIAN_POINT('Ctrl Pts',(-16.6414085620714,-7.59444470905136,7.));
#9018=CARTESIAN_POINT('Ctrl Pts',(-16.8766905033058,-7.84571320523309,7.));
#9019=CARTESIAN_POINT('Ctrl Pts',(-17.0448123137865,-8.04476736935674,7.));
#9020=CARTESIAN_POINT('Ctrl Pts',(-17.1502563092004,-8.1773289360728,7.));
#9021=CARTESIAN_POINT('',(-16.6962658094609,-9.06833546026103,7.));
#9022=CARTESIAN_POINT('Origin',(0.,0.,7.));
#9023=CARTESIAN_POINT('',(-13.7360532384392,-8.68235805704666,7.));
#9024=CARTESIAN_POINT('Ctrl Pts',(-16.6962658094609,-9.06833546026103,7.));
#9025=CARTESIAN_POINT('Ctrl Pts',(-16.5270428237395,-9.06094720995301,7.));
#9026=CARTESIAN_POINT('Ctrl Pts',(-16.2671851013731,-9.0419349102283,7.));
#9027=CARTESIAN_POINT('Ctrl Pts',(-15.9256093626227,-8.99927973772149,7.));
#9028=CARTESIAN_POINT('Ctrl Pts',(-15.6775844882862,-8.95887481023114,7.));
#9029=CARTESIAN_POINT('Ctrl Pts',(-15.4526569741556,-8.91357927057118,7.));
#9030=CARTESIAN_POINT('Ctrl Pts',(-15.2508174554788,-8.8650526891508,7.));
#9031=CARTESIAN_POINT('Ctrl Pts',(-15.0719627020186,-8.81495027721558,7.));
#9032=CARTESIAN_POINT('Ctrl Pts',(-14.9159049694657,-8.76490206435507,7.));
#9033=CARTESIAN_POINT('Ctrl Pts',(-14.7823474421093,-8.71655678814369,7.));
#9034=CARTESIAN_POINT('Ctrl Pts',(-14.6709614647944,-8.67143265073926,7.));
#9035=CARTESIAN_POINT('Ctrl Pts',(-14.5900556026053,-8.63530106864816,7.));
#9036=CARTESIAN_POINT('Ctrl Pts',(-14.5356039231527,-8.60861183441385,7.));
#9037=CARTESIAN_POINT('Ctrl Pts',(-14.4998183311667,-8.59131991078476,7.));
#9038=CARTESIAN_POINT('Ctrl Pts',(-14.4672743909627,-8.57677234909656,7.));
#9039=CARTESIAN_POINT('Ctrl Pts',(-14.4142298919554,-8.5546353342573,7.));
#9040=CARTESIAN_POINT('Ctrl Pts',(-14.3397580968625,-8.52826254822913,7.));
#9041=CARTESIAN_POINT('Ctrl Pts',(-14.2409143873564,-8.50424841775454,7.));
#9042=CARTESIAN_POINT('Ctrl Pts',(-14.1356264252376,-8.4928689101984,7.));
#9043=CARTESIAN_POINT('Ctrl Pts',(-14.0177193038531,-8.50092900394916,7.));
#9044=CARTESIAN_POINT('Ctrl Pts',(-13.8694768008521,-8.54836196063206,7.));
#9045=CARTESIAN_POINT('Ctrl Pts',(-13.7778907925313,-8.62589941321478,7.));
#9046=CARTESIAN_POINT('Ctrl Pts',(-13.7360532384392,-8.68235805704666,7.));
#9047=CARTESIAN_POINT('',(-12.5020870932788,-10.380766749719,7.));
#9048=CARTESIAN_POINT('Origin',(0.,0.,7.));
#9049=CARTESIAN_POINT('',(-13.7839294091566,-13.07682262797,7.));
#9050=CARTESIAN_POINT('Ctrl Pts',(-12.5020870932788,-10.380766749719,7.));
#9051=CARTESIAN_POINT('Ctrl Pts',(-12.4613202473788,-10.4380033085876,7.));
#9052=CARTESIAN_POINT('Ctrl Pts',(-12.4158793808611,-10.5490671691512,7.));
#9053=CARTESIAN_POINT('Ctrl Pts',(-12.4165774110367,-10.7047117573306,7.));
#9054=CARTESIAN_POINT('Ctrl Pts',(-12.4453471106188,-10.8193387993863,7.));
#9055=CARTESIAN_POINT('Ctrl Pts',(-12.4887054350301,-10.9159571406243,7.));
#9056=CARTESIAN_POINT('Ctrl Pts',(-12.5420886163255,-11.0025423202231,7.));
#9057=CARTESIAN_POINT('Ctrl Pts',(-12.5901836766158,-11.0652195671547,7.));
#9058=CARTESIAN_POINT('Ctrl Pts',(-12.6276288804813,-11.1088271697991,7.));
#9059=CARTESIAN_POINT('Ctrl Pts',(-12.6515210644081,-11.1352828524077,7.));
#9060=CARTESIAN_POINT('Ctrl Pts',(-12.6790250171322,-11.1639734745885,7.));
#9061=CARTESIAN_POINT('Ctrl Pts',(-12.7212344815888,-11.2075126722099,7.));
#9062=CARTESIAN_POINT('Ctrl Pts',(-12.7805989445416,-11.2732934467515,7.));
#9063=CARTESIAN_POINT('Ctrl Pts',(-12.8579347093876,-11.3652836809863,7.));
#9064=CARTESIAN_POINT('Ctrl Pts',(-12.9451853450404,-11.4773649257318,7.));
#9065=CARTESIAN_POINT('Ctrl Pts',(-13.0410085154727,-11.6103189008825,7.));
#9066=CARTESIAN_POINT('Ctrl Pts',(-13.1439278991698,-11.764937382884,7.));
#9067=CARTESIAN_POINT('Ctrl Pts',(-13.2524512620508,-11.9419026340297,7.));
#9068=CARTESIAN_POINT('Ctrl Pts',(-13.3650363045724,-12.1418243205134,7.));
#9069=CARTESIAN_POINT('Ctrl Pts',(-13.4801075753502,-12.3652241842034,7.));
#9070=CARTESIAN_POINT('Ctrl Pts',(-13.6262277632565,-12.6769008431476,7.));
#9071=CARTESIAN_POINT('Ctrl Pts',(-13.7246099871303,-12.9181650995967,7.));
#9072=CARTESIAN_POINT('Ctrl Pts',(-13.7839294091566,-13.07682262797,7.));
#9073=CARTESIAN_POINT('',(-13.0768226279701,-13.7839294091565,7.));
#9074=CARTESIAN_POINT('Origin',(0.,0.,7.));
#9075=CARTESIAN_POINT('',(-10.3807667497191,-12.5020870932787,7.));
#9076=CARTESIAN_POINT('Ctrl Pts',(-13.0768226279701,-13.7839294091565,7.));
#9077=CARTESIAN_POINT('Ctrl Pts',(-12.9181650995967,-13.7246099871302,7.));
#9078=CARTESIAN_POINT('Ctrl Pts',(-12.6769008431476,-13.6262277632565,7.));
#9079=CARTESIAN_POINT('Ctrl Pts',(-12.3652241842034,-13.4801075753502,7.));
#9080=CARTESIAN_POINT('Ctrl Pts',(-12.1418243205134,-13.3650363045723,7.));
#9081=CARTESIAN_POINT('Ctrl Pts',(-11.9419026340297,-13.2524512620508,7.));
#9082=CARTESIAN_POINT('Ctrl Pts',(-11.764937382884,-13.1439278991698,7.));
#9083=CARTESIAN_POINT('Ctrl Pts',(-11.6103189008825,-13.0410085154728,7.));
#9084=CARTESIAN_POINT('Ctrl Pts',(-11.4773649257318,-12.9451853450404,7.));
#9085=CARTESIAN_POINT('Ctrl Pts',(-11.3652836809863,-12.8579347093876,7.));
#9086=CARTESIAN_POINT('Ctrl Pts',(-11.2732934467515,-12.7805989445416,7.));
#9087=CARTESIAN_POINT('Ctrl Pts',(-11.2075126722099,-12.7212344815888,7.));
#9088=CARTESIAN_POINT('Ctrl Pts',(-11.1639734745886,-12.6790250171322,7.));
#9089=CARTESIAN_POINT('Ctrl Pts',(-11.1352828524077,-12.651521064408,7.));
#9090=CARTESIAN_POINT('Ctrl Pts',(-11.1088271697991,-12.6276288804813,7.));
#9091=CARTESIAN_POINT('Ctrl Pts',(-11.0652195671547,-12.5901836766158,7.));
#9092=CARTESIAN_POINT('Ctrl Pts',(-11.0025423202231,-12.5420886163255,7.));
#9093=CARTESIAN_POINT('Ctrl Pts',(-10.9159571406243,-12.48870543503,7.));
#9094=CARTESIAN_POINT('Ctrl Pts',(-10.8193387993863,-12.4453471106187,7.));
#9095=CARTESIAN_POINT('Ctrl Pts',(-10.7047117573307,-12.4165774110367,7.));
#9096=CARTESIAN_POINT('Ctrl Pts',(-10.5490671691512,-12.4158793808611,7.));
#9097=CARTESIAN_POINT('Ctrl Pts',(-10.4380033085876,-12.4613202473787,7.));
#9098=CARTESIAN_POINT('Ctrl Pts',(-10.3807667497191,-12.5020870932787,7.));
#9099=CARTESIAN_POINT('',(-8.68235805704677,-13.7360532384392,7.));
#9100=CARTESIAN_POINT('Origin',(0.,0.,7.));
#9101=CARTESIAN_POINT('',(-9.06833546026116,-16.6962658094608,7.));
#9102=CARTESIAN_POINT('Ctrl Pts',(-8.68235805704677,-13.7360532384392,7.));
#9103=CARTESIAN_POINT('Ctrl Pts',(-8.62589941321481,-13.7778907925313,7.));
#9104=CARTESIAN_POINT('Ctrl Pts',(-8.54836196063208,-13.8694768008521,7.));
#9105=CARTESIAN_POINT('Ctrl Pts',(-8.50092900394921,-14.0177193038531,7.));
#9106=CARTESIAN_POINT('Ctrl Pts',(-8.49286891019844,-14.1356264252377,7.));
#9107=CARTESIAN_POINT('Ctrl Pts',(-8.50424841775456,-14.2409143873564,7.));
#9108=CARTESIAN_POINT('Ctrl Pts',(-8.52826254822915,-14.3397580968626,7.));
#9109=CARTESIAN_POINT('Ctrl Pts',(-8.55463533425732,-14.4142298919555,7.));
#9110=CARTESIAN_POINT('Ctrl Pts',(-8.57677234909656,-14.4672743909627,7.));
#9111=CARTESIAN_POINT('Ctrl Pts',(-8.59131991078476,-14.4998183311667,7.));
#9112=CARTESIAN_POINT('Ctrl Pts',(-8.6086118344139,-14.5356039231527,7.));
#9113=CARTESIAN_POINT('Ctrl Pts',(-8.63530106864818,-14.5900556026053,7.));
#9114=CARTESIAN_POINT('Ctrl Pts',(-8.67143265073928,-14.6709614647944,7.));
#9115=CARTESIAN_POINT('Ctrl Pts',(-8.71655678814373,-14.7823474421093,7.));
#9116=CARTESIAN_POINT('Ctrl Pts',(-8.76490206435509,-14.9159049694657,7.));
#9117=CARTESIAN_POINT('Ctrl Pts',(-8.81495027721557,-15.0719627020186,7.));
#9118=CARTESIAN_POINT('Ctrl Pts',(-8.86505268915084,-15.2508174554788,7.));
#9119=CARTESIAN_POINT('Ctrl Pts',(-8.91357927057117,-15.4526569741556,7.));
#9120=CARTESIAN_POINT('Ctrl Pts',(-8.95887481023116,-15.6775844882862,7.));
#9121=CARTESIAN_POINT('Ctrl Pts',(-8.99927973772154,-15.9256093626227,7.));
#9122=CARTESIAN_POINT('Ctrl Pts',(-9.04193491022832,-16.2671851013731,7.));
#9123=CARTESIAN_POINT('Ctrl Pts',(-9.06094720995306,-16.5270428237395,7.));
#9124=CARTESIAN_POINT('Ctrl Pts',(-9.06833546026116,-16.6962658094608,7.));
#9125=CARTESIAN_POINT('',(-8.17732893607292,-17.1502563092003,7.));
#9126=CARTESIAN_POINT('Origin',(0.,0.,7.));
#9127=CARTESIAN_POINT('',(-6.0093384844816,-15.0980247376578,7.));
#9128=CARTESIAN_POINT('Ctrl Pts',(-8.17732893607292,-17.1502563092003,7.));
#9129=CARTESIAN_POINT('Ctrl Pts',(-8.04476736935674,-17.0448123137865,7.));
#9130=CARTESIAN_POINT('Ctrl Pts',(-7.8457132052331,-16.8766905033057,7.));
#9131=CARTESIAN_POINT('Ctrl Pts',(-7.59444470905137,-16.6414085620714,7.));
#9132=CARTESIAN_POINT('Ctrl Pts',(-7.41753779118422,-16.4629349257385,7.));
#9133=CARTESIAN_POINT('Ctrl Pts',(-7.2621916599568,-16.2940809887434,7.));
#9134=CARTESIAN_POINT('Ctrl Pts',(-7.12742326811384,-16.1361838672874,7.));
#9135=CARTESIAN_POINT('Ctrl Pts',(-7.01217619187963,-15.9905219781863,7.));
#9136=CARTESIAN_POINT('Ctrl Pts',(-6.9153404355637,-15.8583036897432,7.));
#9137=CARTESIAN_POINT('Ctrl Pts',(-6.8357067665807,-15.7406883947777,7.));
#9138=CARTESIAN_POINT('Ctrl Pts',(-6.77211692048664,-15.6387111659832,7.));
#9139=CARTESIAN_POINT('Ctrl Pts',(-6.72790031412625,-15.5619248294191,7.));
#9140=CARTESIAN_POINT('Ctrl Pts',(-6.69953551835473,-15.5083268912118,7.));
#9141=CARTESIAN_POINT('Ctrl Pts',(-6.68074830397727,-15.4733031879166,7.));
#9142=CARTESIAN_POINT('Ctrl Pts',(-6.66297054550543,-15.4424051151807,7.));
#9143=CARTESIAN_POINT('Ctrl Pts',(-6.63306845520277,-15.3933171197393,7.));
#9144=CARTESIAN_POINT('Ctrl Pts',(-6.58832104206024,-15.3282076647861,7.));
#9145=CARTESIAN_POINT('Ctrl Pts',(-6.52246995302227,-15.2506809503975,7.));
#9146=CARTESIAN_POINT('Ctrl Pts',(-6.44397890908497,-15.1795880240196,7.));
#9147=CARTESIAN_POINT('Ctrl Pts',(-6.34385243988824,-15.1168047097501,7.));
#9148=CARTESIAN_POINT('Ctrl Pts',(-6.19604134326091,-15.0680440207731,7.));
#9149=CARTESIAN_POINT('Ctrl Pts',(-6.07637133495395,-15.0769402326058,7.));
#9150=CARTESIAN_POINT('Ctrl Pts',(-6.0093384844816,-15.0980247376578,7.));
#9151=CARTESIAN_POINT('',(-4.01273932064531,-15.7467591314704,7.));
#9152=CARTESIAN_POINT('Origin',(0.,0.,7.));
#9153=CARTESIAN_POINT('',(-3.46506965370701,-18.6813621637973,7.));
#9154=CARTESIAN_POINT('Ctrl Pts',(-4.01273932064531,-15.7467591314704,7.));
#9155=CARTESIAN_POINT('Ctrl Pts',(-3.94611544431022,-15.7691023294921,7.));
#9156=CARTESIAN_POINT('Ctrl Pts',(-3.8440713117564,-15.8322454089585,7.));
#9157=CARTESIAN_POINT('Ctrl Pts',(-3.75315043650002,-15.958574817721,7.));
#9158=CARTESIAN_POINT('Ctrl Pts',(-3.70904952755073,-16.0682204478862,7.));
#9159=CARTESIAN_POINT('Ctrl Pts',(-3.68733631276642,-16.1718717115691,7.));
#9160=CARTESIAN_POINT('Ctrl Pts',(-3.67963072201298,-16.2732984400115,7.));
#9161=CARTESIAN_POINT('Ctrl Pts',(-3.68169968173261,-16.3522749650865,7.));
#9162=CARTESIAN_POINT('Ctrl Pts',(-3.68636158229546,-16.409563995311,7.));
#9163=CARTESIAN_POINT('Ctrl Pts',(-3.69014050504826,-16.4450105654963,7.));
#9164=CARTESIAN_POINT('Ctrl Pts',(-3.6955277456176,-16.4843881842109,7.));
#9165=CARTESIAN_POINT('Ctrl Pts',(-3.70408422142792,-16.5444222357228,7.));
#9166=CARTESIAN_POINT('Ctrl Pts',(-3.71344611165872,-16.632533556064,7.));
#9167=CARTESIAN_POINT('Ctrl Pts',(-3.72194155665407,-16.7524120409277,7.));
#9168=CARTESIAN_POINT('Ctrl Pts',(-3.72664910094713,-16.8943723095674,7.));
#9169=CARTESIAN_POINT('Ctrl Pts',(-3.72602328845455,-17.0582577813421,7.));
#9170=CARTESIAN_POINT('Ctrl Pts',(-3.71840435546375,-17.2438412568379,7.));
#9171=CARTESIAN_POINT('Ctrl Pts',(-3.70218403552949,-17.4507975846592,7.));
#9172=CARTESIAN_POINT('Ctrl Pts',(-3.67575622931335,-17.6787134541915,7.));
#9173=CARTESIAN_POINT('Ctrl Pts',(-3.63753969769582,-17.9270849363835,7.));
#9174=CARTESIAN_POINT('Ctrl Pts',(-3.57255446932205,-18.265123941733,7.));
#9175=CARTESIAN_POINT('Ctrl Pts',(-3.51033578853422,-18.5181384456163,7.));
#9176=CARTESIAN_POINT('Ctrl Pts',(-3.46506965370701,-18.6813621637973,7.));
#9177=CARTESIAN_POINT('',(-2.47738131311198,-18.8377966288376,7.));
#9178=CARTESIAN_POINT('Origin',(0.,0.,7.));
#9179=CARTESIAN_POINT('',(-1.04967429885986,-16.2160625265911,7.));
#9180=CARTESIAN_POINT('Ctrl Pts',(-2.47738131311198,-18.8377966288376,7.));
#9181=CARTESIAN_POINT('Ctrl Pts',(-2.38389175781398,-18.6965496529788,7.));
#9182=CARTESIAN_POINT('Ctrl Pts',(-2.24653249449213,-18.4751451900744,7.));
#9183=CARTESIAN_POINT('Ctrl Pts',(-2.08026807216976,-18.1737325312257,7.));
#9184=CARTESIAN_POINT('Ctrl Pts',(-1.96717098182926,-17.949326772361,7.));
#9185=CARTESIAN_POINT('Ctrl Pts',(-1.87160676754278,-17.7407325407201,7.));
#9186=CARTESIAN_POINT('Ctrl Pts',(-1.79222730418273,-17.548917731071,7.));
#9187=CARTESIAN_POINT('Ctrl Pts',(-1.7276328205112,-17.3747717371572,7.));
#9188=CARTESIAN_POINT('Ctrl Pts',(-1.67639424155264,-17.2191007779952,7.));
#9189=CARTESIAN_POINT('Ctrl Pts',(-1.63700324669264,-17.0826338282621,7.));
#9190=CARTESIAN_POINT('Ctrl Pts',(-1.60803840593146,-16.9659973771906,7.));
#9191=CARTESIAN_POINT('Ctrl Pts',(-1.58971419725806,-16.8793055486399,7.));
#9192=CARTESIAN_POINT('Ctrl Pts',(-1.57930034717566,-16.8195656763126,7.));
#9193=CARTESIAN_POINT('Ctrl Pts',(-1.57225556404312,-16.7804505865492,7.));
#9194=CARTESIAN_POINT('Ctrl Pts',(-1.56489594057218,-16.7455711436431,7.));
#9195=CARTESIAN_POINT('Ctrl Pts',(-1.55162638755018,-16.6896454316358,7.));
#9196=CARTESIAN_POINT('Ctrl Pts',(-1.52918899676863,-16.6138949491149,7.));
#9197=CARTESIAN_POINT('Ctrl Pts',(-1.49051796169811,-16.5198135565977,7.));
#9198=CARTESIAN_POINT('Ctrl Pts',(-1.43783746532133,-16.4279450992207,7.));
#9199=CARTESIAN_POINT('Ctrl Pts',(-1.3620126454106,-16.3372938385016,7.));
#9200=CARTESIAN_POINT('Ctrl Pts',(-1.23650382033378,-16.2452435266959,7.));
#9201=CARTESIAN_POINT('Ctrl Pts',(-1.1199417984865,-16.2167242606458,7.));
#9202=CARTESIAN_POINT('Ctrl Pts',(-1.04967429885986,-16.2160625265911,7.));
#9203=CARTESIAN_POINT('',(1.04967429885974,-16.2160625265911,7.));
#9204=CARTESIAN_POINT('Origin',(0.,0.,7.));
#9205=CARTESIAN_POINT('',(2.47738131311187,-18.8377966288376,7.));
#9206=CARTESIAN_POINT('Ctrl Pts',(1.04967429885974,-16.2160625265911,7.));
#9207=CARTESIAN_POINT('Ctrl Pts',(1.11994179848648,-16.2167242606459,7.));
#9208=CARTESIAN_POINT('Ctrl Pts',(1.23650382033375,-16.2452435266959,7.));
#9209=CARTESIAN_POINT('Ctrl Pts',(1.36201264541055,-16.3372938385016,7.));
#9210=CARTESIAN_POINT('Ctrl Pts',(1.4378374653213,-16.4279450992208,7.));
#9211=CARTESIAN_POINT('Ctrl Pts',(1.4905179616981,-16.5198135565978,7.));
#9212=CARTESIAN_POINT('Ctrl Pts',(1.52918899676862,-16.6138949491149,7.));
#9213=CARTESIAN_POINT('Ctrl Pts',(1.55162638755016,-16.6896454316359,7.));
#9214=CARTESIAN_POINT('Ctrl Pts',(1.56489594057218,-16.7455711436431,7.));
#9215=CARTESIAN_POINT('Ctrl Pts',(1.57225556404312,-16.7804505865492,7.));
#9216=CARTESIAN_POINT('Ctrl Pts',(1.57930034717562,-16.8195656763126,7.));
#9217=CARTESIAN_POINT('Ctrl Pts',(1.58971419725804,-16.8793055486399,7.));
#9218=CARTESIAN_POINT('Ctrl Pts',(1.60803840593144,-16.9659973771906,7.));
#9219=CARTESIAN_POINT('Ctrl Pts',(1.6370032466926,-17.0826338282622,7.));
#9220=CARTESIAN_POINT('Ctrl Pts',(1.67639424155263,-17.2191007779953,7.));
#9221=CARTESIAN_POINT('Ctrl Pts',(1.72763282051121,-17.3747717371572,7.));
#9222=CARTESIAN_POINT('Ctrl Pts',(1.79222730418269,-17.548917731071,7.));
#9223=CARTESIAN_POINT('Ctrl Pts',(1.87160676754277,-17.7407325407201,7.));
#9224=CARTESIAN_POINT('Ctrl Pts',(1.96717098182925,-17.949326772361,7.));
#9225=CARTESIAN_POINT('Ctrl Pts',(2.08026807216972,-18.1737325312257,7.));
#9226=CARTESIAN_POINT('Ctrl Pts',(2.2465324944921,-18.4751451900744,7.));
#9227=CARTESIAN_POINT('Ctrl Pts',(2.38389175781394,-18.6965496529788,7.));
#9228=CARTESIAN_POINT('Ctrl Pts',(2.47738131311187,-18.8377966288376,7.));
#9229=CARTESIAN_POINT('',(3.46506965370692,-18.6813621637974,7.));
#9230=CARTESIAN_POINT('Origin',(0.,0.,7.));
#9231=CARTESIAN_POINT('',(4.01273932064523,-15.7467591314704,7.));
#9232=CARTESIAN_POINT('Ctrl Pts',(3.46506965370692,-18.6813621637974,7.));
#9233=CARTESIAN_POINT('Ctrl Pts',(3.51033578853419,-18.5181384456162,7.));
#9234=CARTESIAN_POINT('Ctrl Pts',(3.57255446932203,-18.2651239417329,7.));
#9235=CARTESIAN_POINT('Ctrl Pts',(3.63753969769579,-17.9270849363835,7.));
#9236=CARTESIAN_POINT('Ctrl Pts',(3.67575622931334,-17.6787134541915,7.));
#9237=CARTESIAN_POINT('Ctrl Pts',(3.7021840355295,-17.4507975846592,7.));
#9238=CARTESIAN_POINT('Ctrl Pts',(3.71840435546372,-17.2438412568379,7.));
#9239=CARTESIAN_POINT('Ctrl Pts',(3.72602328845457,-17.0582577813421,7.));
#9240=CARTESIAN_POINT('Ctrl Pts',(3.72664910094712,-16.8943723095674,7.));
#9241=CARTESIAN_POINT('Ctrl Pts',(3.72194155665404,-16.7524120409277,7.));
#9242=CARTESIAN_POINT('Ctrl Pts',(3.71344611165872,-16.632533556064,7.));
#9243=CARTESIAN_POINT('Ctrl Pts',(3.70408422142791,-16.5444222357228,7.));
#9244=CARTESIAN_POINT('Ctrl Pts',(3.69552774561757,-16.4843881842109,7.));
#9245=CARTESIAN_POINT('Ctrl Pts',(3.69014050504827,-16.4450105654963,7.));
#9246=CARTESIAN_POINT('Ctrl Pts',(3.68636158229547,-16.409563995311,7.));
#9247=CARTESIAN_POINT('Ctrl Pts',(3.68169968173261,-16.3522749650865,7.));
#9248=CARTESIAN_POINT('Ctrl Pts',(3.67963072201297,-16.2732984400115,7.));
#9249=CARTESIAN_POINT('Ctrl Pts',(3.68733631276642,-16.1718717115691,7.));
#9250=CARTESIAN_POINT('Ctrl Pts',(3.70904952755071,-16.0682204478862,7.));
#9251=CARTESIAN_POINT('Ctrl Pts',(3.75315043649999,-15.958574817721,7.));
#9252=CARTESIAN_POINT('Ctrl Pts',(3.84407131175639,-15.8322454089585,7.));
#9253=CARTESIAN_POINT('Ctrl Pts',(3.94611544431021,-15.7691023294921,7.));
#9254=CARTESIAN_POINT('Ctrl Pts',(4.01273932064523,-15.7467591314704,7.));
#9255=CARTESIAN_POINT('',(6.00933848448151,-15.0980247376579,7.));
#9256=CARTESIAN_POINT('Origin',(0.,0.,7.));
#9257=CARTESIAN_POINT('',(8.17732893607279,-17.1502563092004,7.));
#9258=CARTESIAN_POINT('Ctrl Pts',(6.00933848448151,-15.0980247376579,7.));
#9259=CARTESIAN_POINT('Ctrl Pts',(6.07637133495396,-15.0769402326058,7.));
#9260=CARTESIAN_POINT('Ctrl Pts',(6.1960413432609,-15.0680440207731,7.));
#9261=CARTESIAN_POINT('Ctrl Pts',(6.34385243988821,-15.1168047097502,7.));
#9262=CARTESIAN_POINT('Ctrl Pts',(6.44397890908497,-15.1795880240196,7.));
#9263=CARTESIAN_POINT('Ctrl Pts',(6.52246995302229,-15.2506809503975,7.));
#9264=CARTESIAN_POINT('Ctrl Pts',(6.58832104206024,-15.3282076647862,7.));
#9265=CARTESIAN_POINT('Ctrl Pts',(6.63306845520277,-15.3933171197393,7.));
#9266=CARTESIAN_POINT('Ctrl Pts',(6.66297054550544,-15.4424051151807,7.));
#9267=CARTESIAN_POINT('Ctrl Pts',(6.68074830397727,-15.4733031879166,7.));
#9268=CARTESIAN_POINT('Ctrl Pts',(6.69953551835471,-15.5083268912119,7.));
#9269=CARTESIAN_POINT('Ctrl Pts',(6.72790031412625,-15.5619248294191,7.));
#9270=CARTESIAN_POINT('Ctrl Pts',(6.77211692048664,-15.6387111659832,7.));
#9271=CARTESIAN_POINT('Ctrl Pts',(6.83570676658069,-15.7406883947778,7.));
#9272=CARTESIAN_POINT('Ctrl Pts',(6.91534043556371,-15.8583036897433,7.));
#9273=CARTESIAN_POINT('Ctrl Pts',(7.01217619187964,-15.9905219781863,7.));
#9274=CARTESIAN_POINT('Ctrl Pts',(7.12742326811382,-16.1361838672874,7.));
#9275=CARTESIAN_POINT('Ctrl Pts',(7.2621916599568,-16.2940809887434,7.));
#9276=CARTESIAN_POINT('Ctrl Pts',(7.41753779118422,-16.4629349257385,7.));
#9277=CARTESIAN_POINT('Ctrl Pts',(7.59444470905135,-16.6414085620714,7.));
#9278=CARTESIAN_POINT('Ctrl Pts',(7.84571320523309,-16.8766905033058,7.));
#9279=CARTESIAN_POINT('Ctrl Pts',(8.04476736935673,-17.0448123137865,7.));
#9280=CARTESIAN_POINT('Ctrl Pts',(8.17732893607279,-17.1502563092004,7.));
#9281=CARTESIAN_POINT('',(9.06833546026109,-16.6962658094609,7.));
#9282=CARTESIAN_POINT('Origin',(0.,0.,7.));
#9283=CARTESIAN_POINT('',(8.68235805704667,-13.7360532384392,7.));
#9284=CARTESIAN_POINT('Ctrl Pts',(9.06833546026109,-16.6962658094609,7.));
#9285=CARTESIAN_POINT('Ctrl Pts',(9.06094720995301,-16.5270428237395,7.));
#9286=CARTESIAN_POINT('Ctrl Pts',(9.0419349102283,-16.267185101373,7.));
#9287=CARTESIAN_POINT('Ctrl Pts',(8.99927973772149,-15.9256093626227,7.));
#9288=CARTESIAN_POINT('Ctrl Pts',(8.95887481023114,-15.6775844882862,7.));
#9289=CARTESIAN_POINT('Ctrl Pts',(8.91357927057119,-15.4526569741556,7.));
#9290=CARTESIAN_POINT('Ctrl Pts',(8.8650526891508,-15.2508174554787,7.));
#9291=CARTESIAN_POINT('Ctrl Pts',(8.81495027721559,-15.0719627020186,7.));
#9292=CARTESIAN_POINT('Ctrl Pts',(8.76490206435508,-14.9159049694657,7.));
#9293=CARTESIAN_POINT('Ctrl Pts',(8.7165567881437,-14.7823474421092,7.));
#9294=CARTESIAN_POINT('Ctrl Pts',(8.67143265073927,-14.6709614647944,7.));
#9295=CARTESIAN_POINT('Ctrl Pts',(8.63530106864817,-14.5900556026053,7.));
#9296=CARTESIAN_POINT('Ctrl Pts',(8.60861183441386,-14.5356039231526,7.));
#9297=CARTESIAN_POINT('Ctrl Pts',(8.59131991078477,-14.4998183311667,7.));
#9298=CARTESIAN_POINT('Ctrl Pts',(8.57677234909656,-14.4672743909626,7.));
#9299=CARTESIAN_POINT('Ctrl Pts',(8.55463533425731,-14.4142298919554,7.));
#9300=CARTESIAN_POINT('Ctrl Pts',(8.52826254822914,-14.3397580968625,7.));
#9301=CARTESIAN_POINT('Ctrl Pts',(8.50424841775455,-14.2409143873564,7.));
#9302=CARTESIAN_POINT('Ctrl Pts',(8.49286891019841,-14.1356264252376,7.));
#9303=CARTESIAN_POINT('Ctrl Pts',(8.50092900394917,-14.0177193038531,7.));
#9304=CARTESIAN_POINT('Ctrl Pts',(8.54836196063206,-13.8694768008521,7.));
#9305=CARTESIAN_POINT('Ctrl Pts',(8.62589941321478,-13.7778907925312,7.));
#9306=CARTESIAN_POINT('Ctrl Pts',(8.68235805704667,-13.7360532384392,7.));
#9307=CARTESIAN_POINT('',(10.3807667497191,-12.5020870932787,7.));
#9308=CARTESIAN_POINT('Origin',(0.,0.,7.));
#9309=CARTESIAN_POINT('',(13.07682262797,-13.7839294091566,7.));
#9310=CARTESIAN_POINT('Ctrl Pts',(10.3807667497191,-12.5020870932787,7.));
#9311=CARTESIAN_POINT('Ctrl Pts',(10.4380033085876,-12.4613202473788,7.));
#9312=CARTESIAN_POINT('Ctrl Pts',(10.5490671691512,-12.4158793808611,7.));
#9313=CARTESIAN_POINT('Ctrl Pts',(10.7047117573306,-12.4165774110367,7.));
#9314=CARTESIAN_POINT('Ctrl Pts',(10.8193387993863,-12.4453471106188,7.));
#9315=CARTESIAN_POINT('Ctrl Pts',(10.9159571406243,-12.48870543503,7.));
#9316=CARTESIAN_POINT('Ctrl Pts',(11.0025423202231,-12.5420886163255,7.));
#9317=CARTESIAN_POINT('Ctrl Pts',(11.0652195671547,-12.5901836766158,7.));
#9318=CARTESIAN_POINT('Ctrl Pts',(11.1088271697991,-12.6276288804813,7.));
#9319=CARTESIAN_POINT('Ctrl Pts',(11.1352828524077,-12.651521064408,7.));
#9320=CARTESIAN_POINT('Ctrl Pts',(11.1639734745885,-12.6790250171322,7.));
#9321=CARTESIAN_POINT('Ctrl Pts',(11.2075126722099,-12.7212344815888,7.));
#9322=CARTESIAN_POINT('Ctrl Pts',(11.2732934467515,-12.7805989445416,7.));
#9323=CARTESIAN_POINT('Ctrl Pts',(11.3652836809863,-12.8579347093876,7.));
#9324=CARTESIAN_POINT('Ctrl Pts',(11.4773649257318,-12.9451853450404,7.));
#9325=CARTESIAN_POINT('Ctrl Pts',(11.6103189008825,-13.0410085154727,7.));
#9326=CARTESIAN_POINT('Ctrl Pts',(11.764937382884,-13.1439278991698,7.));
#9327=CARTESIAN_POINT('Ctrl Pts',(11.9419026340297,-13.2524512620507,7.));
#9328=CARTESIAN_POINT('Ctrl Pts',(12.1418243205134,-13.3650363045724,7.));
#9329=CARTESIAN_POINT('Ctrl Pts',(12.3652241842034,-13.4801075753502,7.));
#9330=CARTESIAN_POINT('Ctrl Pts',(12.6769008431476,-13.6262277632565,7.));
#9331=CARTESIAN_POINT('Ctrl Pts',(12.9181650995967,-13.7246099871303,7.));
#9332=CARTESIAN_POINT('Ctrl Pts',(13.07682262797,-13.7839294091566,7.));
#9333=CARTESIAN_POINT('',(13.7839294091565,-13.0768226279701,7.));
#9334=CARTESIAN_POINT('Origin',(0.,1.10390771809154E-15,7.));
#9335=CARTESIAN_POINT('',(12.5020870932787,-10.3807667497191,7.));
#9336=CARTESIAN_POINT('Ctrl Pts',(13.7839294091565,-13.0768226279701,7.));
#9337=CARTESIAN_POINT('Ctrl Pts',(13.7246099871302,-12.9181650995967,7.));
#9338=CARTESIAN_POINT('Ctrl Pts',(13.6262277632565,-12.6769008431476,7.));
#9339=CARTESIAN_POINT('Ctrl Pts',(13.4801075753502,-12.3652241842034,7.));
#9340=CARTESIAN_POINT('Ctrl Pts',(13.3650363045723,-12.1418243205134,7.));
#9341=CARTESIAN_POINT('Ctrl Pts',(13.2524512620508,-11.9419026340297,7.));
#9342=CARTESIAN_POINT('Ctrl Pts',(13.1439278991698,-11.764937382884,7.));
#9343=CARTESIAN_POINT('Ctrl Pts',(13.0410085154728,-11.6103189008825,7.));
#9344=CARTESIAN_POINT('Ctrl Pts',(12.9451853450404,-11.4773649257318,7.));
#9345=CARTESIAN_POINT('Ctrl Pts',(12.8579347093876,-11.3652836809863,7.));
#9346=CARTESIAN_POINT('Ctrl Pts',(12.7805989445416,-11.2732934467515,7.));
#9347=CARTESIAN_POINT('Ctrl Pts',(12.7212344815888,-11.2075126722099,7.));
#9348=CARTESIAN_POINT('Ctrl Pts',(12.6790250171322,-11.1639734745885,7.));
#9349=CARTESIAN_POINT('Ctrl Pts',(12.6515210644081,-11.1352828524076,7.));
#9350=CARTESIAN_POINT('Ctrl Pts',(12.6276288804813,-11.108827169799,7.));
#9351=CARTESIAN_POINT('Ctrl Pts',(12.5901836766158,-11.0652195671547,7.));
#9352=CARTESIAN_POINT('Ctrl Pts',(12.5420886163255,-11.0025423202231,7.));
#9353=CARTESIAN_POINT('Ctrl Pts',(12.48870543503,-10.9159571406243,7.));
#9354=CARTESIAN_POINT('Ctrl Pts',(12.4453471106188,-10.8193387993863,7.));
#9355=CARTESIAN_POINT('Ctrl Pts',(12.4165774110367,-10.7047117573306,7.));
#9356=CARTESIAN_POINT('Ctrl Pts',(12.4158793808611,-10.5490671691512,7.));
#9357=CARTESIAN_POINT('Ctrl Pts',(12.4613202473788,-10.4380033085876,7.));
#9358=CARTESIAN_POINT('Ctrl Pts',(12.5020870932787,-10.3807667497191,7.));
#9359=CARTESIAN_POINT('',(13.7360532384392,-8.68235805704669,7.));
#9360=CARTESIAN_POINT('Origin',(0.,0.,7.));
#9361=CARTESIAN_POINT('',(16.6962658094608,-9.06833546026116,7.));
#9362=CARTESIAN_POINT('Ctrl Pts',(13.7360532384392,-8.68235805704669,7.));
#9363=CARTESIAN_POINT('Ctrl Pts',(13.7778907925313,-8.62589941321482,7.));
#9364=CARTESIAN_POINT('Ctrl Pts',(13.8694768008521,-8.54836196063209,7.));
#9365=CARTESIAN_POINT('Ctrl Pts',(14.0177193038531,-8.50092900394922,7.));
#9366=CARTESIAN_POINT('Ctrl Pts',(14.1356264252377,-8.49286891019844,7.));
#9367=CARTESIAN_POINT('Ctrl Pts',(14.2409143873564,-8.50424841775457,7.));
#9368=CARTESIAN_POINT('Ctrl Pts',(14.3397580968626,-8.52826254822916,7.));
#9369=CARTESIAN_POINT('Ctrl Pts',(14.4142298919554,-8.55463533425733,7.));
#9370=CARTESIAN_POINT('Ctrl Pts',(14.4672743909627,-8.57677234909657,7.));
#9371=CARTESIAN_POINT('Ctrl Pts',(14.4998183311667,-8.59131991078477,7.));
#9372=CARTESIAN_POINT('Ctrl Pts',(14.5356039231527,-8.6086118344139,7.));
#9373=CARTESIAN_POINT('Ctrl Pts',(14.5900556026053,-8.63530106864818,7.));
#9374=CARTESIAN_POINT('Ctrl Pts',(14.6709614647944,-8.67143265073928,7.));
#9375=CARTESIAN_POINT('Ctrl Pts',(14.7823474421092,-8.71655678814373,7.));
#9376=CARTESIAN_POINT('Ctrl Pts',(14.9159049694657,-8.7649020643551,7.));
#9377=CARTESIAN_POINT('Ctrl Pts',(15.0719627020186,-8.81495027721557,7.));
#9378=CARTESIAN_POINT('Ctrl Pts',(15.2508174554788,-8.86505268915084,7.));
#9379=CARTESIAN_POINT('Ctrl Pts',(15.4526569741556,-8.91357927057117,7.));
#9380=CARTESIAN_POINT('Ctrl Pts',(15.6775844882862,-8.95887481023116,7.));
#9381=CARTESIAN_POINT('Ctrl Pts',(15.9256093626227,-8.99927973772153,7.));
#9382=CARTESIAN_POINT('Ctrl Pts',(16.2671851013731,-9.04193491022831,7.));
#9383=CARTESIAN_POINT('Ctrl Pts',(16.5270428237395,-9.06094720995305,7.));
#9384=CARTESIAN_POINT('Ctrl Pts',(16.6962658094608,-9.06833546026116,7.));
#9385=CARTESIAN_POINT('',(17.1502563092003,-8.17732893607285,7.));
#9386=CARTESIAN_POINT('Origin',(0.,0.,7.));
#9387=CARTESIAN_POINT('',(15.0980247376579,-6.00933848448159,7.));
#9388=CARTESIAN_POINT('Ctrl Pts',(17.1502563092003,-8.17732893607285,7.));
#9389=CARTESIAN_POINT('Ctrl Pts',(17.0448123137865,-8.04476736935674,7.));
#9390=CARTESIAN_POINT('Ctrl Pts',(16.8766905033057,-7.84571320523309,7.));
#9391=CARTESIAN_POINT('Ctrl Pts',(16.6414085620714,-7.59444470905136,7.));
#9392=CARTESIAN_POINT('Ctrl Pts',(16.4629349257385,-7.41753779118421,7.));
#9393=CARTESIAN_POINT('Ctrl Pts',(16.2940809887434,-7.26219165995679,7.));
#9394=CARTESIAN_POINT('Ctrl Pts',(16.1361838672874,-7.12742326811383,7.));
#9395=CARTESIAN_POINT('Ctrl Pts',(15.9905219781863,-7.01217619187962,7.));
#9396=CARTESIAN_POINT('Ctrl Pts',(15.8583036897433,-6.91534043556369,7.));
#9397=CARTESIAN_POINT('Ctrl Pts',(15.7406883947777,-6.83570676658069,7.));
#9398=CARTESIAN_POINT('Ctrl Pts',(15.6387111659832,-6.77211692048663,7.));
#9399=CARTESIAN_POINT('Ctrl Pts',(15.5619248294191,-6.72790031412624,7.));
#9400=CARTESIAN_POINT('Ctrl Pts',(15.5083268912119,-6.69953551835472,7.));
#9401=CARTESIAN_POINT('Ctrl Pts',(15.4733031879166,-6.68074830397725,7.));
#9402=CARTESIAN_POINT('Ctrl Pts',(15.4424051151807,-6.66297054550541,7.));
#9403=CARTESIAN_POINT('Ctrl Pts',(15.3933171197393,-6.63306845520276,7.));
#9404=CARTESIAN_POINT('Ctrl Pts',(15.3282076647862,-6.58832104206022,7.));
#9405=CARTESIAN_POINT('Ctrl Pts',(15.2506809503975,-6.52246995302226,7.));
#9406=CARTESIAN_POINT('Ctrl Pts',(15.1795880240196,-6.44397890908496,7.));
#9407=CARTESIAN_POINT('Ctrl Pts',(15.1168047097501,-6.34385243988822,7.));
#9408=CARTESIAN_POINT('Ctrl Pts',(15.0680440207731,-6.1960413432609,7.));
#9409=CARTESIAN_POINT('Ctrl Pts',(15.0769402326058,-6.07637133495394,7.));
#9410=CARTESIAN_POINT('Ctrl Pts',(15.0980247376579,-6.00933848448159,7.));
#9411=CARTESIAN_POINT('',(15.7467591314704,-4.01273932064523,7.));
#9412=CARTESIAN_POINT('Origin',(0.,0.,7.));
#9413=CARTESIAN_POINT('',(18.6813621637973,-3.46506965370701,7.));
#9414=CARTESIAN_POINT('Ctrl Pts',(15.7467591314704,-4.01273932064523,7.));
#9415=CARTESIAN_POINT('Ctrl Pts',(15.7691023294921,-3.94611544431022,7.));
#9416=CARTESIAN_POINT('Ctrl Pts',(15.8322454089585,-3.8440713117564,7.));
#9417=CARTESIAN_POINT('Ctrl Pts',(15.958574817721,-3.75315043650002,7.));
#9418=CARTESIAN_POINT('Ctrl Pts',(16.0682204478862,-3.70904952755073,7.));
#9419=CARTESIAN_POINT('Ctrl Pts',(16.1718717115691,-3.68733631276642,7.));
#9420=CARTESIAN_POINT('Ctrl Pts',(16.2732984400115,-3.67963072201298,7.));
#9421=CARTESIAN_POINT('Ctrl Pts',(16.3522749650865,-3.68169968173262,7.));
#9422=CARTESIAN_POINT('Ctrl Pts',(16.409563995311,-3.68636158229546,7.));
#9423=CARTESIAN_POINT('Ctrl Pts',(16.4450105654963,-3.69014050504826,7.));
#9424=CARTESIAN_POINT('Ctrl Pts',(16.4843881842109,-3.6955277456176,7.));
#9425=CARTESIAN_POINT('Ctrl Pts',(16.5444222357228,-3.70408422142792,7.));
#9426=CARTESIAN_POINT('Ctrl Pts',(16.632533556064,-3.71344611165872,7.));
#9427=CARTESIAN_POINT('Ctrl Pts',(16.7524120409277,-3.72194155665406,7.));
#9428=CARTESIAN_POINT('Ctrl Pts',(16.8943723095674,-3.72664910094713,7.));
#9429=CARTESIAN_POINT('Ctrl Pts',(17.0582577813421,-3.72602328845455,7.));
#9430=CARTESIAN_POINT('Ctrl Pts',(17.2438412568379,-3.71840435546376,7.));
#9431=CARTESIAN_POINT('Ctrl Pts',(17.4507975846592,-3.70218403552949,7.));
#9432=CARTESIAN_POINT('Ctrl Pts',(17.6787134541915,-3.67575622931335,7.));
#9433=CARTESIAN_POINT('Ctrl Pts',(17.9270849363835,-3.63753969769582,7.));
#9434=CARTESIAN_POINT('Ctrl Pts',(18.265123941733,-3.57255446932205,7.));
#9435=CARTESIAN_POINT('Ctrl Pts',(18.5181384456163,-3.51033578853422,7.));
#9436=CARTESIAN_POINT('Ctrl Pts',(18.6813621637973,-3.46506965370701,7.));
#9437=CARTESIAN_POINT('',(18.8377966288376,-2.47738131311191,7.));
#9438=CARTESIAN_POINT('Origin',(0.,0.,7.));
#9439=CARTESIAN_POINT('',(16.2160625265911,-1.04967429885982,7.));
#9440=CARTESIAN_POINT('Ctrl Pts',(18.8377966288376,-2.47738131311191,7.));
#9441=CARTESIAN_POINT('Ctrl Pts',(18.6965496529788,-2.38389175781396,7.));
#9442=CARTESIAN_POINT('Ctrl Pts',(18.4751451900744,-2.24653249449211,7.));
#9443=CARTESIAN_POINT('Ctrl Pts',(18.1737325312257,-2.08026807216974,7.));
#9444=CARTESIAN_POINT('Ctrl Pts',(17.949326772361,-1.96717098182924,7.));
#9445=CARTESIAN_POINT('Ctrl Pts',(17.7407325407201,-1.87160676754275,7.));
#9446=CARTESIAN_POINT('Ctrl Pts',(17.548917731071,-1.7922273041827,7.));
#9447=CARTESIAN_POINT('Ctrl Pts',(17.3747717371572,-1.72763282051117,7.));
#9448=CARTESIAN_POINT('Ctrl Pts',(17.2191007779952,-1.67639424155261,7.));
#9449=CARTESIAN_POINT('Ctrl Pts',(17.0826338282621,-1.6370032466926,7.));
#9450=CARTESIAN_POINT('Ctrl Pts',(16.9659973771906,-1.60803840593143,7.));
#9451=CARTESIAN_POINT('Ctrl Pts',(16.8793055486399,-1.58971419725802,7.));
#9452=CARTESIAN_POINT('Ctrl Pts',(16.8195656763126,-1.57930034717563,7.));
#9453=CARTESIAN_POINT('Ctrl Pts',(16.7804505865492,-1.57225556404309,7.));
#9454=CARTESIAN_POINT('Ctrl Pts',(16.7455711436431,-1.56489594057215,7.));
#9455=CARTESIAN_POINT('Ctrl Pts',(16.6896454316358,-1.55162638755015,7.));
#9456=CARTESIAN_POINT('Ctrl Pts',(16.6138949491149,-1.5291889967686,7.));
#9457=CARTESIAN_POINT('Ctrl Pts',(16.5198135565977,-1.49051796169807,7.));
#9458=CARTESIAN_POINT('Ctrl Pts',(16.4279450992207,-1.43783746532129,7.));
#9459=CARTESIAN_POINT('Ctrl Pts',(16.3372938385016,-1.36201264541057,7.));
#9460=CARTESIAN_POINT('Ctrl Pts',(16.2452435266959,-1.23650382033374,7.));
#9461=CARTESIAN_POINT('Ctrl Pts',(16.2167242606458,-1.11994179848647,7.));
#9462=CARTESIAN_POINT('Ctrl Pts',(16.2160625265911,-1.04967429885982,7.));
#9463=CARTESIAN_POINT('',(16.2160625265911,1.0496742988598,7.));
#9464=CARTESIAN_POINT('Origin',(0.,0.,7.));
#9465=CARTESIAN_POINT('',(18.8377966288376,2.47738131311188,7.));
#9466=CARTESIAN_POINT('Ctrl Pts',(16.2160625265911,1.0496742988598,7.));
#9467=CARTESIAN_POINT('Ctrl Pts',(16.2167242606459,1.11994179848647,7.));
#9468=CARTESIAN_POINT('Ctrl Pts',(16.2452435266959,1.23650382033374,7.));
#9469=CARTESIAN_POINT('Ctrl Pts',(16.3372938385016,1.36201264541054,7.));
#9470=CARTESIAN_POINT('Ctrl Pts',(16.4279450992208,1.43783746532129,7.));
#9471=CARTESIAN_POINT('Ctrl Pts',(16.5198135565978,1.49051796169809,7.));
#9472=CARTESIAN_POINT('Ctrl Pts',(16.6138949491149,1.52918899676861,7.));
#9473=CARTESIAN_POINT('Ctrl Pts',(16.6896454316359,1.55162638755015,7.));
#9474=CARTESIAN_POINT('Ctrl Pts',(16.7455711436431,1.56489594057217,7.));
#9475=CARTESIAN_POINT('Ctrl Pts',(16.7804505865492,1.57225556404311,7.));
#9476=CARTESIAN_POINT('Ctrl Pts',(16.8195656763126,1.57930034717561,7.));
#9477=CARTESIAN_POINT('Ctrl Pts',(16.8793055486399,1.58971419725803,7.));
#9478=CARTESIAN_POINT('Ctrl Pts',(16.9659973771906,1.60803840593143,7.));
#9479=CARTESIAN_POINT('Ctrl Pts',(17.0826338282621,1.63700324669259,7.));
#9480=CARTESIAN_POINT('Ctrl Pts',(17.2191007779953,1.67639424155262,7.));
#9481=CARTESIAN_POINT('Ctrl Pts',(17.3747717371572,1.7276328205112,7.));
#9482=CARTESIAN_POINT('Ctrl Pts',(17.548917731071,1.79222730418268,7.));
#9483=CARTESIAN_POINT('Ctrl Pts',(17.7407325407201,1.87160676754277,7.));
#9484=CARTESIAN_POINT('Ctrl Pts',(17.949326772361,1.96717098182924,7.));
#9485=CARTESIAN_POINT('Ctrl Pts',(18.1737325312257,2.08026807216972,7.));
#9486=CARTESIAN_POINT('Ctrl Pts',(18.4751451900744,2.2465324944921,7.));
#9487=CARTESIAN_POINT('Ctrl Pts',(18.6965496529788,2.38389175781394,7.));
#9488=CARTESIAN_POINT('Ctrl Pts',(18.8377966288376,2.47738131311188,7.));
#9489=CARTESIAN_POINT('',(18.6813621637973,3.46506965370699,7.));
#9490=CARTESIAN_POINT('Origin',(1.73472347597681E-15,0.,7.));
#9491=CARTESIAN_POINT('',(15.7467591314704,4.01273932064524,7.));
#9492=CARTESIAN_POINT('Ctrl Pts',(18.6813621637973,3.46506965370699,7.));
#9493=CARTESIAN_POINT('Ctrl Pts',(18.5181384456162,3.51033578853419,7.));
#9494=CARTESIAN_POINT('Ctrl Pts',(18.2651239417329,3.57255446932204,7.));
#9495=CARTESIAN_POINT('Ctrl Pts',(17.9270849363835,3.63753969769579,7.));
#9496=CARTESIAN_POINT('Ctrl Pts',(17.6787134541915,3.67575622931334,7.));
#9497=CARTESIAN_POINT('Ctrl Pts',(17.4507975846592,3.70218403552951,7.));
#9498=CARTESIAN_POINT('Ctrl Pts',(17.2438412568379,3.71840435546372,7.));
#9499=CARTESIAN_POINT('Ctrl Pts',(17.0582577813421,3.72602328845457,7.));
#9500=CARTESIAN_POINT('Ctrl Pts',(16.8943723095674,3.72664910094712,7.));
#9501=CARTESIAN_POINT('Ctrl Pts',(16.7524120409277,3.72194155665404,7.));
#9502=CARTESIAN_POINT('Ctrl Pts',(16.632533556064,3.71344611165872,7.));
#9503=CARTESIAN_POINT('Ctrl Pts',(16.5444222357228,3.70408422142792,7.));
#9504=CARTESIAN_POINT('Ctrl Pts',(16.4843881842109,3.69552774561757,7.));
#9505=CARTESIAN_POINT('Ctrl Pts',(16.4450105654963,3.69014050504827,7.));
#9506=CARTESIAN_POINT('Ctrl Pts',(16.409563995311,3.68636158229547,7.));
#9507=CARTESIAN_POINT('Ctrl Pts',(16.3522749650865,3.68169968173261,7.));
#9508=CARTESIAN_POINT('Ctrl Pts',(16.2732984400115,3.67963072201297,7.));
#9509=CARTESIAN_POINT('Ctrl Pts',(16.1718717115691,3.68733631276642,7.));
#9510=CARTESIAN_POINT('Ctrl Pts',(16.0682204478862,3.70904952755071,7.));
#9511=CARTESIAN_POINT('Ctrl Pts',(15.958574817721,3.75315043649999,7.));
#9512=CARTESIAN_POINT('Ctrl Pts',(15.8322454089585,3.84407131175639,7.));
#9513=CARTESIAN_POINT('Ctrl Pts',(15.7691023294921,3.94611544431022,7.));
#9514=CARTESIAN_POINT('Ctrl Pts',(15.7467591314704,4.01273932064524,7.));
#9515=CARTESIAN_POINT('Origin',(0.,0.,7.));
#9516=CARTESIAN_POINT('Origin',(16.0675296603332,7.07348467874013,0.));
#9517=CARTESIAN_POINT('',(15.0980247376579,6.00933848448158,0.));
#9518=CARTESIAN_POINT('',(17.1502563092004,8.17732893607278,0.));
#9519=CARTESIAN_POINT('Ctrl Pts',(15.0980247376579,6.00933848448158,0.));
#9520=CARTESIAN_POINT('Ctrl Pts',(15.0769402326058,6.07637133495396,0.));
#9521=CARTESIAN_POINT('Ctrl Pts',(15.0680440207731,6.1960413432609,0.));
#9522=CARTESIAN_POINT('Ctrl Pts',(15.1168047097502,6.34385243988821,0.));
#9523=CARTESIAN_POINT('Ctrl Pts',(15.1795880240196,6.44397890908497,0.));
#9524=CARTESIAN_POINT('Ctrl Pts',(15.2506809503975,6.52246995302229,0.));
#9525=CARTESIAN_POINT('Ctrl Pts',(15.3282076647862,6.58832104206024,0.));
#9526=CARTESIAN_POINT('Ctrl Pts',(15.3933171197393,6.63306845520277,0.));
#9527=CARTESIAN_POINT('Ctrl Pts',(15.4424051151807,6.66297054550544,0.));
#9528=CARTESIAN_POINT('Ctrl Pts',(15.4733031879166,6.68074830397728,0.));
#9529=CARTESIAN_POINT('Ctrl Pts',(15.5083268912119,6.69953551835471,0.));
#9530=CARTESIAN_POINT('Ctrl Pts',(15.5619248294191,6.72790031412625,0.));
#9531=CARTESIAN_POINT('Ctrl Pts',(15.6387111659832,6.77211692048664,0.));
#9532=CARTESIAN_POINT('Ctrl Pts',(15.7406883947778,6.83570676658069,0.));
#9533=CARTESIAN_POINT('Ctrl Pts',(15.8583036897433,6.91534043556371,0.));
#9534=CARTESIAN_POINT('Ctrl Pts',(15.9905219781863,7.01217619187965,0.));
#9535=CARTESIAN_POINT('Ctrl Pts',(16.1361838672874,7.12742326811382,0.));
#9536=CARTESIAN_POINT('Ctrl Pts',(16.2940809887434,7.2621916599568,0.));
#9537=CARTESIAN_POINT('Ctrl Pts',(16.4629349257385,7.41753779118422,0.));
#9538=CARTESIAN_POINT('Ctrl Pts',(16.6414085620714,7.59444470905136,0.));
#9539=CARTESIAN_POINT('Ctrl Pts',(16.8766905033057,7.84571320523309,0.));
#9540=CARTESIAN_POINT('Ctrl Pts',(17.0448123137865,8.04476736935674,0.));
#9541=CARTESIAN_POINT('Ctrl Pts',(17.1502563092004,8.17732893607278,0.));
#9542=CARTESIAN_POINT('',(15.7467591314704,4.01273932064524,0.));
#9543=CARTESIAN_POINT('Origin',(0.,0.,0.));
#9544=CARTESIAN_POINT('',(18.6813621637973,3.46506965370699,0.));
#9545=CARTESIAN_POINT('Ctrl Pts',(18.6813621637973,3.46506965370699,0.));
#9546=CARTESIAN_POINT('Ctrl Pts',(18.5181384456162,3.51033578853419,0.));
#9547=CARTESIAN_POINT('Ctrl Pts',(18.2651239417329,3.57255446932204,0.));
#9548=CARTESIAN_POINT('Ctrl Pts',(17.9270849363835,3.63753969769579,0.));
#9549=CARTESIAN_POINT('Ctrl Pts',(17.6787134541915,3.67575622931334,0.));
#9550=CARTESIAN_POINT('Ctrl Pts',(17.4507975846592,3.70218403552951,0.));
#9551=CARTESIAN_POINT('Ctrl Pts',(17.2438412568379,3.71840435546372,0.));
#9552=CARTESIAN_POINT('Ctrl Pts',(17.0582577813421,3.72602328845457,0.));
#9553=CARTESIAN_POINT('Ctrl Pts',(16.8943723095674,3.72664910094712,0.));
#9554=CARTESIAN_POINT('Ctrl Pts',(16.7524120409277,3.72194155665404,0.));
#9555=CARTESIAN_POINT('Ctrl Pts',(16.632533556064,3.71344611165872,0.));
#9556=CARTESIAN_POINT('Ctrl Pts',(16.5444222357228,3.70408422142792,0.));
#9557=CARTESIAN_POINT('Ctrl Pts',(16.4843881842109,3.69552774561757,0.));
#9558=CARTESIAN_POINT('Ctrl Pts',(16.4450105654963,3.69014050504827,0.));
#9559=CARTESIAN_POINT('Ctrl Pts',(16.409563995311,3.68636158229547,0.));
#9560=CARTESIAN_POINT('Ctrl Pts',(16.3522749650865,3.68169968173261,0.));
#9561=CARTESIAN_POINT('Ctrl Pts',(16.2732984400115,3.67963072201297,0.));
#9562=CARTESIAN_POINT('Ctrl Pts',(16.1718717115691,3.68733631276642,0.));
#9563=CARTESIAN_POINT('Ctrl Pts',(16.0682204478862,3.70904952755071,0.));
#9564=CARTESIAN_POINT('Ctrl Pts',(15.958574817721,3.75315043649999,0.));
#9565=CARTESIAN_POINT('Ctrl Pts',(15.8322454089585,3.84407131175639,0.));
#9566=CARTESIAN_POINT('Ctrl Pts',(15.7691023294921,3.94611544431022,0.));
#9567=CARTESIAN_POINT('Ctrl Pts',(15.7467591314704,4.01273932064524,0.));
#9568=CARTESIAN_POINT('',(18.8377966288376,2.47738131311188,0.));
#9569=CARTESIAN_POINT('Origin',(1.73472347597681E-15,0.,0.));
#9570=CARTESIAN_POINT('',(16.2160625265911,1.0496742988598,0.));
#9571=CARTESIAN_POINT('Ctrl Pts',(16.2160625265911,1.0496742988598,0.));
#9572=CARTESIAN_POINT('Ctrl Pts',(16.2167242606459,1.11994179848647,0.));
#9573=CARTESIAN_POINT('Ctrl Pts',(16.2452435266959,1.23650382033374,0.));
#9574=CARTESIAN_POINT('Ctrl Pts',(16.3372938385016,1.36201264541054,0.));
#9575=CARTESIAN_POINT('Ctrl Pts',(16.4279450992208,1.43783746532129,0.));
#9576=CARTESIAN_POINT('Ctrl Pts',(16.5198135565978,1.49051796169809,0.));
#9577=CARTESIAN_POINT('Ctrl Pts',(16.6138949491149,1.52918899676861,0.));
#9578=CARTESIAN_POINT('Ctrl Pts',(16.6896454316359,1.55162638755015,0.));
#9579=CARTESIAN_POINT('Ctrl Pts',(16.7455711436431,1.56489594057217,0.));
#9580=CARTESIAN_POINT('Ctrl Pts',(16.7804505865492,1.57225556404311,0.));
#9581=CARTESIAN_POINT('Ctrl Pts',(16.8195656763126,1.57930034717561,0.));
#9582=CARTESIAN_POINT('Ctrl Pts',(16.8793055486399,1.58971419725803,0.));
#9583=CARTESIAN_POINT('Ctrl Pts',(16.9659973771906,1.60803840593143,0.));
#9584=CARTESIAN_POINT('Ctrl Pts',(17.0826338282621,1.63700324669259,0.));
#9585=CARTESIAN_POINT('Ctrl Pts',(17.2191007779953,1.67639424155262,0.));
#9586=CARTESIAN_POINT('Ctrl Pts',(17.3747717371572,1.7276328205112,0.));
#9587=CARTESIAN_POINT('Ctrl Pts',(17.548917731071,1.79222730418268,0.));
#9588=CARTESIAN_POINT('Ctrl Pts',(17.7407325407201,1.87160676754277,0.));
#9589=CARTESIAN_POINT('Ctrl Pts',(17.949326772361,1.96717098182924,0.));
#9590=CARTESIAN_POINT('Ctrl Pts',(18.1737325312257,2.08026807216972,0.));
#9591=CARTESIAN_POINT('Ctrl Pts',(18.4751451900744,2.2465324944921,0.));
#9592=CARTESIAN_POINT('Ctrl Pts',(18.6965496529788,2.38389175781394,0.));
#9593=CARTESIAN_POINT('Ctrl Pts',(18.8377966288376,2.47738131311188,0.));
#9594=CARTESIAN_POINT('',(16.2160625265911,-1.04967429885982,0.));
#9595=CARTESIAN_POINT('Origin',(0.,0.,0.));
#9596=CARTESIAN_POINT('',(18.8377966288376,-2.47738131311191,0.));
#9597=CARTESIAN_POINT('Ctrl Pts',(18.8377966288376,-2.47738131311191,0.));
#9598=CARTESIAN_POINT('Ctrl Pts',(18.6965496529788,-2.38389175781396,0.));
#9599=CARTESIAN_POINT('Ctrl Pts',(18.4751451900744,-2.24653249449211,0.));
#9600=CARTESIAN_POINT('Ctrl Pts',(18.1737325312257,-2.08026807216974,0.));
#9601=CARTESIAN_POINT('Ctrl Pts',(17.949326772361,-1.96717098182924,0.));
#9602=CARTESIAN_POINT('Ctrl Pts',(17.7407325407201,-1.87160676754275,0.));
#9603=CARTESIAN_POINT('Ctrl Pts',(17.548917731071,-1.7922273041827,0.));
#9604=CARTESIAN_POINT('Ctrl Pts',(17.3747717371572,-1.72763282051117,0.));
#9605=CARTESIAN_POINT('Ctrl Pts',(17.2191007779952,-1.67639424155261,0.));
#9606=CARTESIAN_POINT('Ctrl Pts',(17.0826338282621,-1.6370032466926,0.));
#9607=CARTESIAN_POINT('Ctrl Pts',(16.9659973771906,-1.60803840593143,0.));
#9608=CARTESIAN_POINT('Ctrl Pts',(16.8793055486399,-1.58971419725802,0.));
#9609=CARTESIAN_POINT('Ctrl Pts',(16.8195656763126,-1.57930034717563,0.));
#9610=CARTESIAN_POINT('Ctrl Pts',(16.7804505865492,-1.57225556404309,0.));
#9611=CARTESIAN_POINT('Ctrl Pts',(16.7455711436431,-1.56489594057215,0.));
#9612=CARTESIAN_POINT('Ctrl Pts',(16.6896454316358,-1.55162638755015,0.));
#9613=CARTESIAN_POINT('Ctrl Pts',(16.6138949491149,-1.5291889967686,0.));
#9614=CARTESIAN_POINT('Ctrl Pts',(16.5198135565977,-1.49051796169807,0.));
#9615=CARTESIAN_POINT('Ctrl Pts',(16.4279450992207,-1.43783746532129,0.));
#9616=CARTESIAN_POINT('Ctrl Pts',(16.3372938385016,-1.36201264541057,0.));
#9617=CARTESIAN_POINT('Ctrl Pts',(16.2452435266959,-1.23650382033374,0.));
#9618=CARTESIAN_POINT('Ctrl Pts',(16.2167242606458,-1.11994179848647,0.));
#9619=CARTESIAN_POINT('Ctrl Pts',(16.2160625265911,-1.04967429885982,0.));
#9620=CARTESIAN_POINT('',(18.6813621637973,-3.46506965370701,0.));
#9621=CARTESIAN_POINT('Origin',(0.,0.,0.));
#9622=CARTESIAN_POINT('',(15.7467591314704,-4.01273932064523,0.));
#9623=CARTESIAN_POINT('Ctrl Pts',(15.7467591314704,-4.01273932064523,0.));
#9624=CARTESIAN_POINT('Ctrl Pts',(15.7691023294921,-3.94611544431022,0.));
#9625=CARTESIAN_POINT('Ctrl Pts',(15.8322454089585,-3.8440713117564,0.));
#9626=CARTESIAN_POINT('Ctrl Pts',(15.958574817721,-3.75315043650002,0.));
#9627=CARTESIAN_POINT('Ctrl Pts',(16.0682204478862,-3.70904952755073,0.));
#9628=CARTESIAN_POINT('Ctrl Pts',(16.1718717115691,-3.68733631276642,0.));
#9629=CARTESIAN_POINT('Ctrl Pts',(16.2732984400115,-3.67963072201298,0.));
#9630=CARTESIAN_POINT('Ctrl Pts',(16.3522749650865,-3.68169968173262,0.));
#9631=CARTESIAN_POINT('Ctrl Pts',(16.409563995311,-3.68636158229546,0.));
#9632=CARTESIAN_POINT('Ctrl Pts',(16.4450105654963,-3.69014050504826,0.));
#9633=CARTESIAN_POINT('Ctrl Pts',(16.4843881842109,-3.6955277456176,0.));
#9634=CARTESIAN_POINT('Ctrl Pts',(16.5444222357228,-3.70408422142792,0.));
#9635=CARTESIAN_POINT('Ctrl Pts',(16.632533556064,-3.71344611165872,0.));
#9636=CARTESIAN_POINT('Ctrl Pts',(16.7524120409277,-3.72194155665406,0.));
#9637=CARTESIAN_POINT('Ctrl Pts',(16.8943723095674,-3.72664910094713,0.));
#9638=CARTESIAN_POINT('Ctrl Pts',(17.0582577813421,-3.72602328845455,0.));
#9639=CARTESIAN_POINT('Ctrl Pts',(17.2438412568379,-3.71840435546376,0.));
#9640=CARTESIAN_POINT('Ctrl Pts',(17.4507975846592,-3.70218403552949,0.));
#9641=CARTESIAN_POINT('Ctrl Pts',(17.6787134541915,-3.67575622931335,0.));
#9642=CARTESIAN_POINT('Ctrl Pts',(17.9270849363835,-3.63753969769582,0.));
#9643=CARTESIAN_POINT('Ctrl Pts',(18.265123941733,-3.57255446932205,0.));
#9644=CARTESIAN_POINT('Ctrl Pts',(18.5181384456163,-3.51033578853422,0.));
#9645=CARTESIAN_POINT('Ctrl Pts',(18.6813621637973,-3.46506965370701,0.));
#9646=CARTESIAN_POINT('',(15.0980247376579,-6.00933848448159,0.));
#9647=CARTESIAN_POINT('Origin',(0.,0.,0.));
#9648=CARTESIAN_POINT('',(17.1502563092003,-8.17732893607285,0.));
#9649=CARTESIAN_POINT('Ctrl Pts',(17.1502563092003,-8.17732893607285,0.));
#9650=CARTESIAN_POINT('Ctrl Pts',(17.0448123137865,-8.04476736935674,0.));
#9651=CARTESIAN_POINT('Ctrl Pts',(16.8766905033057,-7.84571320523309,0.));
#9652=CARTESIAN_POINT('Ctrl Pts',(16.6414085620714,-7.59444470905136,0.));
#9653=CARTESIAN_POINT('Ctrl Pts',(16.4629349257385,-7.41753779118421,0.));
#9654=CARTESIAN_POINT('Ctrl Pts',(16.2940809887434,-7.26219165995679,0.));
#9655=CARTESIAN_POINT('Ctrl Pts',(16.1361838672874,-7.12742326811383,0.));
#9656=CARTESIAN_POINT('Ctrl Pts',(15.9905219781863,-7.01217619187962,0.));
#9657=CARTESIAN_POINT('Ctrl Pts',(15.8583036897433,-6.91534043556369,0.));
#9658=CARTESIAN_POINT('Ctrl Pts',(15.7406883947777,-6.83570676658069,0.));
#9659=CARTESIAN_POINT('Ctrl Pts',(15.6387111659832,-6.77211692048663,0.));
#9660=CARTESIAN_POINT('Ctrl Pts',(15.5619248294191,-6.72790031412624,0.));
#9661=CARTESIAN_POINT('Ctrl Pts',(15.5083268912119,-6.69953551835472,0.));
#9662=CARTESIAN_POINT('Ctrl Pts',(15.4733031879166,-6.68074830397725,0.));
#9663=CARTESIAN_POINT('Ctrl Pts',(15.4424051151807,-6.66297054550541,0.));
#9664=CARTESIAN_POINT('Ctrl Pts',(15.3933171197393,-6.63306845520276,0.));
#9665=CARTESIAN_POINT('Ctrl Pts',(15.3282076647862,-6.58832104206022,0.));
#9666=CARTESIAN_POINT('Ctrl Pts',(15.2506809503975,-6.52246995302226,0.));
#9667=CARTESIAN_POINT('Ctrl Pts',(15.1795880240196,-6.44397890908496,0.));
#9668=CARTESIAN_POINT('Ctrl Pts',(15.1168047097501,-6.34385243988822,0.));
#9669=CARTESIAN_POINT('Ctrl Pts',(15.0680440207731,-6.1960413432609,0.));
#9670=CARTESIAN_POINT('Ctrl Pts',(15.0769402326058,-6.07637133495394,0.));
#9671=CARTESIAN_POINT('Ctrl Pts',(15.0980247376579,-6.00933848448159,0.));
#9672=CARTESIAN_POINT('',(16.6962658094608,-9.06833546026116,0.));
#9673=CARTESIAN_POINT('Origin',(0.,0.,0.));
#9674=CARTESIAN_POINT('',(13.7360532384392,-8.68235805704669,0.));
#9675=CARTESIAN_POINT('Ctrl Pts',(13.7360532384392,-8.68235805704669,0.));
#9676=CARTESIAN_POINT('Ctrl Pts',(13.7778907925313,-8.62589941321482,0.));
#9677=CARTESIAN_POINT('Ctrl Pts',(13.8694768008521,-8.54836196063209,0.));
#9678=CARTESIAN_POINT('Ctrl Pts',(14.0177193038531,-8.50092900394922,0.));
#9679=CARTESIAN_POINT('Ctrl Pts',(14.1356264252377,-8.49286891019844,0.));
#9680=CARTESIAN_POINT('Ctrl Pts',(14.2409143873564,-8.50424841775457,0.));
#9681=CARTESIAN_POINT('Ctrl Pts',(14.3397580968626,-8.52826254822916,0.));
#9682=CARTESIAN_POINT('Ctrl Pts',(14.4142298919554,-8.55463533425733,0.));
#9683=CARTESIAN_POINT('Ctrl Pts',(14.4672743909627,-8.57677234909657,0.));
#9684=CARTESIAN_POINT('Ctrl Pts',(14.4998183311667,-8.59131991078477,0.));
#9685=CARTESIAN_POINT('Ctrl Pts',(14.5356039231527,-8.6086118344139,0.));
#9686=CARTESIAN_POINT('Ctrl Pts',(14.5900556026053,-8.63530106864818,0.));
#9687=CARTESIAN_POINT('Ctrl Pts',(14.6709614647944,-8.67143265073928,0.));
#9688=CARTESIAN_POINT('Ctrl Pts',(14.7823474421092,-8.71655678814373,0.));
#9689=CARTESIAN_POINT('Ctrl Pts',(14.9159049694657,-8.7649020643551,0.));
#9690=CARTESIAN_POINT('Ctrl Pts',(15.0719627020186,-8.81495027721557,0.));
#9691=CARTESIAN_POINT('Ctrl Pts',(15.2508174554788,-8.86505268915084,0.));
#9692=CARTESIAN_POINT('Ctrl Pts',(15.4526569741556,-8.91357927057117,0.));
#9693=CARTESIAN_POINT('Ctrl Pts',(15.6775844882862,-8.95887481023116,0.));
#9694=CARTESIAN_POINT('Ctrl Pts',(15.9256093626227,-8.99927973772153,0.));
#9695=CARTESIAN_POINT('Ctrl Pts',(16.2671851013731,-9.04193491022831,0.));
#9696=CARTESIAN_POINT('Ctrl Pts',(16.5270428237395,-9.06094720995305,0.));
#9697=CARTESIAN_POINT('Ctrl Pts',(16.6962658094608,-9.06833546026116,0.));
#9698=CARTESIAN_POINT('',(12.5020870932787,-10.3807667497191,0.));
#9699=CARTESIAN_POINT('Origin',(0.,0.,0.));
#9700=CARTESIAN_POINT('',(13.7839294091565,-13.0768226279701,0.));
#9701=CARTESIAN_POINT('Ctrl Pts',(13.7839294091565,-13.0768226279701,0.));
#9702=CARTESIAN_POINT('Ctrl Pts',(13.7246099871302,-12.9181650995967,0.));
#9703=CARTESIAN_POINT('Ctrl Pts',(13.6262277632565,-12.6769008431476,0.));
#9704=CARTESIAN_POINT('Ctrl Pts',(13.4801075753502,-12.3652241842034,0.));
#9705=CARTESIAN_POINT('Ctrl Pts',(13.3650363045723,-12.1418243205134,0.));
#9706=CARTESIAN_POINT('Ctrl Pts',(13.2524512620508,-11.9419026340297,0.));
#9707=CARTESIAN_POINT('Ctrl Pts',(13.1439278991698,-11.764937382884,0.));
#9708=CARTESIAN_POINT('Ctrl Pts',(13.0410085154728,-11.6103189008825,0.));
#9709=CARTESIAN_POINT('Ctrl Pts',(12.9451853450404,-11.4773649257318,0.));
#9710=CARTESIAN_POINT('Ctrl Pts',(12.8579347093876,-11.3652836809863,0.));
#9711=CARTESIAN_POINT('Ctrl Pts',(12.7805989445416,-11.2732934467515,0.));
#9712=CARTESIAN_POINT('Ctrl Pts',(12.7212344815888,-11.2075126722099,0.));
#9713=CARTESIAN_POINT('Ctrl Pts',(12.6790250171322,-11.1639734745885,0.));
#9714=CARTESIAN_POINT('Ctrl Pts',(12.6515210644081,-11.1352828524076,0.));
#9715=CARTESIAN_POINT('Ctrl Pts',(12.6276288804813,-11.108827169799,0.));
#9716=CARTESIAN_POINT('Ctrl Pts',(12.5901836766158,-11.0652195671547,0.));
#9717=CARTESIAN_POINT('Ctrl Pts',(12.5420886163255,-11.0025423202231,0.));
#9718=CARTESIAN_POINT('Ctrl Pts',(12.48870543503,-10.9159571406243,0.));
#9719=CARTESIAN_POINT('Ctrl Pts',(12.4453471106188,-10.8193387993863,0.));
#9720=CARTESIAN_POINT('Ctrl Pts',(12.4165774110367,-10.7047117573306,0.));
#9721=CARTESIAN_POINT('Ctrl Pts',(12.4158793808611,-10.5490671691512,0.));
#9722=CARTESIAN_POINT('Ctrl Pts',(12.4613202473788,-10.4380033085876,0.));
#9723=CARTESIAN_POINT('Ctrl Pts',(12.5020870932787,-10.3807667497191,0.));
#9724=CARTESIAN_POINT('',(13.07682262797,-13.7839294091566,0.));
#9725=CARTESIAN_POINT('Origin',(0.,1.10390771809154E-15,0.));
#9726=CARTESIAN_POINT('',(10.3807667497191,-12.5020870932787,0.));
#9727=CARTESIAN_POINT('Ctrl Pts',(10.3807667497191,-12.5020870932787,0.));
#9728=CARTESIAN_POINT('Ctrl Pts',(10.4380033085876,-12.4613202473788,0.));
#9729=CARTESIAN_POINT('Ctrl Pts',(10.5490671691512,-12.4158793808611,0.));
#9730=CARTESIAN_POINT('Ctrl Pts',(10.7047117573306,-12.4165774110367,0.));
#9731=CARTESIAN_POINT('Ctrl Pts',(10.8193387993863,-12.4453471106188,0.));
#9732=CARTESIAN_POINT('Ctrl Pts',(10.9159571406243,-12.48870543503,0.));
#9733=CARTESIAN_POINT('Ctrl Pts',(11.0025423202231,-12.5420886163255,0.));
#9734=CARTESIAN_POINT('Ctrl Pts',(11.0652195671547,-12.5901836766158,0.));
#9735=CARTESIAN_POINT('Ctrl Pts',(11.1088271697991,-12.6276288804813,0.));
#9736=CARTESIAN_POINT('Ctrl Pts',(11.1352828524077,-12.651521064408,0.));
#9737=CARTESIAN_POINT('Ctrl Pts',(11.1639734745885,-12.6790250171322,0.));
#9738=CARTESIAN_POINT('Ctrl Pts',(11.2075126722099,-12.7212344815888,0.));
#9739=CARTESIAN_POINT('Ctrl Pts',(11.2732934467515,-12.7805989445416,0.));
#9740=CARTESIAN_POINT('Ctrl Pts',(11.3652836809863,-12.8579347093876,0.));
#9741=CARTESIAN_POINT('Ctrl Pts',(11.4773649257318,-12.9451853450404,0.));
#9742=CARTESIAN_POINT('Ctrl Pts',(11.6103189008825,-13.0410085154727,0.));
#9743=CARTESIAN_POINT('Ctrl Pts',(11.764937382884,-13.1439278991698,0.));
#9744=CARTESIAN_POINT('Ctrl Pts',(11.9419026340297,-13.2524512620507,0.));
#9745=CARTESIAN_POINT('Ctrl Pts',(12.1418243205134,-13.3650363045724,0.));
#9746=CARTESIAN_POINT('Ctrl Pts',(12.3652241842034,-13.4801075753502,0.));
#9747=CARTESIAN_POINT('Ctrl Pts',(12.6769008431476,-13.6262277632565,0.));
#9748=CARTESIAN_POINT('Ctrl Pts',(12.9181650995967,-13.7246099871303,0.));
#9749=CARTESIAN_POINT('Ctrl Pts',(13.07682262797,-13.7839294091566,0.));
#9750=CARTESIAN_POINT('',(8.68235805704667,-13.7360532384392,0.));
#9751=CARTESIAN_POINT('Origin',(0.,0.,0.));
#9752=CARTESIAN_POINT('',(9.06833546026109,-16.6962658094609,0.));
#9753=CARTESIAN_POINT('Ctrl Pts',(9.06833546026109,-16.6962658094609,0.));
#9754=CARTESIAN_POINT('Ctrl Pts',(9.06094720995301,-16.5270428237395,0.));
#9755=CARTESIAN_POINT('Ctrl Pts',(9.0419349102283,-16.267185101373,0.));
#9756=CARTESIAN_POINT('Ctrl Pts',(8.99927973772149,-15.9256093626227,0.));
#9757=CARTESIAN_POINT('Ctrl Pts',(8.95887481023114,-15.6775844882862,0.));
#9758=CARTESIAN_POINT('Ctrl Pts',(8.91357927057119,-15.4526569741556,0.));
#9759=CARTESIAN_POINT('Ctrl Pts',(8.8650526891508,-15.2508174554787,0.));
#9760=CARTESIAN_POINT('Ctrl Pts',(8.81495027721559,-15.0719627020186,0.));
#9761=CARTESIAN_POINT('Ctrl Pts',(8.76490206435508,-14.9159049694657,0.));
#9762=CARTESIAN_POINT('Ctrl Pts',(8.7165567881437,-14.7823474421092,0.));
#9763=CARTESIAN_POINT('Ctrl Pts',(8.67143265073927,-14.6709614647944,0.));
#9764=CARTESIAN_POINT('Ctrl Pts',(8.63530106864817,-14.5900556026053,0.));
#9765=CARTESIAN_POINT('Ctrl Pts',(8.60861183441386,-14.5356039231526,0.));
#9766=CARTESIAN_POINT('Ctrl Pts',(8.59131991078477,-14.4998183311667,0.));
#9767=CARTESIAN_POINT('Ctrl Pts',(8.57677234909656,-14.4672743909626,0.));
#9768=CARTESIAN_POINT('Ctrl Pts',(8.55463533425731,-14.4142298919554,0.));
#9769=CARTESIAN_POINT('Ctrl Pts',(8.52826254822914,-14.3397580968625,0.));
#9770=CARTESIAN_POINT('Ctrl Pts',(8.50424841775455,-14.2409143873564,0.));
#9771=CARTESIAN_POINT('Ctrl Pts',(8.49286891019841,-14.1356264252376,0.));
#9772=CARTESIAN_POINT('Ctrl Pts',(8.50092900394917,-14.0177193038531,0.));
#9773=CARTESIAN_POINT('Ctrl Pts',(8.54836196063206,-13.8694768008521,0.));
#9774=CARTESIAN_POINT('Ctrl Pts',(8.62589941321478,-13.7778907925312,0.));
#9775=CARTESIAN_POINT('Ctrl Pts',(8.68235805704667,-13.7360532384392,0.));
#9776=CARTESIAN_POINT('',(8.17732893607279,-17.1502563092004,0.));
#9777=CARTESIAN_POINT('Origin',(0.,0.,0.));
#9778=CARTESIAN_POINT('',(6.00933848448151,-15.0980247376579,0.));
#9779=CARTESIAN_POINT('Ctrl Pts',(6.00933848448151,-15.0980247376579,0.));
#9780=CARTESIAN_POINT('Ctrl Pts',(6.07637133495396,-15.0769402326058,0.));
#9781=CARTESIAN_POINT('Ctrl Pts',(6.1960413432609,-15.0680440207731,0.));
#9782=CARTESIAN_POINT('Ctrl Pts',(6.34385243988821,-15.1168047097502,0.));
#9783=CARTESIAN_POINT('Ctrl Pts',(6.44397890908497,-15.1795880240196,0.));
#9784=CARTESIAN_POINT('Ctrl Pts',(6.52246995302229,-15.2506809503975,0.));
#9785=CARTESIAN_POINT('Ctrl Pts',(6.58832104206024,-15.3282076647862,0.));
#9786=CARTESIAN_POINT('Ctrl Pts',(6.63306845520277,-15.3933171197393,0.));
#9787=CARTESIAN_POINT('Ctrl Pts',(6.66297054550544,-15.4424051151807,0.));
#9788=CARTESIAN_POINT('Ctrl Pts',(6.68074830397727,-15.4733031879166,0.));
#9789=CARTESIAN_POINT('Ctrl Pts',(6.69953551835471,-15.5083268912119,0.));
#9790=CARTESIAN_POINT('Ctrl Pts',(6.72790031412625,-15.5619248294191,0.));
#9791=CARTESIAN_POINT('Ctrl Pts',(6.77211692048664,-15.6387111659832,0.));
#9792=CARTESIAN_POINT('Ctrl Pts',(6.83570676658069,-15.7406883947778,0.));
#9793=CARTESIAN_POINT('Ctrl Pts',(6.91534043556371,-15.8583036897433,0.));
#9794=CARTESIAN_POINT('Ctrl Pts',(7.01217619187964,-15.9905219781863,0.));
#9795=CARTESIAN_POINT('Ctrl Pts',(7.12742326811382,-16.1361838672874,0.));
#9796=CARTESIAN_POINT('Ctrl Pts',(7.2621916599568,-16.2940809887434,0.));
#9797=CARTESIAN_POINT('Ctrl Pts',(7.41753779118422,-16.4629349257385,0.));
#9798=CARTESIAN_POINT('Ctrl Pts',(7.59444470905135,-16.6414085620714,0.));
#9799=CARTESIAN_POINT('Ctrl Pts',(7.84571320523309,-16.8766905033058,0.));
#9800=CARTESIAN_POINT('Ctrl Pts',(8.04476736935673,-17.0448123137865,0.));
#9801=CARTESIAN_POINT('Ctrl Pts',(8.17732893607279,-17.1502563092004,0.));
#9802=CARTESIAN_POINT('',(4.01273932064523,-15.7467591314704,0.));
#9803=CARTESIAN_POINT('Origin',(0.,0.,0.));
#9804=CARTESIAN_POINT('',(3.46506965370692,-18.6813621637974,0.));
#9805=CARTESIAN_POINT('Ctrl Pts',(3.46506965370692,-18.6813621637974,0.));
#9806=CARTESIAN_POINT('Ctrl Pts',(3.51033578853419,-18.5181384456162,0.));
#9807=CARTESIAN_POINT('Ctrl Pts',(3.57255446932203,-18.2651239417329,0.));
#9808=CARTESIAN_POINT('Ctrl Pts',(3.63753969769579,-17.9270849363835,0.));
#9809=CARTESIAN_POINT('Ctrl Pts',(3.67575622931334,-17.6787134541915,0.));
#9810=CARTESIAN_POINT('Ctrl Pts',(3.7021840355295,-17.4507975846592,0.));
#9811=CARTESIAN_POINT('Ctrl Pts',(3.71840435546372,-17.2438412568379,0.));
#9812=CARTESIAN_POINT('Ctrl Pts',(3.72602328845457,-17.0582577813421,0.));
#9813=CARTESIAN_POINT('Ctrl Pts',(3.72664910094712,-16.8943723095674,0.));
#9814=CARTESIAN_POINT('Ctrl Pts',(3.72194155665404,-16.7524120409277,0.));
#9815=CARTESIAN_POINT('Ctrl Pts',(3.71344611165872,-16.632533556064,0.));
#9816=CARTESIAN_POINT('Ctrl Pts',(3.70408422142791,-16.5444222357228,0.));
#9817=CARTESIAN_POINT('Ctrl Pts',(3.69552774561757,-16.4843881842109,0.));
#9818=CARTESIAN_POINT('Ctrl Pts',(3.69014050504827,-16.4450105654963,0.));
#9819=CARTESIAN_POINT('Ctrl Pts',(3.68636158229547,-16.409563995311,0.));
#9820=CARTESIAN_POINT('Ctrl Pts',(3.68169968173261,-16.3522749650865,0.));
#9821=CARTESIAN_POINT('Ctrl Pts',(3.67963072201297,-16.2732984400115,0.));
#9822=CARTESIAN_POINT('Ctrl Pts',(3.68733631276642,-16.1718717115691,0.));
#9823=CARTESIAN_POINT('Ctrl Pts',(3.70904952755071,-16.0682204478862,0.));
#9824=CARTESIAN_POINT('Ctrl Pts',(3.75315043649999,-15.958574817721,0.));
#9825=CARTESIAN_POINT('Ctrl Pts',(3.84407131175639,-15.8322454089585,0.));
#9826=CARTESIAN_POINT('Ctrl Pts',(3.94611544431021,-15.7691023294921,0.));
#9827=CARTESIAN_POINT('Ctrl Pts',(4.01273932064523,-15.7467591314704,0.));
#9828=CARTESIAN_POINT('',(2.47738131311187,-18.8377966288376,0.));
#9829=CARTESIAN_POINT('Origin',(0.,0.,0.));
#9830=CARTESIAN_POINT('',(1.04967429885974,-16.2160625265911,0.));
#9831=CARTESIAN_POINT('Ctrl Pts',(1.04967429885974,-16.2160625265911,0.));
#9832=CARTESIAN_POINT('Ctrl Pts',(1.11994179848648,-16.2167242606459,0.));
#9833=CARTESIAN_POINT('Ctrl Pts',(1.23650382033375,-16.2452435266959,0.));
#9834=CARTESIAN_POINT('Ctrl Pts',(1.36201264541055,-16.3372938385016,0.));
#9835=CARTESIAN_POINT('Ctrl Pts',(1.4378374653213,-16.4279450992208,0.));
#9836=CARTESIAN_POINT('Ctrl Pts',(1.4905179616981,-16.5198135565978,0.));
#9837=CARTESIAN_POINT('Ctrl Pts',(1.52918899676862,-16.6138949491149,0.));
#9838=CARTESIAN_POINT('Ctrl Pts',(1.55162638755016,-16.6896454316359,0.));
#9839=CARTESIAN_POINT('Ctrl Pts',(1.56489594057218,-16.7455711436431,0.));
#9840=CARTESIAN_POINT('Ctrl Pts',(1.57225556404312,-16.7804505865492,0.));
#9841=CARTESIAN_POINT('Ctrl Pts',(1.57930034717562,-16.8195656763126,0.));
#9842=CARTESIAN_POINT('Ctrl Pts',(1.58971419725804,-16.8793055486399,0.));
#9843=CARTESIAN_POINT('Ctrl Pts',(1.60803840593144,-16.9659973771906,0.));
#9844=CARTESIAN_POINT('Ctrl Pts',(1.6370032466926,-17.0826338282622,0.));
#9845=CARTESIAN_POINT('Ctrl Pts',(1.67639424155263,-17.2191007779953,0.));
#9846=CARTESIAN_POINT('Ctrl Pts',(1.72763282051121,-17.3747717371572,0.));
#9847=CARTESIAN_POINT('Ctrl Pts',(1.79222730418269,-17.548917731071,0.));
#9848=CARTESIAN_POINT('Ctrl Pts',(1.87160676754277,-17.7407325407201,0.));
#9849=CARTESIAN_POINT('Ctrl Pts',(1.96717098182925,-17.949326772361,0.));
#9850=CARTESIAN_POINT('Ctrl Pts',(2.08026807216972,-18.1737325312257,0.));
#9851=CARTESIAN_POINT('Ctrl Pts',(2.2465324944921,-18.4751451900744,0.));
#9852=CARTESIAN_POINT('Ctrl Pts',(2.38389175781394,-18.6965496529788,0.));
#9853=CARTESIAN_POINT('Ctrl Pts',(2.47738131311187,-18.8377966288376,0.));
#9854=CARTESIAN_POINT('',(-1.04967429885986,-16.2160625265911,0.));
#9855=CARTESIAN_POINT('Origin',(0.,0.,0.));
#9856=CARTESIAN_POINT('',(-2.47738131311198,-18.8377966288376,0.));
#9857=CARTESIAN_POINT('Ctrl Pts',(-2.47738131311198,-18.8377966288376,0.));
#9858=CARTESIAN_POINT('Ctrl Pts',(-2.38389175781398,-18.6965496529788,0.));
#9859=CARTESIAN_POINT('Ctrl Pts',(-2.24653249449213,-18.4751451900744,0.));
#9860=CARTESIAN_POINT('Ctrl Pts',(-2.08026807216976,-18.1737325312257,0.));
#9861=CARTESIAN_POINT('Ctrl Pts',(-1.96717098182926,-17.949326772361,0.));
#9862=CARTESIAN_POINT('Ctrl Pts',(-1.87160676754278,-17.7407325407201,0.));
#9863=CARTESIAN_POINT('Ctrl Pts',(-1.79222730418273,-17.548917731071,0.));
#9864=CARTESIAN_POINT('Ctrl Pts',(-1.7276328205112,-17.3747717371572,0.));
#9865=CARTESIAN_POINT('Ctrl Pts',(-1.67639424155264,-17.2191007779952,0.));
#9866=CARTESIAN_POINT('Ctrl Pts',(-1.63700324669264,-17.0826338282621,0.));
#9867=CARTESIAN_POINT('Ctrl Pts',(-1.60803840593146,-16.9659973771906,0.));
#9868=CARTESIAN_POINT('Ctrl Pts',(-1.58971419725806,-16.8793055486399,0.));
#9869=CARTESIAN_POINT('Ctrl Pts',(-1.57930034717566,-16.8195656763126,0.));
#9870=CARTESIAN_POINT('Ctrl Pts',(-1.57225556404312,-16.7804505865492,0.));
#9871=CARTESIAN_POINT('Ctrl Pts',(-1.56489594057218,-16.7455711436431,0.));
#9872=CARTESIAN_POINT('Ctrl Pts',(-1.55162638755018,-16.6896454316358,0.));
#9873=CARTESIAN_POINT('Ctrl Pts',(-1.52918899676863,-16.6138949491149,0.));
#9874=CARTESIAN_POINT('Ctrl Pts',(-1.49051796169811,-16.5198135565977,0.));
#9875=CARTESIAN_POINT('Ctrl Pts',(-1.43783746532133,-16.4279450992207,0.));
#9876=CARTESIAN_POINT('Ctrl Pts',(-1.3620126454106,-16.3372938385016,0.));
#9877=CARTESIAN_POINT('Ctrl Pts',(-1.23650382033378,-16.2452435266959,0.));
#9878=CARTESIAN_POINT('Ctrl Pts',(-1.1199417984865,-16.2167242606458,0.));
#9879=CARTESIAN_POINT('Ctrl Pts',(-1.04967429885986,-16.2160625265911,0.));
#9880=CARTESIAN_POINT('',(-3.46506965370701,-18.6813621637973,0.));
#9881=CARTESIAN_POINT('Origin',(0.,0.,0.));
#9882=CARTESIAN_POINT('',(-4.01273932064531,-15.7467591314704,0.));
#9883=CARTESIAN_POINT('Ctrl Pts',(-4.01273932064531,-15.7467591314704,0.));
#9884=CARTESIAN_POINT('Ctrl Pts',(-3.94611544431022,-15.7691023294921,0.));
#9885=CARTESIAN_POINT('Ctrl Pts',(-3.8440713117564,-15.8322454089585,0.));
#9886=CARTESIAN_POINT('Ctrl Pts',(-3.75315043650002,-15.958574817721,0.));
#9887=CARTESIAN_POINT('Ctrl Pts',(-3.70904952755073,-16.0682204478862,0.));
#9888=CARTESIAN_POINT('Ctrl Pts',(-3.68733631276642,-16.1718717115691,0.));
#9889=CARTESIAN_POINT('Ctrl Pts',(-3.67963072201298,-16.2732984400115,0.));
#9890=CARTESIAN_POINT('Ctrl Pts',(-3.68169968173261,-16.3522749650865,0.));
#9891=CARTESIAN_POINT('Ctrl Pts',(-3.68636158229546,-16.409563995311,0.));
#9892=CARTESIAN_POINT('Ctrl Pts',(-3.69014050504826,-16.4450105654963,0.));
#9893=CARTESIAN_POINT('Ctrl Pts',(-3.6955277456176,-16.4843881842109,0.));
#9894=CARTESIAN_POINT('Ctrl Pts',(-3.70408422142792,-16.5444222357228,0.));
#9895=CARTESIAN_POINT('Ctrl Pts',(-3.71344611165872,-16.632533556064,0.));
#9896=CARTESIAN_POINT('Ctrl Pts',(-3.72194155665407,-16.7524120409277,0.));
#9897=CARTESIAN_POINT('Ctrl Pts',(-3.72664910094713,-16.8943723095674,0.));
#9898=CARTESIAN_POINT('Ctrl Pts',(-3.72602328845455,-17.0582577813421,0.));
#9899=CARTESIAN_POINT('Ctrl Pts',(-3.71840435546375,-17.2438412568379,0.));
#9900=CARTESIAN_POINT('Ctrl Pts',(-3.70218403552949,-17.4507975846592,0.));
#9901=CARTESIAN_POINT('Ctrl Pts',(-3.67575622931335,-17.6787134541915,0.));
#9902=CARTESIAN_POINT('Ctrl Pts',(-3.63753969769582,-17.9270849363835,0.));
#9903=CARTESIAN_POINT('Ctrl Pts',(-3.57255446932205,-18.265123941733,0.));
#9904=CARTESIAN_POINT('Ctrl Pts',(-3.51033578853422,-18.5181384456163,0.));
#9905=CARTESIAN_POINT('Ctrl Pts',(-3.46506965370701,-18.6813621637973,0.));
#9906=CARTESIAN_POINT('',(-6.0093384844816,-15.0980247376578,0.));
#9907=CARTESIAN_POINT('Origin',(0.,0.,0.));
#9908=CARTESIAN_POINT('',(-8.17732893607292,-17.1502563092003,0.));
#9909=CARTESIAN_POINT('Ctrl Pts',(-8.17732893607292,-17.1502563092003,0.));
#9910=CARTESIAN_POINT('Ctrl Pts',(-8.04476736935674,-17.0448123137865,0.));
#9911=CARTESIAN_POINT('Ctrl Pts',(-7.8457132052331,-16.8766905033057,0.));
#9912=CARTESIAN_POINT('Ctrl Pts',(-7.59444470905137,-16.6414085620714,0.));
#9913=CARTESIAN_POINT('Ctrl Pts',(-7.41753779118422,-16.4629349257385,0.));
#9914=CARTESIAN_POINT('Ctrl Pts',(-7.2621916599568,-16.2940809887434,0.));
#9915=CARTESIAN_POINT('Ctrl Pts',(-7.12742326811384,-16.1361838672874,0.));
#9916=CARTESIAN_POINT('Ctrl Pts',(-7.01217619187963,-15.9905219781863,0.));
#9917=CARTESIAN_POINT('Ctrl Pts',(-6.9153404355637,-15.8583036897432,0.));
#9918=CARTESIAN_POINT('Ctrl Pts',(-6.8357067665807,-15.7406883947777,0.));
#9919=CARTESIAN_POINT('Ctrl Pts',(-6.77211692048664,-15.6387111659832,0.));
#9920=CARTESIAN_POINT('Ctrl Pts',(-6.72790031412625,-15.5619248294191,0.));
#9921=CARTESIAN_POINT('Ctrl Pts',(-6.69953551835473,-15.5083268912118,0.));
#9922=CARTESIAN_POINT('Ctrl Pts',(-6.68074830397727,-15.4733031879166,0.));
#9923=CARTESIAN_POINT('Ctrl Pts',(-6.66297054550543,-15.4424051151807,0.));
#9924=CARTESIAN_POINT('Ctrl Pts',(-6.63306845520277,-15.3933171197393,0.));
#9925=CARTESIAN_POINT('Ctrl Pts',(-6.58832104206024,-15.3282076647861,0.));
#9926=CARTESIAN_POINT('Ctrl Pts',(-6.52246995302227,-15.2506809503975,0.));
#9927=CARTESIAN_POINT('Ctrl Pts',(-6.44397890908497,-15.1795880240196,0.));
#9928=CARTESIAN_POINT('Ctrl Pts',(-6.34385243988824,-15.1168047097501,0.));
#9929=CARTESIAN_POINT('Ctrl Pts',(-6.19604134326091,-15.0680440207731,0.));
#9930=CARTESIAN_POINT('Ctrl Pts',(-6.07637133495395,-15.0769402326058,0.));
#9931=CARTESIAN_POINT('Ctrl Pts',(-6.0093384844816,-15.0980247376578,0.));
#9932=CARTESIAN_POINT('',(-9.06833546026116,-16.6962658094608,0.));
#9933=CARTESIAN_POINT('Origin',(0.,0.,0.));
#9934=CARTESIAN_POINT('',(-8.68235805704677,-13.7360532384392,0.));
#9935=CARTESIAN_POINT('Ctrl Pts',(-8.68235805704677,-13.7360532384392,0.));
#9936=CARTESIAN_POINT('Ctrl Pts',(-8.62589941321481,-13.7778907925313,0.));
#9937=CARTESIAN_POINT('Ctrl Pts',(-8.54836196063208,-13.8694768008521,0.));
#9938=CARTESIAN_POINT('Ctrl Pts',(-8.50092900394921,-14.0177193038531,0.));
#9939=CARTESIAN_POINT('Ctrl Pts',(-8.49286891019844,-14.1356264252377,0.));
#9940=CARTESIAN_POINT('Ctrl Pts',(-8.50424841775456,-14.2409143873564,0.));
#9941=CARTESIAN_POINT('Ctrl Pts',(-8.52826254822915,-14.3397580968626,0.));
#9942=CARTESIAN_POINT('Ctrl Pts',(-8.55463533425732,-14.4142298919555,0.));
#9943=CARTESIAN_POINT('Ctrl Pts',(-8.57677234909656,-14.4672743909627,0.));
#9944=CARTESIAN_POINT('Ctrl Pts',(-8.59131991078476,-14.4998183311667,0.));
#9945=CARTESIAN_POINT('Ctrl Pts',(-8.6086118344139,-14.5356039231527,0.));
#9946=CARTESIAN_POINT('Ctrl Pts',(-8.63530106864818,-14.5900556026053,0.));
#9947=CARTESIAN_POINT('Ctrl Pts',(-8.67143265073928,-14.6709614647944,0.));
#9948=CARTESIAN_POINT('Ctrl Pts',(-8.71655678814373,-14.7823474421093,0.));
#9949=CARTESIAN_POINT('Ctrl Pts',(-8.76490206435509,-14.9159049694657,0.));
#9950=CARTESIAN_POINT('Ctrl Pts',(-8.81495027721557,-15.0719627020186,0.));
#9951=CARTESIAN_POINT('Ctrl Pts',(-8.86505268915084,-15.2508174554788,0.));
#9952=CARTESIAN_POINT('Ctrl Pts',(-8.91357927057117,-15.4526569741556,0.));
#9953=CARTESIAN_POINT('Ctrl Pts',(-8.95887481023116,-15.6775844882862,0.));
#9954=CARTESIAN_POINT('Ctrl Pts',(-8.99927973772154,-15.9256093626227,0.));
#9955=CARTESIAN_POINT('Ctrl Pts',(-9.04193491022832,-16.2671851013731,0.));
#9956=CARTESIAN_POINT('Ctrl Pts',(-9.06094720995306,-16.5270428237395,0.));
#9957=CARTESIAN_POINT('Ctrl Pts',(-9.06833546026116,-16.6962658094608,0.));
#9958=CARTESIAN_POINT('',(-10.3807667497191,-12.5020870932787,0.));
#9959=CARTESIAN_POINT('Origin',(0.,0.,0.));
#9960=CARTESIAN_POINT('',(-13.0768226279701,-13.7839294091565,0.));
#9961=CARTESIAN_POINT('Ctrl Pts',(-13.0768226279701,-13.7839294091565,0.));
#9962=CARTESIAN_POINT('Ctrl Pts',(-12.9181650995967,-13.7246099871302,0.));
#9963=CARTESIAN_POINT('Ctrl Pts',(-12.6769008431476,-13.6262277632565,0.));
#9964=CARTESIAN_POINT('Ctrl Pts',(-12.3652241842034,-13.4801075753502,0.));
#9965=CARTESIAN_POINT('Ctrl Pts',(-12.1418243205134,-13.3650363045723,0.));
#9966=CARTESIAN_POINT('Ctrl Pts',(-11.9419026340297,-13.2524512620508,0.));
#9967=CARTESIAN_POINT('Ctrl Pts',(-11.764937382884,-13.1439278991698,0.));
#9968=CARTESIAN_POINT('Ctrl Pts',(-11.6103189008825,-13.0410085154728,0.));
#9969=CARTESIAN_POINT('Ctrl Pts',(-11.4773649257318,-12.9451853450404,0.));
#9970=CARTESIAN_POINT('Ctrl Pts',(-11.3652836809863,-12.8579347093876,0.));
#9971=CARTESIAN_POINT('Ctrl Pts',(-11.2732934467515,-12.7805989445416,0.));
#9972=CARTESIAN_POINT('Ctrl Pts',(-11.2075126722099,-12.7212344815888,0.));
#9973=CARTESIAN_POINT('Ctrl Pts',(-11.1639734745886,-12.6790250171322,0.));
#9974=CARTESIAN_POINT('Ctrl Pts',(-11.1352828524077,-12.651521064408,0.));
#9975=CARTESIAN_POINT('Ctrl Pts',(-11.1088271697991,-12.6276288804813,0.));
#9976=CARTESIAN_POINT('Ctrl Pts',(-11.0652195671547,-12.5901836766158,0.));
#9977=CARTESIAN_POINT('Ctrl Pts',(-11.0025423202231,-12.5420886163255,0.));
#9978=CARTESIAN_POINT('Ctrl Pts',(-10.9159571406243,-12.48870543503,0.));
#9979=CARTESIAN_POINT('Ctrl Pts',(-10.8193387993863,-12.4453471106187,0.));
#9980=CARTESIAN_POINT('Ctrl Pts',(-10.7047117573307,-12.4165774110367,0.));
#9981=CARTESIAN_POINT('Ctrl Pts',(-10.5490671691512,-12.4158793808611,0.));
#9982=CARTESIAN_POINT('Ctrl Pts',(-10.4380033085876,-12.4613202473787,0.));
#9983=CARTESIAN_POINT('Ctrl Pts',(-10.3807667497191,-12.5020870932787,0.));
#9984=CARTESIAN_POINT('',(-13.7839294091566,-13.07682262797,0.));
#9985=CARTESIAN_POINT('Origin',(0.,0.,0.));
#9986=CARTESIAN_POINT('',(-12.5020870932788,-10.380766749719,0.));
#9987=CARTESIAN_POINT('Ctrl Pts',(-12.5020870932788,-10.380766749719,0.));
#9988=CARTESIAN_POINT('Ctrl Pts',(-12.4613202473788,-10.4380033085876,0.));
#9989=CARTESIAN_POINT('Ctrl Pts',(-12.4158793808611,-10.5490671691512,0.));
#9990=CARTESIAN_POINT('Ctrl Pts',(-12.4165774110367,-10.7047117573306,0.));
#9991=CARTESIAN_POINT('Ctrl Pts',(-12.4453471106188,-10.8193387993863,0.));
#9992=CARTESIAN_POINT('Ctrl Pts',(-12.4887054350301,-10.9159571406243,0.));
#9993=CARTESIAN_POINT('Ctrl Pts',(-12.5420886163255,-11.0025423202231,0.));
#9994=CARTESIAN_POINT('Ctrl Pts',(-12.5901836766158,-11.0652195671547,0.));
#9995=CARTESIAN_POINT('Ctrl Pts',(-12.6276288804813,-11.1088271697991,0.));
#9996=CARTESIAN_POINT('Ctrl Pts',(-12.6515210644081,-11.1352828524077,0.));
#9997=CARTESIAN_POINT('Ctrl Pts',(-12.6790250171322,-11.1639734745885,0.));
#9998=CARTESIAN_POINT('Ctrl Pts',(-12.7212344815888,-11.2075126722099,0.));
#9999=CARTESIAN_POINT('Ctrl Pts',(-12.7805989445416,-11.2732934467515,0.));
#10000=CARTESIAN_POINT('Ctrl Pts',(-12.8579347093876,-11.3652836809863,
0.));
#10001=CARTESIAN_POINT('Ctrl Pts',(-12.9451853450404,-11.4773649257318,
0.));
#10002=CARTESIAN_POINT('Ctrl Pts',(-13.0410085154727,-11.6103189008825,
0.));
#10003=CARTESIAN_POINT('Ctrl Pts',(-13.1439278991698,-11.764937382884,0.));
#10004=CARTESIAN_POINT('Ctrl Pts',(-13.2524512620508,-11.9419026340297,
0.));
#10005=CARTESIAN_POINT('Ctrl Pts',(-13.3650363045724,-12.1418243205134,
0.));
#10006=CARTESIAN_POINT('Ctrl Pts',(-13.4801075753502,-12.3652241842034,
0.));
#10007=CARTESIAN_POINT('Ctrl Pts',(-13.6262277632565,-12.6769008431476,
0.));
#10008=CARTESIAN_POINT('Ctrl Pts',(-13.7246099871303,-12.9181650995967,
0.));
#10009=CARTESIAN_POINT('Ctrl Pts',(-13.7839294091566,-13.07682262797,0.));
#10010=CARTESIAN_POINT('',(-13.7360532384392,-8.68235805704666,0.));
#10011=CARTESIAN_POINT('Origin',(0.,0.,0.));
#10012=CARTESIAN_POINT('',(-16.6962658094609,-9.06833546026103,0.));
#10013=CARTESIAN_POINT('Ctrl Pts',(-16.6962658094609,-9.06833546026103,
0.));
#10014=CARTESIAN_POINT('Ctrl Pts',(-16.5270428237395,-9.06094720995301,
0.));
#10015=CARTESIAN_POINT('Ctrl Pts',(-16.2671851013731,-9.0419349102283,0.));
#10016=CARTESIAN_POINT('Ctrl Pts',(-15.9256093626227,-8.99927973772149,
0.));
#10017=CARTESIAN_POINT('Ctrl Pts',(-15.6775844882862,-8.95887481023114,
0.));
#10018=CARTESIAN_POINT('Ctrl Pts',(-15.4526569741556,-8.91357927057118,
0.));
#10019=CARTESIAN_POINT('Ctrl Pts',(-15.2508174554788,-8.8650526891508,0.));
#10020=CARTESIAN_POINT('Ctrl Pts',(-15.0719627020186,-8.81495027721558,
0.));
#10021=CARTESIAN_POINT('Ctrl Pts',(-14.9159049694657,-8.76490206435507,
0.));
#10022=CARTESIAN_POINT('Ctrl Pts',(-14.7823474421093,-8.71655678814369,
0.));
#10023=CARTESIAN_POINT('Ctrl Pts',(-14.6709614647944,-8.67143265073926,
0.));
#10024=CARTESIAN_POINT('Ctrl Pts',(-14.5900556026053,-8.63530106864816,
0.));
#10025=CARTESIAN_POINT('Ctrl Pts',(-14.5356039231527,-8.60861183441385,
0.));
#10026=CARTESIAN_POINT('Ctrl Pts',(-14.4998183311667,-8.59131991078476,
0.));
#10027=CARTESIAN_POINT('Ctrl Pts',(-14.4672743909627,-8.57677234909656,
0.));
#10028=CARTESIAN_POINT('Ctrl Pts',(-14.4142298919554,-8.5546353342573,0.));
#10029=CARTESIAN_POINT('Ctrl Pts',(-14.3397580968625,-8.52826254822913,
0.));
#10030=CARTESIAN_POINT('Ctrl Pts',(-14.2409143873564,-8.50424841775454,
0.));
#10031=CARTESIAN_POINT('Ctrl Pts',(-14.1356264252376,-8.4928689101984,0.));
#10032=CARTESIAN_POINT('Ctrl Pts',(-14.0177193038531,-8.50092900394916,
0.));
#10033=CARTESIAN_POINT('Ctrl Pts',(-13.8694768008521,-8.54836196063206,
0.));
#10034=CARTESIAN_POINT('Ctrl Pts',(-13.7778907925313,-8.62589941321478,
0.));
#10035=CARTESIAN_POINT('Ctrl Pts',(-13.7360532384392,-8.68235805704666,
0.));
#10036=CARTESIAN_POINT('',(-17.1502563092004,-8.1773289360728,0.));
#10037=CARTESIAN_POINT('Origin',(0.,0.,0.));
#10038=CARTESIAN_POINT('',(-15.0980247376579,-6.00933848448149,0.));
#10039=CARTESIAN_POINT('Ctrl Pts',(-15.0980247376579,-6.00933848448149,
0.));
#10040=CARTESIAN_POINT('Ctrl Pts',(-15.0769402326058,-6.07637133495397,
0.));
#10041=CARTESIAN_POINT('Ctrl Pts',(-15.0680440207731,-6.19604134326091,
0.));
#10042=CARTESIAN_POINT('Ctrl Pts',(-15.1168047097502,-6.34385243988823,
0.));
#10043=CARTESIAN_POINT('Ctrl Pts',(-15.1795880240196,-6.44397890908498,
0.));
#10044=CARTESIAN_POINT('Ctrl Pts',(-15.2506809503975,-6.52246995302231,
0.));
#10045=CARTESIAN_POINT('Ctrl Pts',(-15.3282076647862,-6.58832104206025,
0.));
#10046=CARTESIAN_POINT('Ctrl Pts',(-15.3933171197393,-6.63306845520279,
0.));
#10047=CARTESIAN_POINT('Ctrl Pts',(-15.4424051151807,-6.66297054550545,
0.));
#10048=CARTESIAN_POINT('Ctrl Pts',(-15.4733031879166,-6.68074830397729,
0.));
#10049=CARTESIAN_POINT('Ctrl Pts',(-15.5083268912119,-6.69953551835472,
0.));
#10050=CARTESIAN_POINT('Ctrl Pts',(-15.5619248294191,-6.72790031412626,
0.));
#10051=CARTESIAN_POINT('Ctrl Pts',(-15.6387111659832,-6.77211692048665,
0.));
#10052=CARTESIAN_POINT('Ctrl Pts',(-15.7406883947778,-6.8357067665807,0.));
#10053=CARTESIAN_POINT('Ctrl Pts',(-15.8583036897433,-6.91534043556372,
0.));
#10054=CARTESIAN_POINT('Ctrl Pts',(-15.9905219781863,-7.01217619187965,
0.));
#10055=CARTESIAN_POINT('Ctrl Pts',(-16.1361838672874,-7.12742326811382,
0.));
#10056=CARTESIAN_POINT('Ctrl Pts',(-16.2940809887434,-7.26219165995681,
0.));
#10057=CARTESIAN_POINT('Ctrl Pts',(-16.4629349257385,-7.41753779118423,
0.));
#10058=CARTESIAN_POINT('Ctrl Pts',(-16.6414085620714,-7.59444470905136,
0.));
#10059=CARTESIAN_POINT('Ctrl Pts',(-16.8766905033058,-7.84571320523309,
0.));
#10060=CARTESIAN_POINT('Ctrl Pts',(-17.0448123137865,-8.04476736935674,
0.));
#10061=CARTESIAN_POINT('Ctrl Pts',(-17.1502563092004,-8.1773289360728,0.));
#10062=CARTESIAN_POINT('',(-15.7467591314705,-4.0127393206452,0.));
#10063=CARTESIAN_POINT('Origin',(0.,0.,0.));
#10064=CARTESIAN_POINT('',(-18.6813621637974,-3.46506965370684,0.));
#10065=CARTESIAN_POINT('Ctrl Pts',(-18.6813621637974,-3.46506965370684,
0.));
#10066=CARTESIAN_POINT('Ctrl Pts',(-18.5181384456162,-3.51033578853419,
0.));
#10067=CARTESIAN_POINT('Ctrl Pts',(-18.265123941733,-3.57255446932203,0.));
#10068=CARTESIAN_POINT('Ctrl Pts',(-17.9270849363835,-3.63753969769578,
0.));
#10069=CARTESIAN_POINT('Ctrl Pts',(-17.6787134541915,-3.67575622931333,
0.));
#10070=CARTESIAN_POINT('Ctrl Pts',(-17.4507975846592,-3.70218403552949,
0.));
#10071=CARTESIAN_POINT('Ctrl Pts',(-17.2438412568379,-3.71840435546371,
0.));
#10072=CARTESIAN_POINT('Ctrl Pts',(-17.0582577813421,-3.72602328845455,
0.));
#10073=CARTESIAN_POINT('Ctrl Pts',(-16.8943723095674,-3.7266491009471,0.));
#10074=CARTESIAN_POINT('Ctrl Pts',(-16.7524120409277,-3.72194155665402,
0.));
#10075=CARTESIAN_POINT('Ctrl Pts',(-16.632533556064,-3.7134461116587,0.));
#10076=CARTESIAN_POINT('Ctrl Pts',(-16.5444222357228,-3.70408422142789,
0.));
#10077=CARTESIAN_POINT('Ctrl Pts',(-16.4843881842109,-3.69552774561754,
0.));
#10078=CARTESIAN_POINT('Ctrl Pts',(-16.4450105654964,-3.69014050504824,
0.));
#10079=CARTESIAN_POINT('Ctrl Pts',(-16.409563995311,-3.68636158229544,0.));
#10080=CARTESIAN_POINT('Ctrl Pts',(-16.3522749650865,-3.68169968173258,
0.));
#10081=CARTESIAN_POINT('Ctrl Pts',(-16.2732984400115,-3.67963072201294,
0.));
#10082=CARTESIAN_POINT('Ctrl Pts',(-16.1718717115691,-3.68733631276639,
0.));
#10083=CARTESIAN_POINT('Ctrl Pts',(-16.0682204478862,-3.70904952755068,
0.));
#10084=CARTESIAN_POINT('Ctrl Pts',(-15.958574817721,-3.75315043649995,0.));
#10085=CARTESIAN_POINT('Ctrl Pts',(-15.8322454089585,-3.84407131175635,
0.));
#10086=CARTESIAN_POINT('Ctrl Pts',(-15.7691023294921,-3.94611544431017,
0.));
#10087=CARTESIAN_POINT('Ctrl Pts',(-15.7467591314705,-4.0127393206452,0.));
#10088=CARTESIAN_POINT('',(-18.8377966288376,-2.47738131311187,0.));
#10089=CARTESIAN_POINT('Origin',(0.,0.,0.));
#10090=CARTESIAN_POINT('Ctrl Pts',(-16.2160625265912,-1.04967429885971,
0.));
#10091=CARTESIAN_POINT('Ctrl Pts',(-16.2167242606459,-1.11994179848649,
0.));
#10092=CARTESIAN_POINT('Ctrl Pts',(-16.2452435266959,-1.23650382033376,
0.));
#10093=CARTESIAN_POINT('Ctrl Pts',(-16.3372938385016,-1.36201264541056,
0.));
#10094=CARTESIAN_POINT('Ctrl Pts',(-16.4279450992208,-1.43783746532131,
0.));
#10095=CARTESIAN_POINT('Ctrl Pts',(-16.5198135565978,-1.49051796169811,
0.));
#10096=CARTESIAN_POINT('Ctrl Pts',(-16.6138949491149,-1.52918899676863,
0.));
#10097=CARTESIAN_POINT('Ctrl Pts',(-16.6896454316359,-1.55162638755017,
0.));
#10098=CARTESIAN_POINT('Ctrl Pts',(-16.7455711436431,-1.56489594057219,
0.));
#10099=CARTESIAN_POINT('Ctrl Pts',(-16.7804505865492,-1.57225556404312,
0.));
#10100=CARTESIAN_POINT('Ctrl Pts',(-16.8195656763126,-1.57930034717562,
0.));
#10101=CARTESIAN_POINT('Ctrl Pts',(-16.8793055486399,-1.58971419725805,
0.));
#10102=CARTESIAN_POINT('Ctrl Pts',(-16.9659973771906,-1.60803840593145,
0.));
#10103=CARTESIAN_POINT('Ctrl Pts',(-17.0826338282621,-1.63700324669261,
0.));
#10104=CARTESIAN_POINT('Ctrl Pts',(-17.2191007779953,-1.67639424155264,
0.));
#10105=CARTESIAN_POINT('Ctrl Pts',(-17.3747717371572,-1.72763282051121,
0.));
#10106=CARTESIAN_POINT('Ctrl Pts',(-17.548917731071,-1.79222730418269,0.));
#10107=CARTESIAN_POINT('Ctrl Pts',(-17.7407325407201,-1.87160676754278,
0.));
#10108=CARTESIAN_POINT('Ctrl Pts',(-17.949326772361,-1.96717098182925,0.));
#10109=CARTESIAN_POINT('Ctrl Pts',(-18.1737325312258,-2.08026807216972,
0.));
#10110=CARTESIAN_POINT('Ctrl Pts',(-18.4751451900744,-2.2465324944921,0.));
#10111=CARTESIAN_POINT('Ctrl Pts',(-18.6965496529788,-2.38389175781394,
0.));
#10112=CARTESIAN_POINT('Ctrl Pts',(-18.8377966288376,-2.47738131311187,
0.));
#10113=CARTESIAN_POINT('',(-18.8377966288375,2.47738131311205,0.));
#10114=CARTESIAN_POINT('Ctrl Pts',(-18.8377966288375,2.47738131311205,0.));
#10115=CARTESIAN_POINT('Ctrl Pts',(-18.6965496529788,2.38389175781397,0.));
#10116=CARTESIAN_POINT('Ctrl Pts',(-18.4751451900744,2.24653249449212,0.));
#10117=CARTESIAN_POINT('Ctrl Pts',(-18.1737325312257,2.08026807216975,0.));
#10118=CARTESIAN_POINT('Ctrl Pts',(-17.949326772361,1.96717098182926,0.));
#10119=CARTESIAN_POINT('Ctrl Pts',(-17.7407325407201,1.87160676754277,0.));
#10120=CARTESIAN_POINT('Ctrl Pts',(-17.548917731071,1.79222730418272,0.));
#10121=CARTESIAN_POINT('Ctrl Pts',(-17.3747717371572,1.72763282051119,0.));
#10122=CARTESIAN_POINT('Ctrl Pts',(-17.2191007779952,1.67639424155264,0.));
#10123=CARTESIAN_POINT('Ctrl Pts',(-17.0826338282621,1.63700324669263,0.));
#10124=CARTESIAN_POINT('Ctrl Pts',(-16.9659973771906,1.60803840593145,0.));
#10125=CARTESIAN_POINT('Ctrl Pts',(-16.8793055486399,1.58971419725805,0.));
#10126=CARTESIAN_POINT('Ctrl Pts',(-16.8195656763126,1.57930034717566,0.));
#10127=CARTESIAN_POINT('Ctrl Pts',(-16.7804505865492,1.57225556404312,0.));
#10128=CARTESIAN_POINT('Ctrl Pts',(-16.7455711436431,1.56489594057218,0.));
#10129=CARTESIAN_POINT('Ctrl Pts',(-16.6896454316358,1.55162638755017,0.));
#10130=CARTESIAN_POINT('Ctrl Pts',(-16.6138949491149,1.52918899676863,0.));
#10131=CARTESIAN_POINT('Ctrl Pts',(-16.5198135565977,1.4905179616981,0.));
#10132=CARTESIAN_POINT('Ctrl Pts',(-16.4279450992207,1.43783746532133,0.));
#10133=CARTESIAN_POINT('Ctrl Pts',(-16.3372938385016,1.3620126454106,0.));
#10134=CARTESIAN_POINT('Ctrl Pts',(-16.2452435266959,1.23650382033378,0.));
#10135=CARTESIAN_POINT('Ctrl Pts',(-16.2167242606458,1.1199417984865,0.));
#10136=CARTESIAN_POINT('Ctrl Pts',(-16.2160625265911,1.04967429885986,0.));
#10137=CARTESIAN_POINT('',(-18.6813621637973,3.46506965370702,0.));
#10138=CARTESIAN_POINT('Origin',(0.,0.,0.));
#10139=CARTESIAN_POINT('',(-15.7467591314704,4.01273932064536,0.));
#10140=CARTESIAN_POINT('Ctrl Pts',(-15.7467591314704,4.01273932064536,0.));
#10141=CARTESIAN_POINT('Ctrl Pts',(-15.7691023294921,3.94611544431018,0.));
#10142=CARTESIAN_POINT('Ctrl Pts',(-15.8322454089585,3.84407131175636,0.));
#10143=CARTESIAN_POINT('Ctrl Pts',(-15.958574817721,3.75315043649999,0.));
#10144=CARTESIAN_POINT('Ctrl Pts',(-16.0682204478862,3.7090495275507,0.));
#10145=CARTESIAN_POINT('Ctrl Pts',(-16.1718717115691,3.68733631276638,0.));
#10146=CARTESIAN_POINT('Ctrl Pts',(-16.2732984400115,3.67963072201295,0.));
#10147=CARTESIAN_POINT('Ctrl Pts',(-16.3522749650865,3.68169968173258,0.));
#10148=CARTESIAN_POINT('Ctrl Pts',(-16.409563995311,3.68636158229543,0.));
#10149=CARTESIAN_POINT('Ctrl Pts',(-16.4450105654964,3.69014050504823,0.));
#10150=CARTESIAN_POINT('Ctrl Pts',(-16.4843881842109,3.69552774561757,0.));
#10151=CARTESIAN_POINT('Ctrl Pts',(-16.5444222357228,3.70408422142789,0.));
#10152=CARTESIAN_POINT('Ctrl Pts',(-16.632533556064,3.7134461116587,0.));
#10153=CARTESIAN_POINT('Ctrl Pts',(-16.7524120409277,3.72194155665404,0.));
#10154=CARTESIAN_POINT('Ctrl Pts',(-16.8943723095674,3.72664910094711,0.));
#10155=CARTESIAN_POINT('Ctrl Pts',(-17.0582577813421,3.72602328845453,0.));
#10156=CARTESIAN_POINT('Ctrl Pts',(-17.2438412568379,3.71840435546374,0.));
#10157=CARTESIAN_POINT('Ctrl Pts',(-17.4507975846592,3.70218403552947,0.));
#10158=CARTESIAN_POINT('Ctrl Pts',(-17.6787134541915,3.67575622931334,0.));
#10159=CARTESIAN_POINT('Ctrl Pts',(-17.9270849363835,3.63753969769581,0.));
#10160=CARTESIAN_POINT('Ctrl Pts',(-18.265123941733,3.57255446932205,0.));
#10161=CARTESIAN_POINT('Ctrl Pts',(-18.5181384456163,3.51033578853423,0.));
#10162=CARTESIAN_POINT('Ctrl Pts',(-18.6813621637973,3.46506965370702,0.));
#10163=CARTESIAN_POINT('',(-15.0980247376578,6.00933848448163,0.));
#10164=CARTESIAN_POINT('Origin',(0.,0.,0.));
#10165=CARTESIAN_POINT('',(-17.1502563092003,8.17732893607296,0.));
#10166=CARTESIAN_POINT('Ctrl Pts',(-17.1502563092003,8.17732893607296,0.));
#10167=CARTESIAN_POINT('Ctrl Pts',(-17.0448123137865,8.04476736935675,0.));
#10168=CARTESIAN_POINT('Ctrl Pts',(-16.8766905033057,7.8457132052331,0.));
#10169=CARTESIAN_POINT('Ctrl Pts',(-16.6414085620714,7.59444470905138,0.));
#10170=CARTESIAN_POINT('Ctrl Pts',(-16.4629349257385,7.41753779118423,0.));
#10171=CARTESIAN_POINT('Ctrl Pts',(-16.2940809887434,7.26219165995682,0.));
#10172=CARTESIAN_POINT('Ctrl Pts',(-16.1361838672874,7.12742326811386,0.));
#10173=CARTESIAN_POINT('Ctrl Pts',(-15.9905219781863,7.01217619187965,0.));
#10174=CARTESIAN_POINT('Ctrl Pts',(-15.8583036897432,6.91534043556372,0.));
#10175=CARTESIAN_POINT('Ctrl Pts',(-15.7406883947777,6.83570676658073,0.));
#10176=CARTESIAN_POINT('Ctrl Pts',(-15.6387111659832,6.77211692048666,0.));
#10177=CARTESIAN_POINT('Ctrl Pts',(-15.5619248294191,6.72790031412627,0.));
#10178=CARTESIAN_POINT('Ctrl Pts',(-15.5083268912118,6.69953551835476,0.));
#10179=CARTESIAN_POINT('Ctrl Pts',(-15.4733031879166,6.68074830397729,0.));
#10180=CARTESIAN_POINT('Ctrl Pts',(-15.4424051151807,6.66297054550545,0.));
#10181=CARTESIAN_POINT('Ctrl Pts',(-15.3933171197393,6.6330684552028,0.));
#10182=CARTESIAN_POINT('Ctrl Pts',(-15.3282076647861,6.58832104206026,0.));
#10183=CARTESIAN_POINT('Ctrl Pts',(-15.2506809503975,6.5224699530223,0.));
#10184=CARTESIAN_POINT('Ctrl Pts',(-15.1795880240196,6.443978909085,0.));
#10185=CARTESIAN_POINT('Ctrl Pts',(-15.1168047097501,6.34385243988827,0.));
#10186=CARTESIAN_POINT('Ctrl Pts',(-15.0680440207731,6.19604134326095,0.));
#10187=CARTESIAN_POINT('Ctrl Pts',(-15.0769402326058,6.07637133495398,0.));
#10188=CARTESIAN_POINT('Ctrl Pts',(-15.0980247376578,6.00933848448163,0.));
#10189=CARTESIAN_POINT('',(-16.6962658094608,9.06833546026117,0.));
#10190=CARTESIAN_POINT('Origin',(-1.73472347597681E-15,0.,0.));
#10191=CARTESIAN_POINT('',(-13.7360532384391,8.68235805704682,0.));
#10192=CARTESIAN_POINT('Ctrl Pts',(-13.7360532384391,8.68235805704682,0.));
#10193=CARTESIAN_POINT('Ctrl Pts',(-13.7778907925313,8.62589941321479,0.));
#10194=CARTESIAN_POINT('Ctrl Pts',(-13.8694768008521,8.54836196063206,0.));
#10195=CARTESIAN_POINT('Ctrl Pts',(-14.0177193038531,8.50092900394919,0.));
#10196=CARTESIAN_POINT('Ctrl Pts',(-14.1356264252377,8.49286891019842,0.));
#10197=CARTESIAN_POINT('Ctrl Pts',(-14.2409143873564,8.50424841775455,0.));
#10198=CARTESIAN_POINT('Ctrl Pts',(-14.3397580968626,8.52826254822914,0.));
#10199=CARTESIAN_POINT('Ctrl Pts',(-14.4142298919555,8.55463533425731,0.));
#10200=CARTESIAN_POINT('Ctrl Pts',(-14.4672743909627,8.57677234909655,0.));
#10201=CARTESIAN_POINT('Ctrl Pts',(-14.4998183311667,8.59131991078475,0.));
#10202=CARTESIAN_POINT('Ctrl Pts',(-14.5356039231527,8.60861183441388,0.));
#10203=CARTESIAN_POINT('Ctrl Pts',(-14.5900556026053,8.63530106864817,0.));
#10204=CARTESIAN_POINT('Ctrl Pts',(-14.6709614647944,8.67143265073926,0.));
#10205=CARTESIAN_POINT('Ctrl Pts',(-14.7823474421093,8.71655678814371,0.));
#10206=CARTESIAN_POINT('Ctrl Pts',(-14.9159049694657,8.76490206435508,0.));
#10207=CARTESIAN_POINT('Ctrl Pts',(-15.0719627020186,8.81495027721556,0.));
#10208=CARTESIAN_POINT('Ctrl Pts',(-15.2508174554788,8.86505268915083,0.));
#10209=CARTESIAN_POINT('Ctrl Pts',(-15.4526569741556,8.91357927057117,0.));
#10210=CARTESIAN_POINT('Ctrl Pts',(-15.6775844882863,8.95887481023116,0.));
#10211=CARTESIAN_POINT('Ctrl Pts',(-15.9256093626227,8.99927973772153,0.));
#10212=CARTESIAN_POINT('Ctrl Pts',(-16.2671851013731,9.04193491022832,0.));
#10213=CARTESIAN_POINT('Ctrl Pts',(-16.5270428237395,9.06094720995306,0.));
#10214=CARTESIAN_POINT('Ctrl Pts',(-16.6962658094608,9.06833546026117,0.));
#10215=CARTESIAN_POINT('',(-12.5020870932787,10.3807667497191,0.));
#10216=CARTESIAN_POINT('Origin',(0.,0.,0.));
#10217=CARTESIAN_POINT('',(-13.7839294091564,13.0768226279702,0.));
#10218=CARTESIAN_POINT('Ctrl Pts',(-13.7839294091564,13.0768226279702,0.));
#10219=CARTESIAN_POINT('Ctrl Pts',(-13.7246099871302,12.9181650995968,0.));
#10220=CARTESIAN_POINT('Ctrl Pts',(-13.6262277632565,12.6769008431476,0.));
#10221=CARTESIAN_POINT('Ctrl Pts',(-13.4801075753502,12.3652241842034,0.));
#10222=CARTESIAN_POINT('Ctrl Pts',(-13.3650363045723,12.1418243205134,0.));
#10223=CARTESIAN_POINT('Ctrl Pts',(-13.2524512620508,11.9419026340297,0.));
#10224=CARTESIAN_POINT('Ctrl Pts',(-13.1439278991698,11.764937382884,0.));
#10225=CARTESIAN_POINT('Ctrl Pts',(-13.0410085154728,11.6103189008826,0.));
#10226=CARTESIAN_POINT('Ctrl Pts',(-12.9451853450404,11.4773649257318,0.));
#10227=CARTESIAN_POINT('Ctrl Pts',(-12.8579347093876,11.3652836809863,0.));
#10228=CARTESIAN_POINT('Ctrl Pts',(-12.7805989445416,11.2732934467516,0.));
#10229=CARTESIAN_POINT('Ctrl Pts',(-12.7212344815888,11.2075126722099,0.));
#10230=CARTESIAN_POINT('Ctrl Pts',(-12.6790250171322,11.1639734745886,0.));
#10231=CARTESIAN_POINT('Ctrl Pts',(-12.651521064408,11.1352828524077,0.));
#10232=CARTESIAN_POINT('Ctrl Pts',(-12.6276288804813,11.1088271697991,0.));
#10233=CARTESIAN_POINT('Ctrl Pts',(-12.5901836766158,11.0652195671547,0.));
#10234=CARTESIAN_POINT('Ctrl Pts',(-12.5420886163255,11.0025423202231,0.));
#10235=CARTESIAN_POINT('Ctrl Pts',(-12.48870543503,10.9159571406243,0.));
#10236=CARTESIAN_POINT('Ctrl Pts',(-12.4453471106187,10.8193387993863,0.));
#10237=CARTESIAN_POINT('Ctrl Pts',(-12.4165774110367,10.7047117573307,0.));
#10238=CARTESIAN_POINT('Ctrl Pts',(-12.4158793808611,10.5490671691512,0.));
#10239=CARTESIAN_POINT('Ctrl Pts',(-12.4613202473787,10.4380033085876,0.));
#10240=CARTESIAN_POINT('Ctrl Pts',(-12.5020870932787,10.3807667497191,0.));
#10241=CARTESIAN_POINT('',(-13.07682262797,13.7839294091566,0.));
#10242=CARTESIAN_POINT('Origin',(1.57723797680727E-16,0.,0.));
#10243=CARTESIAN_POINT('',(-10.380766749719,12.5020870932788,0.));
#10244=CARTESIAN_POINT('Ctrl Pts',(-10.380766749719,12.5020870932788,0.));
#10245=CARTESIAN_POINT('Ctrl Pts',(-10.4380033085876,12.4613202473787,0.));
#10246=CARTESIAN_POINT('Ctrl Pts',(-10.5490671691512,12.4158793808611,0.));
#10247=CARTESIAN_POINT('Ctrl Pts',(-10.7047117573307,12.4165774110367,0.));
#10248=CARTESIAN_POINT('Ctrl Pts',(-10.8193387993863,12.4453471106187,0.));
#10249=CARTESIAN_POINT('Ctrl Pts',(-10.9159571406243,12.48870543503,0.));
#10250=CARTESIAN_POINT('Ctrl Pts',(-11.0025423202232,12.5420886163255,0.));
#10251=CARTESIAN_POINT('Ctrl Pts',(-11.0652195671547,12.5901836766158,0.));
#10252=CARTESIAN_POINT('Ctrl Pts',(-11.1088271697991,12.6276288804813,0.));
#10253=CARTESIAN_POINT('Ctrl Pts',(-11.1352828524077,12.651521064408,0.));
#10254=CARTESIAN_POINT('Ctrl Pts',(-11.1639734745886,12.6790250171322,0.));
#10255=CARTESIAN_POINT('Ctrl Pts',(-11.20751267221,12.7212344815888,0.));
#10256=CARTESIAN_POINT('Ctrl Pts',(-11.2732934467516,12.7805989445416,0.));
#10257=CARTESIAN_POINT('Ctrl Pts',(-11.3652836809863,12.8579347093876,0.));
#10258=CARTESIAN_POINT('Ctrl Pts',(-11.4773649257319,12.9451853450404,0.));
#10259=CARTESIAN_POINT('Ctrl Pts',(-11.6103189008826,13.0410085154727,0.));
#10260=CARTESIAN_POINT('Ctrl Pts',(-11.764937382884,13.1439278991698,0.));
#10261=CARTESIAN_POINT('Ctrl Pts',(-11.9419026340297,13.2524512620507,0.));
#10262=CARTESIAN_POINT('Ctrl Pts',(-12.1418243205134,13.3650363045724,0.));
#10263=CARTESIAN_POINT('Ctrl Pts',(-12.3652241842034,13.4801075753502,0.));
#10264=CARTESIAN_POINT('Ctrl Pts',(-12.6769008431476,13.6262277632565,0.));
#10265=CARTESIAN_POINT('Ctrl Pts',(-12.9181650995968,13.7246099871303,0.));
#10266=CARTESIAN_POINT('Ctrl Pts',(-13.07682262797,13.7839294091566,0.));
#10267=CARTESIAN_POINT('',(-8.68235805704666,13.7360532384392,0.));
#10268=CARTESIAN_POINT('Origin',(0.,0.,0.));
#10269=CARTESIAN_POINT('',(-9.06833546026097,16.6962658094609,0.));
#10270=CARTESIAN_POINT('Ctrl Pts',(-9.06833546026097,16.6962658094609,0.));
#10271=CARTESIAN_POINT('Ctrl Pts',(-9.06094720995302,16.5270428237395,0.));
#10272=CARTESIAN_POINT('Ctrl Pts',(-9.04193491022831,16.2671851013731,0.));
#10273=CARTESIAN_POINT('Ctrl Pts',(-8.9992797377215,15.9256093626227,0.));
#10274=CARTESIAN_POINT('Ctrl Pts',(-8.95887481023115,15.6775844882862,0.));
#10275=CARTESIAN_POINT('Ctrl Pts',(-8.91357927057119,15.4526569741556,0.));
#10276=CARTESIAN_POINT('Ctrl Pts',(-8.8650526891508,15.2508174554788,0.));
#10277=CARTESIAN_POINT('Ctrl Pts',(-8.81495027721559,15.0719627020186,0.));
#10278=CARTESIAN_POINT('Ctrl Pts',(-8.76490206435507,14.9159049694657,0.));
#10279=CARTESIAN_POINT('Ctrl Pts',(-8.71655678814369,14.7823474421093,0.));
#10280=CARTESIAN_POINT('Ctrl Pts',(-8.67143265073926,14.6709614647944,0.));
#10281=CARTESIAN_POINT('Ctrl Pts',(-8.63530106864816,14.5900556026053,0.));
#10282=CARTESIAN_POINT('Ctrl Pts',(-8.60861183441386,14.5356039231527,0.));
#10283=CARTESIAN_POINT('Ctrl Pts',(-8.59131991078476,14.4998183311667,0.));
#10284=CARTESIAN_POINT('Ctrl Pts',(-8.57677234909655,14.4672743909627,0.));
#10285=CARTESIAN_POINT('Ctrl Pts',(-8.55463533425729,14.4142298919554,0.));
#10286=CARTESIAN_POINT('Ctrl Pts',(-8.52826254822913,14.3397580968626,0.));
#10287=CARTESIAN_POINT('Ctrl Pts',(-8.50424841775454,14.2409143873564,0.));
#10288=CARTESIAN_POINT('Ctrl Pts',(-8.49286891019839,14.1356264252377,0.));
#10289=CARTESIAN_POINT('Ctrl Pts',(-8.50092900394916,14.0177193038531,0.));
#10290=CARTESIAN_POINT('Ctrl Pts',(-8.54836196063204,13.8694768008521,0.));
#10291=CARTESIAN_POINT('Ctrl Pts',(-8.62589941321477,13.7778907925313,0.));
#10292=CARTESIAN_POINT('Ctrl Pts',(-8.68235805704666,13.7360532384392,0.));
#10293=CARTESIAN_POINT('',(-8.1773289360728,17.1502563092004,0.));
#10294=CARTESIAN_POINT('Origin',(1.73472347597681E-15,0.,0.));
#10295=CARTESIAN_POINT('',(-6.00933848448141,15.0980247376579,0.));
#10296=CARTESIAN_POINT('Ctrl Pts',(-6.00933848448141,15.0980247376579,0.));
#10297=CARTESIAN_POINT('Ctrl Pts',(-6.076371334954,15.0769402326058,0.));
#10298=CARTESIAN_POINT('Ctrl Pts',(-6.19604134326094,15.0680440207731,0.));
#10299=CARTESIAN_POINT('Ctrl Pts',(-6.34385243988825,15.1168047097501,0.));
#10300=CARTESIAN_POINT('Ctrl Pts',(-6.44397890908501,15.1795880240196,0.));
#10301=CARTESIAN_POINT('Ctrl Pts',(-6.52246995302233,15.2506809503975,0.));
#10302=CARTESIAN_POINT('Ctrl Pts',(-6.58832104206028,15.3282076647862,0.));
#10303=CARTESIAN_POINT('Ctrl Pts',(-6.63306845520281,15.3933171197393,0.));
#10304=CARTESIAN_POINT('Ctrl Pts',(-6.66297054550547,15.4424051151807,0.));
#10305=CARTESIAN_POINT('Ctrl Pts',(-6.68074830397731,15.4733031879166,0.));
#10306=CARTESIAN_POINT('Ctrl Pts',(-6.69953551835474,15.5083268912119,0.));
#10307=CARTESIAN_POINT('Ctrl Pts',(-6.72790031412628,15.5619248294191,0.));
#10308=CARTESIAN_POINT('Ctrl Pts',(-6.77211692048667,15.6387111659832,0.));
#10309=CARTESIAN_POINT('Ctrl Pts',(-6.83570676658072,15.7406883947778,0.));
#10310=CARTESIAN_POINT('Ctrl Pts',(-6.91534043556374,15.8583036897433,0.));
#10311=CARTESIAN_POINT('Ctrl Pts',(-7.01217619187967,15.9905219781863,0.));
#10312=CARTESIAN_POINT('Ctrl Pts',(-7.12742326811385,16.1361838672874,0.));
#10313=CARTESIAN_POINT('Ctrl Pts',(-7.26219165995682,16.2940809887434,0.));
#10314=CARTESIAN_POINT('Ctrl Pts',(-7.41753779118424,16.4629349257385,0.));
#10315=CARTESIAN_POINT('Ctrl Pts',(-7.59444470905137,16.6414085620714,0.));
#10316=CARTESIAN_POINT('Ctrl Pts',(-7.8457132052331,16.8766905033058,0.));
#10317=CARTESIAN_POINT('Ctrl Pts',(-8.04476736935674,17.0448123137865,0.));
#10318=CARTESIAN_POINT('Ctrl Pts',(-8.1773289360728,17.1502563092004,0.));
#10319=CARTESIAN_POINT('',(-4.01273932064518,15.7467591314705,0.));
#10320=CARTESIAN_POINT('Origin',(0.,0.,0.));
#10321=CARTESIAN_POINT('',(-3.46506965370679,18.6813621637974,0.));
#10322=CARTESIAN_POINT('Ctrl Pts',(-3.46506965370679,18.6813621637974,0.));
#10323=CARTESIAN_POINT('Ctrl Pts',(-3.51033578853418,18.5181384456162,0.));
#10324=CARTESIAN_POINT('Ctrl Pts',(-3.57255446932203,18.265123941733,0.));
#10325=CARTESIAN_POINT('Ctrl Pts',(-3.63753969769577,17.9270849363835,0.));
#10326=CARTESIAN_POINT('Ctrl Pts',(-3.67575622931332,17.6787134541915,0.));
#10327=CARTESIAN_POINT('Ctrl Pts',(-3.70218403552948,17.4507975846592,0.));
#10328=CARTESIAN_POINT('Ctrl Pts',(-3.7184043554637,17.2438412568379,0.));
#10329=CARTESIAN_POINT('Ctrl Pts',(-3.72602328845454,17.0582577813421,0.));
#10330=CARTESIAN_POINT('Ctrl Pts',(-3.72664910094709,16.8943723095674,0.));
#10331=CARTESIAN_POINT('Ctrl Pts',(-3.72194155665401,16.7524120409277,0.));
#10332=CARTESIAN_POINT('Ctrl Pts',(-3.71344611165868,16.632533556064,0.));
#10333=CARTESIAN_POINT('Ctrl Pts',(-3.70408422142788,16.5444222357228,0.));
#10334=CARTESIAN_POINT('Ctrl Pts',(-3.69552774561753,16.4843881842109,0.));
#10335=CARTESIAN_POINT('Ctrl Pts',(-3.69014050504823,16.4450105654964,0.));
#10336=CARTESIAN_POINT('Ctrl Pts',(-3.68636158229542,16.409563995311,0.));
#10337=CARTESIAN_POINT('Ctrl Pts',(-3.68169968173256,16.3522749650865,0.));
#10338=CARTESIAN_POINT('Ctrl Pts',(-3.67963072201293,16.2732984400115,0.));
#10339=CARTESIAN_POINT('Ctrl Pts',(-3.68733631276638,16.1718717115691,0.));
#10340=CARTESIAN_POINT('Ctrl Pts',(-3.70904952755066,16.0682204478862,0.));
#10341=CARTESIAN_POINT('Ctrl Pts',(-3.75315043649994,15.958574817721,0.));
#10342=CARTESIAN_POINT('Ctrl Pts',(-3.84407131175633,15.8322454089585,0.));
#10343=CARTESIAN_POINT('Ctrl Pts',(-3.94611544431016,15.7691023294921,0.));
#10344=CARTESIAN_POINT('Ctrl Pts',(-4.01273932064518,15.7467591314705,0.));
#10345=CARTESIAN_POINT('',(-2.47738131311187,18.8377966288376,0.));
#10346=CARTESIAN_POINT('Origin',(-1.73472347597681E-15,0.,0.));
#10347=CARTESIAN_POINT('',(-1.04967429885962,16.2160625265911,0.));
#10348=CARTESIAN_POINT('Ctrl Pts',(-1.04967429885962,16.2160625265911,0.));
#10349=CARTESIAN_POINT('Ctrl Pts',(-1.11994179848651,16.2167242606459,0.));
#10350=CARTESIAN_POINT('Ctrl Pts',(-1.23650382033378,16.2452435266959,0.));
#10351=CARTESIAN_POINT('Ctrl Pts',(-1.36201264541058,16.3372938385016,0.));
#10352=CARTESIAN_POINT('Ctrl Pts',(-1.43783746532133,16.4279450992208,0.));
#10353=CARTESIAN_POINT('Ctrl Pts',(-1.49051796169812,16.5198135565978,0.));
#10354=CARTESIAN_POINT('Ctrl Pts',(-1.52918899676864,16.6138949491149,0.));
#10355=CARTESIAN_POINT('Ctrl Pts',(-1.55162638755018,16.6896454316359,0.));
#10356=CARTESIAN_POINT('Ctrl Pts',(-1.5648959405722,16.7455711436431,0.));
#10357=CARTESIAN_POINT('Ctrl Pts',(-1.57225556404314,16.7804505865492,0.));
#10358=CARTESIAN_POINT('Ctrl Pts',(-1.57930034717564,16.8195656763126,0.));
#10359=CARTESIAN_POINT('Ctrl Pts',(-1.58971419725806,16.8793055486399,0.));
#10360=CARTESIAN_POINT('Ctrl Pts',(-1.60803840593146,16.9659973771906,0.));
#10361=CARTESIAN_POINT('Ctrl Pts',(-1.63700324669262,17.0826338282622,0.));
#10362=CARTESIAN_POINT('Ctrl Pts',(-1.67639424155265,17.2191007779953,0.));
#10363=CARTESIAN_POINT('Ctrl Pts',(-1.72763282051122,17.3747717371572,0.));
#10364=CARTESIAN_POINT('Ctrl Pts',(-1.7922273041827,17.548917731071,0.));
#10365=CARTESIAN_POINT('Ctrl Pts',(-1.87160676754278,17.7407325407201,0.));
#10366=CARTESIAN_POINT('Ctrl Pts',(-1.96717098182926,17.949326772361,0.));
#10367=CARTESIAN_POINT('Ctrl Pts',(-2.08026807216973,18.1737325312257,0.));
#10368=CARTESIAN_POINT('Ctrl Pts',(-2.24653249449211,18.4751451900744,0.));
#10369=CARTESIAN_POINT('Ctrl Pts',(-2.38389175781394,18.6965496529788,0.));
#10370=CARTESIAN_POINT('Ctrl Pts',(-2.47738131311187,18.8377966288376,0.));
#10371=CARTESIAN_POINT('',(1.04967429885989,16.2160625265911,0.));
#10372=CARTESIAN_POINT('Origin',(0.,0.,0.));
#10373=CARTESIAN_POINT('',(2.47738131311212,18.8377966288375,0.));
#10374=CARTESIAN_POINT('Ctrl Pts',(2.47738131311212,18.8377966288375,0.));
#10375=CARTESIAN_POINT('Ctrl Pts',(2.38389175781397,18.6965496529788,0.));
#10376=CARTESIAN_POINT('Ctrl Pts',(2.24653249449213,18.4751451900744,0.));
#10377=CARTESIAN_POINT('Ctrl Pts',(2.08026807216976,18.1737325312257,0.));
#10378=CARTESIAN_POINT('Ctrl Pts',(1.96717098182927,17.949326772361,0.));
#10379=CARTESIAN_POINT('Ctrl Pts',(1.87160676754279,17.7407325407201,0.));
#10380=CARTESIAN_POINT('Ctrl Pts',(1.79222730418274,17.548917731071,0.));
#10381=CARTESIAN_POINT('Ctrl Pts',(1.72763282051121,17.3747717371572,0.));
#10382=CARTESIAN_POINT('Ctrl Pts',(1.67639424155266,17.2191007779952,0.));
#10383=CARTESIAN_POINT('Ctrl Pts',(1.63700324669265,17.0826338282621,0.));
#10384=CARTESIAN_POINT('Ctrl Pts',(1.60803840593148,16.9659973771906,0.));
#10385=CARTESIAN_POINT('Ctrl Pts',(1.58971419725808,16.8793055486399,0.));
#10386=CARTESIAN_POINT('Ctrl Pts',(1.57930034717568,16.8195656763126,0.));
#10387=CARTESIAN_POINT('Ctrl Pts',(1.57225556404314,16.7804505865492,0.));
#10388=CARTESIAN_POINT('Ctrl Pts',(1.5648959405722,16.7455711436431,0.));
#10389=CARTESIAN_POINT('Ctrl Pts',(1.5516263875502,16.6896454316358,0.));
#10390=CARTESIAN_POINT('Ctrl Pts',(1.52918899676866,16.6138949491149,0.));
#10391=CARTESIAN_POINT('Ctrl Pts',(1.49051796169813,16.5198135565977,0.));
#10392=CARTESIAN_POINT('Ctrl Pts',(1.43783746532136,16.4279450992207,0.));
#10393=CARTESIAN_POINT('Ctrl Pts',(1.36201264541063,16.3372938385016,0.));
#10394=CARTESIAN_POINT('Ctrl Pts',(1.23650382033381,16.2452435266959,0.));
#10395=CARTESIAN_POINT('Ctrl Pts',(1.11994179848653,16.2167242606458,0.));
#10396=CARTESIAN_POINT('Ctrl Pts',(1.04967429885989,16.2160625265911,0.));
#10397=CARTESIAN_POINT('',(3.46506965370702,18.6813621637974,0.));
#10398=CARTESIAN_POINT('Origin',(0.,8.67361737988404E-16,0.));
#10399=CARTESIAN_POINT('',(4.01273932064543,15.7467591314704,0.));
#10400=CARTESIAN_POINT('Ctrl Pts',(4.01273932064543,15.7467591314704,0.));
#10401=CARTESIAN_POINT('Ctrl Pts',(3.94611544431017,15.7691023294921,0.));
#10402=CARTESIAN_POINT('Ctrl Pts',(3.84407131175635,15.8322454089585,0.));
#10403=CARTESIAN_POINT('Ctrl Pts',(3.75315043649997,15.9585748177211,0.));
#10404=CARTESIAN_POINT('Ctrl Pts',(3.70904952755068,16.0682204478862,0.));
#10405=CARTESIAN_POINT('Ctrl Pts',(3.68733631276637,16.1718717115691,0.));
#10406=CARTESIAN_POINT('Ctrl Pts',(3.67963072201293,16.2732984400116,0.));
#10407=CARTESIAN_POINT('Ctrl Pts',(3.68169968173257,16.3522749650866,0.));
#10408=CARTESIAN_POINT('Ctrl Pts',(3.68636158229542,16.409563995311,0.));
#10409=CARTESIAN_POINT('Ctrl Pts',(3.69014050504822,16.4450105654964,0.));
#10410=CARTESIAN_POINT('Ctrl Pts',(3.69552774561756,16.4843881842109,0.));
#10411=CARTESIAN_POINT('Ctrl Pts',(3.70408422142788,16.5444222357228,0.));
#10412=CARTESIAN_POINT('Ctrl Pts',(3.71344611165869,16.632533556064,0.));
#10413=CARTESIAN_POINT('Ctrl Pts',(3.72194155665403,16.7524120409277,0.));
#10414=CARTESIAN_POINT('Ctrl Pts',(3.7266491009471,16.8943723095674,0.));
#10415=CARTESIAN_POINT('Ctrl Pts',(3.72602328845452,17.0582577813421,0.));
#10416=CARTESIAN_POINT('Ctrl Pts',(3.71840435546373,17.2438412568379,0.));
#10417=CARTESIAN_POINT('Ctrl Pts',(3.70218403552947,17.4507975846592,0.));
#10418=CARTESIAN_POINT('Ctrl Pts',(3.67575622931333,17.6787134541915,0.));
#10419=CARTESIAN_POINT('Ctrl Pts',(3.63753969769581,17.9270849363835,0.));
#10420=CARTESIAN_POINT('Ctrl Pts',(3.57255446932205,18.265123941733,0.));
#10421=CARTESIAN_POINT('Ctrl Pts',(3.51033578853423,18.5181384456163,0.));
#10422=CARTESIAN_POINT('Ctrl Pts',(3.46506965370702,18.6813621637974,0.));
#10423=CARTESIAN_POINT('',(6.00933848448158,15.0980247376579,0.));
#10424=CARTESIAN_POINT('Origin',(0.,0.,0.));
#10425=CARTESIAN_POINT('',(8.17732893607301,17.1502563092002,0.));
#10426=CARTESIAN_POINT('Ctrl Pts',(8.17732893607301,17.1502563092002,0.));
#10427=CARTESIAN_POINT('Ctrl Pts',(8.04476736935673,17.0448123137865,0.));
#10428=CARTESIAN_POINT('Ctrl Pts',(7.84571320523309,16.8766905033057,0.));
#10429=CARTESIAN_POINT('Ctrl Pts',(7.59444470905135,16.6414085620714,0.));
#10430=CARTESIAN_POINT('Ctrl Pts',(7.4175377911842,16.4629349257385,0.));
#10431=CARTESIAN_POINT('Ctrl Pts',(7.26219165995678,16.2940809887434,0.));
#10432=CARTESIAN_POINT('Ctrl Pts',(7.12742326811382,16.1361838672874,0.));
#10433=CARTESIAN_POINT('Ctrl Pts',(7.01217619187961,15.9905219781863,0.));
#10434=CARTESIAN_POINT('Ctrl Pts',(6.91534043556368,15.8583036897433,0.));
#10435=CARTESIAN_POINT('Ctrl Pts',(6.83570676658068,15.7406883947777,0.));
#10436=CARTESIAN_POINT('Ctrl Pts',(6.77211692048662,15.6387111659832,0.));
#10437=CARTESIAN_POINT('Ctrl Pts',(6.72790031412623,15.5619248294191,0.));
#10438=CARTESIAN_POINT('Ctrl Pts',(6.69953551835472,15.5083268912119,0.));
#10439=CARTESIAN_POINT('Ctrl Pts',(6.68074830397725,15.4733031879166,0.));
#10440=CARTESIAN_POINT('Ctrl Pts',(6.66297054550541,15.4424051151807,0.));
#10441=CARTESIAN_POINT('Ctrl Pts',(6.63306845520275,15.3933171197393,0.));
#10442=CARTESIAN_POINT('Ctrl Pts',(6.58832104206022,15.3282076647862,0.));
#10443=CARTESIAN_POINT('Ctrl Pts',(6.52246995302225,15.2506809503975,0.));
#10444=CARTESIAN_POINT('Ctrl Pts',(6.44397890908495,15.1795880240196,0.));
#10445=CARTESIAN_POINT('Ctrl Pts',(6.34385243988822,15.1168047097501,0.));
#10446=CARTESIAN_POINT('Ctrl Pts',(6.19604134326089,15.0680440207731,0.));
#10447=CARTESIAN_POINT('Ctrl Pts',(6.07637133495393,15.0769402326058,0.));
#10448=CARTESIAN_POINT('Ctrl Pts',(6.00933848448158,15.0980247376579,0.));
#10449=CARTESIAN_POINT('',(9.06833546026116,16.6962658094608,0.));
#10450=CARTESIAN_POINT('Origin',(0.,-2.16840434497101E-15,0.));
#10451=CARTESIAN_POINT('',(8.68235805704686,13.7360532384391,0.));
#10452=CARTESIAN_POINT('Ctrl Pts',(8.68235805704686,13.7360532384391,0.));
#10453=CARTESIAN_POINT('Ctrl Pts',(8.62589941321482,13.7778907925313,0.));
#10454=CARTESIAN_POINT('Ctrl Pts',(8.54836196063209,13.8694768008521,0.));
#10455=CARTESIAN_POINT('Ctrl Pts',(8.50092900394922,14.0177193038531,0.));
#10456=CARTESIAN_POINT('Ctrl Pts',(8.49286891019844,14.1356264252377,0.));
#10457=CARTESIAN_POINT('Ctrl Pts',(8.50424841775457,14.2409143873564,0.));
#10458=CARTESIAN_POINT('Ctrl Pts',(8.52826254822916,14.3397580968626,0.));
#10459=CARTESIAN_POINT('Ctrl Pts',(8.55463533425733,14.4142298919554,0.));
#10460=CARTESIAN_POINT('Ctrl Pts',(8.57677234909656,14.4672743909627,0.));
#10461=CARTESIAN_POINT('Ctrl Pts',(8.59131991078476,14.4998183311667,0.));
#10462=CARTESIAN_POINT('Ctrl Pts',(8.6086118344139,14.5356039231527,0.));
#10463=CARTESIAN_POINT('Ctrl Pts',(8.63530106864819,14.5900556026053,0.));
#10464=CARTESIAN_POINT('Ctrl Pts',(8.67143265073928,14.6709614647944,0.));
#10465=CARTESIAN_POINT('Ctrl Pts',(8.71655678814373,14.7823474421093,0.));
#10466=CARTESIAN_POINT('Ctrl Pts',(8.76490206435509,14.9159049694657,0.));
#10467=CARTESIAN_POINT('Ctrl Pts',(8.81495027721557,15.0719627020186,0.));
#10468=CARTESIAN_POINT('Ctrl Pts',(8.86505268915084,15.2508174554788,0.));
#10469=CARTESIAN_POINT('Ctrl Pts',(8.91357927057117,15.4526569741556,0.));
#10470=CARTESIAN_POINT('Ctrl Pts',(8.95887481023115,15.6775844882862,0.));
#10471=CARTESIAN_POINT('Ctrl Pts',(8.99927973772153,15.9256093626227,0.));
#10472=CARTESIAN_POINT('Ctrl Pts',(9.04193491022831,16.2671851013731,0.));
#10473=CARTESIAN_POINT('Ctrl Pts',(9.06094720995305,16.5270428237395,0.));
#10474=CARTESIAN_POINT('Ctrl Pts',(9.06833546026116,16.6962658094608,0.));
#10475=CARTESIAN_POINT('',(10.3807667497191,12.5020870932787,0.));
#10476=CARTESIAN_POINT('Origin',(0.,0.,0.));
#10477=CARTESIAN_POINT('',(13.07682262797,13.7839294091566,0.));
#10478=CARTESIAN_POINT('Ctrl Pts',(13.07682262797,13.7839294091566,0.));
#10479=CARTESIAN_POINT('Ctrl Pts',(12.9181650995967,13.7246099871302,0.));
#10480=CARTESIAN_POINT('Ctrl Pts',(12.6769008431476,13.6262277632565,0.));
#10481=CARTESIAN_POINT('Ctrl Pts',(12.3652241842033,13.4801075753502,0.));
#10482=CARTESIAN_POINT('Ctrl Pts',(12.1418243205134,13.3650363045723,0.));
#10483=CARTESIAN_POINT('Ctrl Pts',(11.9419026340297,13.2524512620508,0.));
#10484=CARTESIAN_POINT('Ctrl Pts',(11.764937382884,13.1439278991698,0.));
#10485=CARTESIAN_POINT('Ctrl Pts',(11.6103189008825,13.0410085154728,0.));
#10486=CARTESIAN_POINT('Ctrl Pts',(11.4773649257318,12.9451853450404,0.));
#10487=CARTESIAN_POINT('Ctrl Pts',(11.3652836809863,12.8579347093876,0.));
#10488=CARTESIAN_POINT('Ctrl Pts',(11.2732934467515,12.7805989445416,0.));
#10489=CARTESIAN_POINT('Ctrl Pts',(11.2075126722099,12.7212344815888,0.));
#10490=CARTESIAN_POINT('Ctrl Pts',(11.1639734745885,12.6790250171322,0.));
#10491=CARTESIAN_POINT('Ctrl Pts',(11.1352828524076,12.6515210644081,0.));
#10492=CARTESIAN_POINT('Ctrl Pts',(11.108827169799,12.6276288804813,0.));
#10493=CARTESIAN_POINT('Ctrl Pts',(11.0652195671547,12.5901836766158,0.));
#10494=CARTESIAN_POINT('Ctrl Pts',(11.0025423202231,12.5420886163255,0.));
#10495=CARTESIAN_POINT('Ctrl Pts',(10.9159571406242,12.48870543503,0.));
#10496=CARTESIAN_POINT('Ctrl Pts',(10.8193387993863,12.4453471106187,0.));
#10497=CARTESIAN_POINT('Ctrl Pts',(10.7047117573306,12.4165774110367,0.));
#10498=CARTESIAN_POINT('Ctrl Pts',(10.5490671691512,12.4158793808611,0.));
#10499=CARTESIAN_POINT('Ctrl Pts',(10.4380033085876,12.4613202473787,0.));
#10500=CARTESIAN_POINT('Ctrl Pts',(10.3807667497191,12.5020870932787,0.));
#10501=CARTESIAN_POINT('',(13.7839294091566,13.07682262797,0.));
#10502=CARTESIAN_POINT('Origin',(0.,0.,0.));
#10503=CARTESIAN_POINT('',(12.5020870932787,10.3807667497191,0.));
#10504=CARTESIAN_POINT('Ctrl Pts',(12.5020870932787,10.3807667497191,0.));
#10505=CARTESIAN_POINT('Ctrl Pts',(12.4613202473788,10.4380033085876,0.));
#10506=CARTESIAN_POINT('Ctrl Pts',(12.4158793808611,10.5490671691512,0.));
#10507=CARTESIAN_POINT('Ctrl Pts',(12.4165774110367,10.7047117573306,0.));
#10508=CARTESIAN_POINT('Ctrl Pts',(12.4453471106188,10.8193387993863,0.));
#10509=CARTESIAN_POINT('Ctrl Pts',(12.48870543503,10.9159571406243,0.));
#10510=CARTESIAN_POINT('Ctrl Pts',(12.5420886163255,11.0025423202231,0.));
#10511=CARTESIAN_POINT('Ctrl Pts',(12.5901836766158,11.0652195671547,0.));
#10512=CARTESIAN_POINT('Ctrl Pts',(12.6276288804813,11.1088271697991,0.));
#10513=CARTESIAN_POINT('Ctrl Pts',(12.651521064408,11.1352828524077,0.));
#10514=CARTESIAN_POINT('Ctrl Pts',(12.6790250171322,11.1639734745885,0.));
#10515=CARTESIAN_POINT('Ctrl Pts',(12.7212344815888,11.2075126722099,0.));
#10516=CARTESIAN_POINT('Ctrl Pts',(12.7805989445416,11.2732934467515,0.));
#10517=CARTESIAN_POINT('Ctrl Pts',(12.8579347093876,11.3652836809863,0.));
#10518=CARTESIAN_POINT('Ctrl Pts',(12.9451853450404,11.4773649257318,0.));
#10519=CARTESIAN_POINT('Ctrl Pts',(13.0410085154727,11.6103189008825,0.));
#10520=CARTESIAN_POINT('Ctrl Pts',(13.1439278991698,11.764937382884,0.));
#10521=CARTESIAN_POINT('Ctrl Pts',(13.2524512620507,11.9419026340297,0.));
#10522=CARTESIAN_POINT('Ctrl Pts',(13.3650363045724,12.1418243205134,0.));
#10523=CARTESIAN_POINT('Ctrl Pts',(13.4801075753502,12.3652241842034,0.));
#10524=CARTESIAN_POINT('Ctrl Pts',(13.6262277632565,12.6769008431476,0.));
#10525=CARTESIAN_POINT('Ctrl Pts',(13.7246099871303,12.9181650995967,0.));
#10526=CARTESIAN_POINT('Ctrl Pts',(13.7839294091566,13.07682262797,0.));
#10527=CARTESIAN_POINT('',(13.7360532384392,8.6823580570467,0.));
#10528=CARTESIAN_POINT('Origin',(0.,0.,0.));
#10529=CARTESIAN_POINT('',(16.6962658094608,9.06833546026115,0.));
#10530=CARTESIAN_POINT('Ctrl Pts',(16.6962658094608,9.06833546026115,0.));
#10531=CARTESIAN_POINT('Ctrl Pts',(16.5270428237395,9.06094720995301,0.));
#10532=CARTESIAN_POINT('Ctrl Pts',(16.267185101373,9.0419349102283,0.));
#10533=CARTESIAN_POINT('Ctrl Pts',(15.9256093626227,8.9992797377215,0.));
#10534=CARTESIAN_POINT('Ctrl Pts',(15.6775844882862,8.95887481023115,0.));
#10535=CARTESIAN_POINT('Ctrl Pts',(15.4526569741556,8.9135792705712,0.));
#10536=CARTESIAN_POINT('Ctrl Pts',(15.2508174554787,8.86505268915081,0.));
#10537=CARTESIAN_POINT('Ctrl Pts',(15.0719627020186,8.8149502772156,0.));
#10538=CARTESIAN_POINT('Ctrl Pts',(14.9159049694657,8.76490206435509,0.));
#10539=CARTESIAN_POINT('Ctrl Pts',(14.7823474421092,8.71655678814372,0.));
#10540=CARTESIAN_POINT('Ctrl Pts',(14.6709614647943,8.67143265073928,0.));
#10541=CARTESIAN_POINT('Ctrl Pts',(14.5900556026053,8.63530106864818,0.));
#10542=CARTESIAN_POINT('Ctrl Pts',(14.5356039231526,8.60861183441388,0.));
#10543=CARTESIAN_POINT('Ctrl Pts',(14.4998183311667,8.59131991078479,0.));
#10544=CARTESIAN_POINT('Ctrl Pts',(14.4672743909626,8.57677234909658,0.));
#10545=CARTESIAN_POINT('Ctrl Pts',(14.4142298919554,8.55463533425733,0.));
#10546=CARTESIAN_POINT('Ctrl Pts',(14.3397580968625,8.52826254822916,0.));
#10547=CARTESIAN_POINT('Ctrl Pts',(14.2409143873564,8.50424841775457,0.));
#10548=CARTESIAN_POINT('Ctrl Pts',(14.1356264252376,8.49286891019843,0.));
#10549=CARTESIAN_POINT('Ctrl Pts',(14.0177193038531,8.5009290039492,0.));
#10550=CARTESIAN_POINT('Ctrl Pts',(13.8694768008521,8.54836196063209,0.));
#10551=CARTESIAN_POINT('Ctrl Pts',(13.7778907925312,8.62589941321481,0.));
#10552=CARTESIAN_POINT('Ctrl Pts',(13.7360532384392,8.6823580570467,0.));
#10553=CARTESIAN_POINT('Origin',(2.16840434497101E-15,0.,0.));
#10554=CARTESIAN_POINT('Ctrl Pts',(15.0980247376579,6.00933848448159,7.));
#10555=CARTESIAN_POINT('Ctrl Pts',(15.0980247376579,6.00933848448159,-1.4));
#10556=CARTESIAN_POINT('Ctrl Pts',(15.0769402326058,6.07637133495396,7.));
#10557=CARTESIAN_POINT('Ctrl Pts',(15.0769402326058,6.07637133495396,-1.4));
#10558=CARTESIAN_POINT('Ctrl Pts',(15.0680440207731,6.1960413432609,7.));
#10559=CARTESIAN_POINT('Ctrl Pts',(15.0680440207731,6.1960413432609,-1.4));
#10560=CARTESIAN_POINT('Ctrl Pts',(15.1168047097502,6.34385243988821,7.));
#10561=CARTESIAN_POINT('Ctrl Pts',(15.1168047097502,6.34385243988821,-1.4));
#10562=CARTESIAN_POINT('Ctrl Pts',(15.1795880240196,6.44397890908497,7.));
#10563=CARTESIAN_POINT('Ctrl Pts',(15.1795880240196,6.44397890908497,-1.4));
#10564=CARTESIAN_POINT('Ctrl Pts',(15.2506809503975,6.52246995302229,7.));
#10565=CARTESIAN_POINT('Ctrl Pts',(15.2506809503975,6.52246995302229,-1.4));
#10566=CARTESIAN_POINT('Ctrl Pts',(15.3282076647862,6.58832104206024,7.));
#10567=CARTESIAN_POINT('Ctrl Pts',(15.3282076647862,6.58832104206024,-1.4));
#10568=CARTESIAN_POINT('Ctrl Pts',(15.3933171197393,6.63306845520277,7.));
#10569=CARTESIAN_POINT('Ctrl Pts',(15.3933171197393,6.63306845520277,-1.4));
#10570=CARTESIAN_POINT('Ctrl Pts',(15.4424051151807,6.66297054550544,7.));
#10571=CARTESIAN_POINT('Ctrl Pts',(15.4424051151807,6.66297054550544,-1.4));
#10572=CARTESIAN_POINT('Ctrl Pts',(15.4733031879166,6.68074830397728,7.));
#10573=CARTESIAN_POINT('Ctrl Pts',(15.4733031879166,6.68074830397728,-1.4));
#10574=CARTESIAN_POINT('Ctrl Pts',(15.5083268912119,6.69953551835471,7.));
#10575=CARTESIAN_POINT('Ctrl Pts',(15.5083268912119,6.69953551835471,-1.4));
#10576=CARTESIAN_POINT('Ctrl Pts',(15.5619248294191,6.72790031412625,7.));
#10577=CARTESIAN_POINT('Ctrl Pts',(15.5619248294191,6.72790031412625,-1.4));
#10578=CARTESIAN_POINT('Ctrl Pts',(15.6387111659832,6.77211692048664,7.));
#10579=CARTESIAN_POINT('Ctrl Pts',(15.6387111659832,6.77211692048664,-1.4));
#10580=CARTESIAN_POINT('Ctrl Pts',(15.7406883947778,6.83570676658069,7.));
#10581=CARTESIAN_POINT('Ctrl Pts',(15.7406883947778,6.83570676658069,-1.4));
#10582=CARTESIAN_POINT('Ctrl Pts',(15.8583036897433,6.91534043556371,7.));
#10583=CARTESIAN_POINT('Ctrl Pts',(15.8583036897433,6.91534043556371,-1.4));
#10584=CARTESIAN_POINT('Ctrl Pts',(15.9905219781863,7.01217619187965,7.));
#10585=CARTESIAN_POINT('Ctrl Pts',(15.9905219781863,7.01217619187965,-1.4));
#10586=CARTESIAN_POINT('Ctrl Pts',(16.1361838672874,7.12742326811382,7.));
#10587=CARTESIAN_POINT('Ctrl Pts',(16.1361838672874,7.12742326811382,-1.4));
#10588=CARTESIAN_POINT('Ctrl Pts',(16.2940809887434,7.2621916599568,7.));
#10589=CARTESIAN_POINT('Ctrl Pts',(16.2940809887434,7.2621916599568,-1.4));
#10590=CARTESIAN_POINT('Ctrl Pts',(16.4629349257385,7.41753779118422,7.));
#10591=CARTESIAN_POINT('Ctrl Pts',(16.4629349257385,7.41753779118422,-1.4));
#10592=CARTESIAN_POINT('Ctrl Pts',(16.6414085620714,7.59444470905136,7.));
#10593=CARTESIAN_POINT('Ctrl Pts',(16.6414085620714,7.59444470905136,-1.4));
#10594=CARTESIAN_POINT('Ctrl Pts',(16.8766905033057,7.84571320523309,7.));
#10595=CARTESIAN_POINT('Ctrl Pts',(16.8766905033057,7.84571320523309,-1.4));
#10596=CARTESIAN_POINT('Ctrl Pts',(17.0448123137865,8.04476736935674,7.));
#10597=CARTESIAN_POINT('Ctrl Pts',(17.0448123137865,8.04476736935674,-1.4));
#10598=CARTESIAN_POINT('Ctrl Pts',(17.1502563092004,8.1773289360728,7.));
#10599=CARTESIAN_POINT('Ctrl Pts',(17.1502563092004,8.1773289360728,-1.4));
#10600=CARTESIAN_POINT('',(17.1502563092004,8.17732893607278,7.));
#10601=CARTESIAN_POINT('',(15.0980247376579,6.00933848448158,7.));
#10602=CARTESIAN_POINT('Origin',(2.16840434497101E-15,0.,7.));
#10603=CARTESIAN_POINT('',(16.6962658094608,9.06833546026115,7.));
#10604=CARTESIAN_POINT('Ctrl Pts',(16.6962658094608,9.06833546026116,7.));
#10605=CARTESIAN_POINT('Ctrl Pts',(16.6962658094608,9.06833546026116,-1.39999999999999));
#10606=CARTESIAN_POINT('Ctrl Pts',(16.5270428237395,9.06094720995301,7.));
#10607=CARTESIAN_POINT('Ctrl Pts',(16.5270428237395,9.06094720995301,-1.39999999999999));
#10608=CARTESIAN_POINT('Ctrl Pts',(16.267185101373,9.0419349102283,7.));
#10609=CARTESIAN_POINT('Ctrl Pts',(16.267185101373,9.0419349102283,-1.39999999999999));
#10610=CARTESIAN_POINT('Ctrl Pts',(15.9256093626227,8.9992797377215,7.));
#10611=CARTESIAN_POINT('Ctrl Pts',(15.9256093626227,8.9992797377215,-1.39999999999999));
#10612=CARTESIAN_POINT('Ctrl Pts',(15.6775844882862,8.95887481023115,7.));
#10613=CARTESIAN_POINT('Ctrl Pts',(15.6775844882862,8.95887481023115,-1.39999999999999));
#10614=CARTESIAN_POINT('Ctrl Pts',(15.4526569741556,8.9135792705712,7.));
#10615=CARTESIAN_POINT('Ctrl Pts',(15.4526569741556,8.9135792705712,-1.39999999999999));
#10616=CARTESIAN_POINT('Ctrl Pts',(15.2508174554787,8.86505268915081,7.));
#10617=CARTESIAN_POINT('Ctrl Pts',(15.2508174554787,8.86505268915081,-1.39999999999999));
#10618=CARTESIAN_POINT('Ctrl Pts',(15.0719627020186,8.8149502772156,7.));
#10619=CARTESIAN_POINT('Ctrl Pts',(15.0719627020186,8.8149502772156,-1.39999999999999));
#10620=CARTESIAN_POINT('Ctrl Pts',(14.9159049694657,8.76490206435509,7.));
#10621=CARTESIAN_POINT('Ctrl Pts',(14.9159049694657,8.76490206435509,-1.39999999999999));
#10622=CARTESIAN_POINT('Ctrl Pts',(14.7823474421092,8.71655678814372,7.));
#10623=CARTESIAN_POINT('Ctrl Pts',(14.7823474421092,8.71655678814372,-1.39999999999999));
#10624=CARTESIAN_POINT('Ctrl Pts',(14.6709614647943,8.67143265073928,7.));
#10625=CARTESIAN_POINT('Ctrl Pts',(14.6709614647943,8.67143265073928,-1.39999999999999));
#10626=CARTESIAN_POINT('Ctrl Pts',(14.5900556026053,8.63530106864818,7.));
#10627=CARTESIAN_POINT('Ctrl Pts',(14.5900556026053,8.63530106864818,-1.39999999999999));
#10628=CARTESIAN_POINT('Ctrl Pts',(14.5356039231526,8.60861183441388,7.));
#10629=CARTESIAN_POINT('Ctrl Pts',(14.5356039231526,8.60861183441388,-1.39999999999999));
#10630=CARTESIAN_POINT('Ctrl Pts',(14.4998183311667,8.59131991078479,7.));
#10631=CARTESIAN_POINT('Ctrl Pts',(14.4998183311667,8.59131991078479,-1.39999999999999));
#10632=CARTESIAN_POINT('Ctrl Pts',(14.4672743909626,8.57677234909658,7.));
#10633=CARTESIAN_POINT('Ctrl Pts',(14.4672743909626,8.57677234909658,-1.39999999999999));
#10634=CARTESIAN_POINT('Ctrl Pts',(14.4142298919554,8.55463533425733,7.));
#10635=CARTESIAN_POINT('Ctrl Pts',(14.4142298919554,8.55463533425733,-1.39999999999999));
#10636=CARTESIAN_POINT('Ctrl Pts',(14.3397580968625,8.52826254822916,7.));
#10637=CARTESIAN_POINT('Ctrl Pts',(14.3397580968625,8.52826254822916,-1.39999999999999));
#10638=CARTESIAN_POINT('Ctrl Pts',(14.2409143873564,8.50424841775457,7.));
#10639=CARTESIAN_POINT('Ctrl Pts',(14.2409143873564,8.50424841775457,-1.39999999999999));
#10640=CARTESIAN_POINT('Ctrl Pts',(14.1356264252376,8.49286891019843,7.));
#10641=CARTESIAN_POINT('Ctrl Pts',(14.1356264252376,8.49286891019843,-1.39999999999999));
#10642=CARTESIAN_POINT('Ctrl Pts',(14.0177193038531,8.5009290039492,7.));
#10643=CARTESIAN_POINT('Ctrl Pts',(14.0177193038531,8.5009290039492,-1.39999999999999));
#10644=CARTESIAN_POINT('Ctrl Pts',(13.8694768008521,8.54836196063209,7.));
#10645=CARTESIAN_POINT('Ctrl Pts',(13.8694768008521,8.54836196063209,-1.39999999999999));
#10646=CARTESIAN_POINT('Ctrl Pts',(13.7778907925312,8.62589941321481,7.));
#10647=CARTESIAN_POINT('Ctrl Pts',(13.7778907925312,8.62589941321481,-1.39999999999999));
#10648=CARTESIAN_POINT('Ctrl Pts',(13.7360532384392,8.6823580570467,7.));
#10649=CARTESIAN_POINT('Ctrl Pts',(13.7360532384392,8.6823580570467,-1.39999999999999));
#10650=CARTESIAN_POINT('',(13.7360532384392,8.6823580570467,7.));
#10651=CARTESIAN_POINT('Origin',(0.,0.,7.));
#10652=CARTESIAN_POINT('',(12.5020870932787,10.3807667497191,7.));
#10653=CARTESIAN_POINT('Ctrl Pts',(12.5020870932787,10.3807667497191,7.));
#10654=CARTESIAN_POINT('Ctrl Pts',(12.5020870932787,10.3807667497191,-1.4));
#10655=CARTESIAN_POINT('Ctrl Pts',(12.4613202473788,10.4380033085876,7.));
#10656=CARTESIAN_POINT('Ctrl Pts',(12.4613202473788,10.4380033085876,-1.4));
#10657=CARTESIAN_POINT('Ctrl Pts',(12.4158793808611,10.5490671691512,7.));
#10658=CARTESIAN_POINT('Ctrl Pts',(12.4158793808611,10.5490671691512,-1.4));
#10659=CARTESIAN_POINT('Ctrl Pts',(12.4165774110367,10.7047117573306,7.));
#10660=CARTESIAN_POINT('Ctrl Pts',(12.4165774110367,10.7047117573306,-1.4));
#10661=CARTESIAN_POINT('Ctrl Pts',(12.4453471106188,10.8193387993863,7.));
#10662=CARTESIAN_POINT('Ctrl Pts',(12.4453471106188,10.8193387993863,-1.4));
#10663=CARTESIAN_POINT('Ctrl Pts',(12.48870543503,10.9159571406243,7.));
#10664=CARTESIAN_POINT('Ctrl Pts',(12.48870543503,10.9159571406243,-1.4));
#10665=CARTESIAN_POINT('Ctrl Pts',(12.5420886163255,11.0025423202231,7.));
#10666=CARTESIAN_POINT('Ctrl Pts',(12.5420886163255,11.0025423202231,-1.4));
#10667=CARTESIAN_POINT('Ctrl Pts',(12.5901836766158,11.0652195671547,7.));
#10668=CARTESIAN_POINT('Ctrl Pts',(12.5901836766158,11.0652195671547,-1.4));
#10669=CARTESIAN_POINT('Ctrl Pts',(12.6276288804813,11.1088271697991,7.));
#10670=CARTESIAN_POINT('Ctrl Pts',(12.6276288804813,11.1088271697991,-1.4));
#10671=CARTESIAN_POINT('Ctrl Pts',(12.651521064408,11.1352828524077,7.));
#10672=CARTESIAN_POINT('Ctrl Pts',(12.651521064408,11.1352828524077,-1.4));
#10673=CARTESIAN_POINT('Ctrl Pts',(12.6790250171322,11.1639734745885,7.));
#10674=CARTESIAN_POINT('Ctrl Pts',(12.6790250171322,11.1639734745885,-1.4));
#10675=CARTESIAN_POINT('Ctrl Pts',(12.7212344815888,11.2075126722099,7.));
#10676=CARTESIAN_POINT('Ctrl Pts',(12.7212344815888,11.2075126722099,-1.4));
#10677=CARTESIAN_POINT('Ctrl Pts',(12.7805989445416,11.2732934467515,7.));
#10678=CARTESIAN_POINT('Ctrl Pts',(12.7805989445416,11.2732934467515,-1.4));
#10679=CARTESIAN_POINT('Ctrl Pts',(12.8579347093876,11.3652836809863,7.));
#10680=CARTESIAN_POINT('Ctrl Pts',(12.8579347093876,11.3652836809863,-1.4));
#10681=CARTESIAN_POINT('Ctrl Pts',(12.9451853450404,11.4773649257318,7.));
#10682=CARTESIAN_POINT('Ctrl Pts',(12.9451853450404,11.4773649257318,-1.4));
#10683=CARTESIAN_POINT('Ctrl Pts',(13.0410085154727,11.6103189008825,7.));
#10684=CARTESIAN_POINT('Ctrl Pts',(13.0410085154727,11.6103189008825,-1.4));
#10685=CARTESIAN_POINT('Ctrl Pts',(13.1439278991698,11.764937382884,7.));
#10686=CARTESIAN_POINT('Ctrl Pts',(13.1439278991698,11.764937382884,-1.4));
#10687=CARTESIAN_POINT('Ctrl Pts',(13.2524512620507,11.9419026340297,7.));
#10688=CARTESIAN_POINT('Ctrl Pts',(13.2524512620507,11.9419026340297,-1.4));
#10689=CARTESIAN_POINT('Ctrl Pts',(13.3650363045724,12.1418243205134,7.));
#10690=CARTESIAN_POINT('Ctrl Pts',(13.3650363045724,12.1418243205134,-1.4));
#10691=CARTESIAN_POINT('Ctrl Pts',(13.4801075753502,12.3652241842034,7.));
#10692=CARTESIAN_POINT('Ctrl Pts',(13.4801075753502,12.3652241842034,-1.4));
#10693=CARTESIAN_POINT('Ctrl Pts',(13.6262277632565,12.6769008431476,7.));
#10694=CARTESIAN_POINT('Ctrl Pts',(13.6262277632565,12.6769008431476,-1.4));
#10695=CARTESIAN_POINT('Ctrl Pts',(13.7246099871303,12.9181650995967,7.));
#10696=CARTESIAN_POINT('Ctrl Pts',(13.7246099871303,12.9181650995967,-1.4));
#10697=CARTESIAN_POINT('Ctrl Pts',(13.7839294091566,13.07682262797,7.));
#10698=CARTESIAN_POINT('Ctrl Pts',(13.7839294091566,13.07682262797,-1.4));
#10699=CARTESIAN_POINT('',(13.7839294091566,13.07682262797,7.));
#10700=CARTESIAN_POINT('Origin',(0.,0.,7.));
#10701=CARTESIAN_POINT('',(13.07682262797,13.7839294091566,7.));
#10702=CARTESIAN_POINT('Ctrl Pts',(13.07682262797,13.7839294091566,7.));
#10703=CARTESIAN_POINT('Ctrl Pts',(13.07682262797,13.7839294091566,-1.39999999999998));
#10704=CARTESIAN_POINT('Ctrl Pts',(12.9181650995967,13.7246099871302,7.));
#10705=CARTESIAN_POINT('Ctrl Pts',(12.9181650995967,13.7246099871302,-1.39999999999998));
#10706=CARTESIAN_POINT('Ctrl Pts',(12.6769008431476,13.6262277632565,7.));
#10707=CARTESIAN_POINT('Ctrl Pts',(12.6769008431476,13.6262277632565,-1.39999999999998));
#10708=CARTESIAN_POINT('Ctrl Pts',(12.3652241842033,13.4801075753502,7.));
#10709=CARTESIAN_POINT('Ctrl Pts',(12.3652241842033,13.4801075753502,-1.39999999999998));
#10710=CARTESIAN_POINT('Ctrl Pts',(12.1418243205134,13.3650363045723,7.));
#10711=CARTESIAN_POINT('Ctrl Pts',(12.1418243205134,13.3650363045723,-1.39999999999998));
#10712=CARTESIAN_POINT('Ctrl Pts',(11.9419026340297,13.2524512620508,7.));
#10713=CARTESIAN_POINT('Ctrl Pts',(11.9419026340297,13.2524512620508,-1.39999999999998));
#10714=CARTESIAN_POINT('Ctrl Pts',(11.764937382884,13.1439278991698,7.));
#10715=CARTESIAN_POINT('Ctrl Pts',(11.764937382884,13.1439278991698,-1.39999999999998));
#10716=CARTESIAN_POINT('Ctrl Pts',(11.6103189008825,13.0410085154728,7.));
#10717=CARTESIAN_POINT('Ctrl Pts',(11.6103189008825,13.0410085154728,-1.39999999999998));
#10718=CARTESIAN_POINT('Ctrl Pts',(11.4773649257318,12.9451853450404,7.));
#10719=CARTESIAN_POINT('Ctrl Pts',(11.4773649257318,12.9451853450404,-1.39999999999998));
#10720=CARTESIAN_POINT('Ctrl Pts',(11.3652836809863,12.8579347093876,7.));
#10721=CARTESIAN_POINT('Ctrl Pts',(11.3652836809863,12.8579347093876,-1.39999999999998));
#10722=CARTESIAN_POINT('Ctrl Pts',(11.2732934467515,12.7805989445416,7.));
#10723=CARTESIAN_POINT('Ctrl Pts',(11.2732934467515,12.7805989445416,-1.39999999999998));
#10724=CARTESIAN_POINT('Ctrl Pts',(11.2075126722099,12.7212344815888,7.));
#10725=CARTESIAN_POINT('Ctrl Pts',(11.2075126722099,12.7212344815888,-1.39999999999998));
#10726=CARTESIAN_POINT('Ctrl Pts',(11.1639734745885,12.6790250171322,7.));
#10727=CARTESIAN_POINT('Ctrl Pts',(11.1639734745885,12.6790250171322,-1.39999999999998));
#10728=CARTESIAN_POINT('Ctrl Pts',(11.1352828524076,12.6515210644081,7.));
#10729=CARTESIAN_POINT('Ctrl Pts',(11.1352828524076,12.6515210644081,-1.39999999999998));
#10730=CARTESIAN_POINT('Ctrl Pts',(11.108827169799,12.6276288804813,7.));
#10731=CARTESIAN_POINT('Ctrl Pts',(11.108827169799,12.6276288804813,-1.39999999999998));
#10732=CARTESIAN_POINT('Ctrl Pts',(11.0652195671547,12.5901836766158,7.));
#10733=CARTESIAN_POINT('Ctrl Pts',(11.0652195671547,12.5901836766158,-1.39999999999998));
#10734=CARTESIAN_POINT('Ctrl Pts',(11.0025423202231,12.5420886163255,7.));
#10735=CARTESIAN_POINT('Ctrl Pts',(11.0025423202231,12.5420886163255,-1.39999999999998));
#10736=CARTESIAN_POINT('Ctrl Pts',(10.9159571406242,12.48870543503,7.));
#10737=CARTESIAN_POINT('Ctrl Pts',(10.9159571406242,12.48870543503,-1.39999999999998));
#10738=CARTESIAN_POINT('Ctrl Pts',(10.8193387993863,12.4453471106187,7.));
#10739=CARTESIAN_POINT('Ctrl Pts',(10.8193387993863,12.4453471106187,-1.39999999999998));
#10740=CARTESIAN_POINT('Ctrl Pts',(10.7047117573306,12.4165774110367,7.));
#10741=CARTESIAN_POINT('Ctrl Pts',(10.7047117573306,12.4165774110367,-1.39999999999998));
#10742=CARTESIAN_POINT('Ctrl Pts',(10.5490671691512,12.4158793808611,7.));
#10743=CARTESIAN_POINT('Ctrl Pts',(10.5490671691512,12.4158793808611,-1.39999999999998));
#10744=CARTESIAN_POINT('Ctrl Pts',(10.4380033085876,12.4613202473787,7.));
#10745=CARTESIAN_POINT('Ctrl Pts',(10.4380033085876,12.4613202473787,-1.39999999999998));
#10746=CARTESIAN_POINT('Ctrl Pts',(10.3807667497191,12.5020870932787,7.));
#10747=CARTESIAN_POINT('Ctrl Pts',(10.3807667497191,12.5020870932787,-1.39999999999998));
#10748=CARTESIAN_POINT('',(10.3807667497191,12.5020870932787,7.));
#10749=CARTESIAN_POINT('Origin',(0.,0.,7.));
#10750=CARTESIAN_POINT('',(8.68235805704686,13.7360532384391,7.));
#10751=CARTESIAN_POINT('Ctrl Pts',(8.68235805704669,13.7360532384392,7.));
#10752=CARTESIAN_POINT('Ctrl Pts',(8.68235805704669,13.7360532384392,-1.4));
#10753=CARTESIAN_POINT('Ctrl Pts',(8.62589941321482,13.7778907925313,7.));
#10754=CARTESIAN_POINT('Ctrl Pts',(8.62589941321482,13.7778907925313,-1.4));
#10755=CARTESIAN_POINT('Ctrl Pts',(8.54836196063209,13.8694768008521,7.));
#10756=CARTESIAN_POINT('Ctrl Pts',(8.54836196063209,13.8694768008521,-1.4));
#10757=CARTESIAN_POINT('Ctrl Pts',(8.50092900394922,14.0177193038531,7.));
#10758=CARTESIAN_POINT('Ctrl Pts',(8.50092900394922,14.0177193038531,-1.4));
#10759=CARTESIAN_POINT('Ctrl Pts',(8.49286891019844,14.1356264252377,7.));
#10760=CARTESIAN_POINT('Ctrl Pts',(8.49286891019844,14.1356264252377,-1.4));
#10761=CARTESIAN_POINT('Ctrl Pts',(8.50424841775457,14.2409143873564,7.));
#10762=CARTESIAN_POINT('Ctrl Pts',(8.50424841775457,14.2409143873564,-1.4));
#10763=CARTESIAN_POINT('Ctrl Pts',(8.52826254822916,14.3397580968626,7.));
#10764=CARTESIAN_POINT('Ctrl Pts',(8.52826254822916,14.3397580968626,-1.4));
#10765=CARTESIAN_POINT('Ctrl Pts',(8.55463533425733,14.4142298919554,7.));
#10766=CARTESIAN_POINT('Ctrl Pts',(8.55463533425733,14.4142298919554,-1.4));
#10767=CARTESIAN_POINT('Ctrl Pts',(8.57677234909656,14.4672743909627,7.));
#10768=CARTESIAN_POINT('Ctrl Pts',(8.57677234909656,14.4672743909627,-1.4));
#10769=CARTESIAN_POINT('Ctrl Pts',(8.59131991078476,14.4998183311667,7.));
#10770=CARTESIAN_POINT('Ctrl Pts',(8.59131991078476,14.4998183311667,-1.4));
#10771=CARTESIAN_POINT('Ctrl Pts',(8.6086118344139,14.5356039231527,7.));
#10772=CARTESIAN_POINT('Ctrl Pts',(8.6086118344139,14.5356039231527,-1.4));
#10773=CARTESIAN_POINT('Ctrl Pts',(8.63530106864819,14.5900556026053,7.));
#10774=CARTESIAN_POINT('Ctrl Pts',(8.63530106864819,14.5900556026053,-1.4));
#10775=CARTESIAN_POINT('Ctrl Pts',(8.67143265073928,14.6709614647944,7.));
#10776=CARTESIAN_POINT('Ctrl Pts',(8.67143265073928,14.6709614647944,-1.4));
#10777=CARTESIAN_POINT('Ctrl Pts',(8.71655678814373,14.7823474421093,7.));
#10778=CARTESIAN_POINT('Ctrl Pts',(8.71655678814373,14.7823474421093,-1.4));
#10779=CARTESIAN_POINT('Ctrl Pts',(8.76490206435509,14.9159049694657,7.));
#10780=CARTESIAN_POINT('Ctrl Pts',(8.76490206435509,14.9159049694657,-1.4));
#10781=CARTESIAN_POINT('Ctrl Pts',(8.81495027721557,15.0719627020186,7.));
#10782=CARTESIAN_POINT('Ctrl Pts',(8.81495027721557,15.0719627020186,-1.4));
#10783=CARTESIAN_POINT('Ctrl Pts',(8.86505268915084,15.2508174554788,7.));
#10784=CARTESIAN_POINT('Ctrl Pts',(8.86505268915084,15.2508174554788,-1.4));
#10785=CARTESIAN_POINT('Ctrl Pts',(8.91357927057117,15.4526569741556,7.));
#10786=CARTESIAN_POINT('Ctrl Pts',(8.91357927057117,15.4526569741556,-1.4));
#10787=CARTESIAN_POINT('Ctrl Pts',(8.95887481023115,15.6775844882862,7.));
#10788=CARTESIAN_POINT('Ctrl Pts',(8.95887481023115,15.6775844882862,-1.4));
#10789=CARTESIAN_POINT('Ctrl Pts',(8.99927973772153,15.9256093626227,7.));
#10790=CARTESIAN_POINT('Ctrl Pts',(8.99927973772153,15.9256093626227,-1.4));
#10791=CARTESIAN_POINT('Ctrl Pts',(9.04193491022831,16.2671851013731,7.));
#10792=CARTESIAN_POINT('Ctrl Pts',(9.04193491022831,16.2671851013731,-1.4));
#10793=CARTESIAN_POINT('Ctrl Pts',(9.06094720995305,16.5270428237395,7.));
#10794=CARTESIAN_POINT('Ctrl Pts',(9.06094720995305,16.5270428237395,-1.4));
#10795=CARTESIAN_POINT('Ctrl Pts',(9.06833546026116,16.6962658094608,7.));
#10796=CARTESIAN_POINT('Ctrl Pts',(9.06833546026116,16.6962658094608,-1.4));
#10797=CARTESIAN_POINT('',(9.06833546026116,16.6962658094608,7.));
#10798=CARTESIAN_POINT('Origin',(0.,-2.16840434497101E-15,7.));
#10799=CARTESIAN_POINT('',(8.17732893607301,17.1502563092002,7.));
#10800=CARTESIAN_POINT('Ctrl Pts',(8.17732893607279,17.1502563092004,7.));
#10801=CARTESIAN_POINT('Ctrl Pts',(8.17732893607279,17.1502563092004,-1.39999999999999));
#10802=CARTESIAN_POINT('Ctrl Pts',(8.04476736935673,17.0448123137865,7.));
#10803=CARTESIAN_POINT('Ctrl Pts',(8.04476736935673,17.0448123137865,-1.39999999999999));
#10804=CARTESIAN_POINT('Ctrl Pts',(7.84571320523309,16.8766905033057,7.));
#10805=CARTESIAN_POINT('Ctrl Pts',(7.84571320523309,16.8766905033057,-1.39999999999999));
#10806=CARTESIAN_POINT('Ctrl Pts',(7.59444470905135,16.6414085620714,7.));
#10807=CARTESIAN_POINT('Ctrl Pts',(7.59444470905135,16.6414085620714,-1.39999999999999));
#10808=CARTESIAN_POINT('Ctrl Pts',(7.4175377911842,16.4629349257385,7.));
#10809=CARTESIAN_POINT('Ctrl Pts',(7.4175377911842,16.4629349257385,-1.39999999999999));
#10810=CARTESIAN_POINT('Ctrl Pts',(7.26219165995678,16.2940809887434,7.));
#10811=CARTESIAN_POINT('Ctrl Pts',(7.26219165995678,16.2940809887434,-1.39999999999999));
#10812=CARTESIAN_POINT('Ctrl Pts',(7.12742326811382,16.1361838672874,7.));
#10813=CARTESIAN_POINT('Ctrl Pts',(7.12742326811382,16.1361838672874,-1.39999999999999));
#10814=CARTESIAN_POINT('Ctrl Pts',(7.01217619187961,15.9905219781863,7.));
#10815=CARTESIAN_POINT('Ctrl Pts',(7.01217619187961,15.9905219781863,-1.39999999999999));
#10816=CARTESIAN_POINT('Ctrl Pts',(6.91534043556368,15.8583036897433,7.));
#10817=CARTESIAN_POINT('Ctrl Pts',(6.91534043556368,15.8583036897433,-1.39999999999999));
#10818=CARTESIAN_POINT('Ctrl Pts',(6.83570676658068,15.7406883947777,7.));
#10819=CARTESIAN_POINT('Ctrl Pts',(6.83570676658068,15.7406883947777,-1.39999999999999));
#10820=CARTESIAN_POINT('Ctrl Pts',(6.77211692048662,15.6387111659832,7.));
#10821=CARTESIAN_POINT('Ctrl Pts',(6.77211692048662,15.6387111659832,-1.39999999999999));
#10822=CARTESIAN_POINT('Ctrl Pts',(6.72790031412623,15.5619248294191,7.));
#10823=CARTESIAN_POINT('Ctrl Pts',(6.72790031412623,15.5619248294191,-1.39999999999999));
#10824=CARTESIAN_POINT('Ctrl Pts',(6.69953551835472,15.5083268912119,7.));
#10825=CARTESIAN_POINT('Ctrl Pts',(6.69953551835472,15.5083268912119,-1.39999999999999));
#10826=CARTESIAN_POINT('Ctrl Pts',(6.68074830397725,15.4733031879166,7.));
#10827=CARTESIAN_POINT('Ctrl Pts',(6.68074830397725,15.4733031879166,-1.39999999999999));
#10828=CARTESIAN_POINT('Ctrl Pts',(6.66297054550541,15.4424051151807,7.));
#10829=CARTESIAN_POINT('Ctrl Pts',(6.66297054550541,15.4424051151807,-1.39999999999999));
#10830=CARTESIAN_POINT('Ctrl Pts',(6.63306845520275,15.3933171197393,7.));
#10831=CARTESIAN_POINT('Ctrl Pts',(6.63306845520275,15.3933171197393,-1.39999999999999));
#10832=CARTESIAN_POINT('Ctrl Pts',(6.58832104206022,15.3282076647862,7.));
#10833=CARTESIAN_POINT('Ctrl Pts',(6.58832104206022,15.3282076647862,-1.39999999999999));
#10834=CARTESIAN_POINT('Ctrl Pts',(6.52246995302225,15.2506809503975,7.));
#10835=CARTESIAN_POINT('Ctrl Pts',(6.52246995302225,15.2506809503975,-1.39999999999999));
#10836=CARTESIAN_POINT('Ctrl Pts',(6.44397890908495,15.1795880240196,7.));
#10837=CARTESIAN_POINT('Ctrl Pts',(6.44397890908495,15.1795880240196,-1.39999999999999));
#10838=CARTESIAN_POINT('Ctrl Pts',(6.34385243988822,15.1168047097501,7.));
#10839=CARTESIAN_POINT('Ctrl Pts',(6.34385243988822,15.1168047097501,-1.39999999999999));
#10840=CARTESIAN_POINT('Ctrl Pts',(6.19604134326089,15.0680440207731,7.));
#10841=CARTESIAN_POINT('Ctrl Pts',(6.19604134326089,15.0680440207731,-1.39999999999999));
#10842=CARTESIAN_POINT('Ctrl Pts',(6.07637133495393,15.0769402326058,7.));
#10843=CARTESIAN_POINT('Ctrl Pts',(6.07637133495393,15.0769402326058,-1.39999999999999));
#10844=CARTESIAN_POINT('Ctrl Pts',(6.00933848448158,15.0980247376579,7.));
#10845=CARTESIAN_POINT('Ctrl Pts',(6.00933848448158,15.0980247376579,-1.39999999999999));
#10846=CARTESIAN_POINT('',(6.00933848448158,15.0980247376579,7.));
#10847=CARTESIAN_POINT('Origin',(0.,0.,7.));
#10848=CARTESIAN_POINT('',(4.01273932064543,15.7467591314704,7.));
#10849=CARTESIAN_POINT('Ctrl Pts',(4.01273932064519,15.7467591314705,7.));
#10850=CARTESIAN_POINT('Ctrl Pts',(4.01273932064519,15.7467591314705,-1.40000000000002));
#10851=CARTESIAN_POINT('Ctrl Pts',(3.94611544431017,15.7691023294921,7.));
#10852=CARTESIAN_POINT('Ctrl Pts',(3.94611544431017,15.7691023294921,-1.40000000000002));
#10853=CARTESIAN_POINT('Ctrl Pts',(3.84407131175635,15.8322454089585,7.));
#10854=CARTESIAN_POINT('Ctrl Pts',(3.84407131175635,15.8322454089585,-1.40000000000002));
#10855=CARTESIAN_POINT('Ctrl Pts',(3.75315043649997,15.9585748177211,7.));
#10856=CARTESIAN_POINT('Ctrl Pts',(3.75315043649997,15.9585748177211,-1.40000000000002));
#10857=CARTESIAN_POINT('Ctrl Pts',(3.70904952755068,16.0682204478862,7.));
#10858=CARTESIAN_POINT('Ctrl Pts',(3.70904952755068,16.0682204478862,-1.40000000000002));
#10859=CARTESIAN_POINT('Ctrl Pts',(3.68733631276637,16.1718717115691,7.));
#10860=CARTESIAN_POINT('Ctrl Pts',(3.68733631276637,16.1718717115691,-1.40000000000002));
#10861=CARTESIAN_POINT('Ctrl Pts',(3.67963072201293,16.2732984400116,7.));
#10862=CARTESIAN_POINT('Ctrl Pts',(3.67963072201293,16.2732984400116,-1.40000000000002));
#10863=CARTESIAN_POINT('Ctrl Pts',(3.68169968173257,16.3522749650866,7.));
#10864=CARTESIAN_POINT('Ctrl Pts',(3.68169968173257,16.3522749650866,-1.40000000000002));
#10865=CARTESIAN_POINT('Ctrl Pts',(3.68636158229542,16.409563995311,7.));
#10866=CARTESIAN_POINT('Ctrl Pts',(3.68636158229542,16.409563995311,-1.40000000000002));
#10867=CARTESIAN_POINT('Ctrl Pts',(3.69014050504822,16.4450105654964,7.));
#10868=CARTESIAN_POINT('Ctrl Pts',(3.69014050504822,16.4450105654964,-1.40000000000002));
#10869=CARTESIAN_POINT('Ctrl Pts',(3.69552774561756,16.4843881842109,7.));
#10870=CARTESIAN_POINT('Ctrl Pts',(3.69552774561756,16.4843881842109,-1.40000000000002));
#10871=CARTESIAN_POINT('Ctrl Pts',(3.70408422142788,16.5444222357228,7.));
#10872=CARTESIAN_POINT('Ctrl Pts',(3.70408422142788,16.5444222357228,-1.40000000000002));
#10873=CARTESIAN_POINT('Ctrl Pts',(3.71344611165869,16.632533556064,7.));
#10874=CARTESIAN_POINT('Ctrl Pts',(3.71344611165869,16.632533556064,-1.40000000000002));
#10875=CARTESIAN_POINT('Ctrl Pts',(3.72194155665403,16.7524120409277,7.));
#10876=CARTESIAN_POINT('Ctrl Pts',(3.72194155665403,16.7524120409277,-1.40000000000002));
#10877=CARTESIAN_POINT('Ctrl Pts',(3.7266491009471,16.8943723095674,7.));
#10878=CARTESIAN_POINT('Ctrl Pts',(3.7266491009471,16.8943723095674,-1.40000000000002));
#10879=CARTESIAN_POINT('Ctrl Pts',(3.72602328845452,17.0582577813421,7.));
#10880=CARTESIAN_POINT('Ctrl Pts',(3.72602328845452,17.0582577813421,-1.40000000000002));
#10881=CARTESIAN_POINT('Ctrl Pts',(3.71840435546373,17.2438412568379,7.));
#10882=CARTESIAN_POINT('Ctrl Pts',(3.71840435546373,17.2438412568379,-1.40000000000002));
#10883=CARTESIAN_POINT('Ctrl Pts',(3.70218403552947,17.4507975846592,7.));
#10884=CARTESIAN_POINT('Ctrl Pts',(3.70218403552947,17.4507975846592,-1.40000000000002));
#10885=CARTESIAN_POINT('Ctrl Pts',(3.67575622931333,17.6787134541915,7.));
#10886=CARTESIAN_POINT('Ctrl Pts',(3.67575622931333,17.6787134541915,-1.40000000000002));
#10887=CARTESIAN_POINT('Ctrl Pts',(3.63753969769581,17.9270849363835,7.));
#10888=CARTESIAN_POINT('Ctrl Pts',(3.63753969769581,17.9270849363835,-1.40000000000002));
#10889=CARTESIAN_POINT('Ctrl Pts',(3.57255446932205,18.265123941733,7.));
#10890=CARTESIAN_POINT('Ctrl Pts',(3.57255446932205,18.265123941733,-1.40000000000002));
#10891=CARTESIAN_POINT('Ctrl Pts',(3.51033578853423,18.5181384456163,7.));
#10892=CARTESIAN_POINT('Ctrl Pts',(3.51033578853423,18.5181384456163,-1.40000000000002));
#10893=CARTESIAN_POINT('Ctrl Pts',(3.46506965370702,18.6813621637974,7.));
#10894=CARTESIAN_POINT('Ctrl Pts',(3.46506965370702,18.6813621637974,-1.40000000000002));
#10895=CARTESIAN_POINT('',(3.46506965370702,18.6813621637974,7.));
#10896=CARTESIAN_POINT('Origin',(0.,8.67361737988404E-16,7.));
#10897=CARTESIAN_POINT('',(2.47738131311212,18.8377966288375,7.));
#10898=CARTESIAN_POINT('Ctrl Pts',(2.47738131311188,18.8377966288376,7.));
#10899=CARTESIAN_POINT('Ctrl Pts',(2.47738131311188,18.8377966288376,-1.39999999999999));
#10900=CARTESIAN_POINT('Ctrl Pts',(2.38389175781397,18.6965496529788,7.));
#10901=CARTESIAN_POINT('Ctrl Pts',(2.38389175781397,18.6965496529788,-1.39999999999999));
#10902=CARTESIAN_POINT('Ctrl Pts',(2.24653249449213,18.4751451900744,7.));
#10903=CARTESIAN_POINT('Ctrl Pts',(2.24653249449213,18.4751451900744,-1.39999999999999));
#10904=CARTESIAN_POINT('Ctrl Pts',(2.08026807216976,18.1737325312257,7.));
#10905=CARTESIAN_POINT('Ctrl Pts',(2.08026807216976,18.1737325312257,-1.39999999999999));
#10906=CARTESIAN_POINT('Ctrl Pts',(1.96717098182927,17.949326772361,7.));
#10907=CARTESIAN_POINT('Ctrl Pts',(1.96717098182927,17.949326772361,-1.39999999999999));
#10908=CARTESIAN_POINT('Ctrl Pts',(1.87160676754279,17.7407325407201,7.));
#10909=CARTESIAN_POINT('Ctrl Pts',(1.87160676754279,17.7407325407201,-1.39999999999999));
#10910=CARTESIAN_POINT('Ctrl Pts',(1.79222730418274,17.548917731071,7.));
#10911=CARTESIAN_POINT('Ctrl Pts',(1.79222730418274,17.548917731071,-1.39999999999999));
#10912=CARTESIAN_POINT('Ctrl Pts',(1.72763282051121,17.3747717371572,7.));
#10913=CARTESIAN_POINT('Ctrl Pts',(1.72763282051121,17.3747717371572,-1.39999999999999));
#10914=CARTESIAN_POINT('Ctrl Pts',(1.67639424155266,17.2191007779952,7.));
#10915=CARTESIAN_POINT('Ctrl Pts',(1.67639424155266,17.2191007779952,-1.39999999999999));
#10916=CARTESIAN_POINT('Ctrl Pts',(1.63700324669265,17.0826338282621,7.));
#10917=CARTESIAN_POINT('Ctrl Pts',(1.63700324669265,17.0826338282621,-1.39999999999999));
#10918=CARTESIAN_POINT('Ctrl Pts',(1.60803840593148,16.9659973771906,7.));
#10919=CARTESIAN_POINT('Ctrl Pts',(1.60803840593148,16.9659973771906,-1.39999999999999));
#10920=CARTESIAN_POINT('Ctrl Pts',(1.58971419725808,16.8793055486399,7.));
#10921=CARTESIAN_POINT('Ctrl Pts',(1.58971419725808,16.8793055486399,-1.39999999999999));
#10922=CARTESIAN_POINT('Ctrl Pts',(1.57930034717568,16.8195656763126,7.));
#10923=CARTESIAN_POINT('Ctrl Pts',(1.57930034717568,16.8195656763126,-1.39999999999999));
#10924=CARTESIAN_POINT('Ctrl Pts',(1.57225556404314,16.7804505865492,7.));
#10925=CARTESIAN_POINT('Ctrl Pts',(1.57225556404314,16.7804505865492,-1.39999999999999));
#10926=CARTESIAN_POINT('Ctrl Pts',(1.5648959405722,16.7455711436431,7.));
#10927=CARTESIAN_POINT('Ctrl Pts',(1.5648959405722,16.7455711436431,-1.39999999999999));
#10928=CARTESIAN_POINT('Ctrl Pts',(1.5516263875502,16.6896454316358,7.));
#10929=CARTESIAN_POINT('Ctrl Pts',(1.5516263875502,16.6896454316358,-1.39999999999999));
#10930=CARTESIAN_POINT('Ctrl Pts',(1.52918899676866,16.6138949491149,7.));
#10931=CARTESIAN_POINT('Ctrl Pts',(1.52918899676866,16.6138949491149,-1.39999999999999));
#10932=CARTESIAN_POINT('Ctrl Pts',(1.49051796169813,16.5198135565977,7.));
#10933=CARTESIAN_POINT('Ctrl Pts',(1.49051796169813,16.5198135565977,-1.39999999999999));
#10934=CARTESIAN_POINT('Ctrl Pts',(1.43783746532136,16.4279450992207,7.));
#10935=CARTESIAN_POINT('Ctrl Pts',(1.43783746532136,16.4279450992207,-1.39999999999999));
#10936=CARTESIAN_POINT('Ctrl Pts',(1.36201264541063,16.3372938385016,7.));
#10937=CARTESIAN_POINT('Ctrl Pts',(1.36201264541063,16.3372938385016,-1.39999999999999));
#10938=CARTESIAN_POINT('Ctrl Pts',(1.23650382033381,16.2452435266959,7.));
#10939=CARTESIAN_POINT('Ctrl Pts',(1.23650382033381,16.2452435266959,-1.39999999999999));
#10940=CARTESIAN_POINT('Ctrl Pts',(1.11994179848653,16.2167242606458,7.));
#10941=CARTESIAN_POINT('Ctrl Pts',(1.11994179848653,16.2167242606458,-1.39999999999999));
#10942=CARTESIAN_POINT('Ctrl Pts',(1.04967429885989,16.2160625265911,7.));
#10943=CARTESIAN_POINT('Ctrl Pts',(1.04967429885989,16.2160625265911,-1.39999999999999));
#10944=CARTESIAN_POINT('',(1.04967429885989,16.2160625265911,7.));
#10945=CARTESIAN_POINT('Origin',(0.,0.,7.));
#10946=CARTESIAN_POINT('',(-1.04967429885962,16.2160625265911,7.));
#10947=CARTESIAN_POINT('Ctrl Pts',(-1.04967429885986,16.2160625265911,7.));
#10948=CARTESIAN_POINT('Ctrl Pts',(-1.04967429885986,16.2160625265911,-1.4));
#10949=CARTESIAN_POINT('Ctrl Pts',(-1.11994179848651,16.2167242606459,7.));
#10950=CARTESIAN_POINT('Ctrl Pts',(-1.11994179848651,16.2167242606459,-1.4));
#10951=CARTESIAN_POINT('Ctrl Pts',(-1.23650382033378,16.2452435266959,7.));
#10952=CARTESIAN_POINT('Ctrl Pts',(-1.23650382033378,16.2452435266959,-1.4));
#10953=CARTESIAN_POINT('Ctrl Pts',(-1.36201264541058,16.3372938385016,7.));
#10954=CARTESIAN_POINT('Ctrl Pts',(-1.36201264541058,16.3372938385016,-1.4));
#10955=CARTESIAN_POINT('Ctrl Pts',(-1.43783746532133,16.4279450992208,7.));
#10956=CARTESIAN_POINT('Ctrl Pts',(-1.43783746532133,16.4279450992208,-1.4));
#10957=CARTESIAN_POINT('Ctrl Pts',(-1.49051796169812,16.5198135565978,7.));
#10958=CARTESIAN_POINT('Ctrl Pts',(-1.49051796169812,16.5198135565978,-1.4));
#10959=CARTESIAN_POINT('Ctrl Pts',(-1.52918899676864,16.6138949491149,7.));
#10960=CARTESIAN_POINT('Ctrl Pts',(-1.52918899676864,16.6138949491149,-1.4));
#10961=CARTESIAN_POINT('Ctrl Pts',(-1.55162638755018,16.6896454316359,7.));
#10962=CARTESIAN_POINT('Ctrl Pts',(-1.55162638755018,16.6896454316359,-1.4));
#10963=CARTESIAN_POINT('Ctrl Pts',(-1.5648959405722,16.7455711436431,7.));
#10964=CARTESIAN_POINT('Ctrl Pts',(-1.5648959405722,16.7455711436431,-1.4));
#10965=CARTESIAN_POINT('Ctrl Pts',(-1.57225556404314,16.7804505865492,7.));
#10966=CARTESIAN_POINT('Ctrl Pts',(-1.57225556404314,16.7804505865492,-1.4));
#10967=CARTESIAN_POINT('Ctrl Pts',(-1.57930034717564,16.8195656763126,7.));
#10968=CARTESIAN_POINT('Ctrl Pts',(-1.57930034717564,16.8195656763126,-1.4));
#10969=CARTESIAN_POINT('Ctrl Pts',(-1.58971419725806,16.8793055486399,7.));
#10970=CARTESIAN_POINT('Ctrl Pts',(-1.58971419725806,16.8793055486399,-1.4));
#10971=CARTESIAN_POINT('Ctrl Pts',(-1.60803840593146,16.9659973771906,7.));
#10972=CARTESIAN_POINT('Ctrl Pts',(-1.60803840593146,16.9659973771906,-1.4));
#10973=CARTESIAN_POINT('Ctrl Pts',(-1.63700324669262,17.0826338282622,7.));
#10974=CARTESIAN_POINT('Ctrl Pts',(-1.63700324669262,17.0826338282622,-1.4));
#10975=CARTESIAN_POINT('Ctrl Pts',(-1.67639424155265,17.2191007779953,7.));
#10976=CARTESIAN_POINT('Ctrl Pts',(-1.67639424155265,17.2191007779953,-1.4));
#10977=CARTESIAN_POINT('Ctrl Pts',(-1.72763282051122,17.3747717371572,7.));
#10978=CARTESIAN_POINT('Ctrl Pts',(-1.72763282051122,17.3747717371572,-1.4));
#10979=CARTESIAN_POINT('Ctrl Pts',(-1.7922273041827,17.548917731071,7.));
#10980=CARTESIAN_POINT('Ctrl Pts',(-1.7922273041827,17.548917731071,-1.4));
#10981=CARTESIAN_POINT('Ctrl Pts',(-1.87160676754278,17.7407325407201,7.));
#10982=CARTESIAN_POINT('Ctrl Pts',(-1.87160676754278,17.7407325407201,-1.4));
#10983=CARTESIAN_POINT('Ctrl Pts',(-1.96717098182926,17.949326772361,7.));
#10984=CARTESIAN_POINT('Ctrl Pts',(-1.96717098182926,17.949326772361,-1.4));
#10985=CARTESIAN_POINT('Ctrl Pts',(-2.08026807216973,18.1737325312257,7.));
#10986=CARTESIAN_POINT('Ctrl Pts',(-2.08026807216973,18.1737325312257,-1.4));
#10987=CARTESIAN_POINT('Ctrl Pts',(-2.24653249449211,18.4751451900744,7.));
#10988=CARTESIAN_POINT('Ctrl Pts',(-2.24653249449211,18.4751451900744,-1.4));
#10989=CARTESIAN_POINT('Ctrl Pts',(-2.38389175781394,18.6965496529788,7.));
#10990=CARTESIAN_POINT('Ctrl Pts',(-2.38389175781394,18.6965496529788,-1.4));
#10991=CARTESIAN_POINT('Ctrl Pts',(-2.47738131311187,18.8377966288376,7.));
#10992=CARTESIAN_POINT('Ctrl Pts',(-2.47738131311187,18.8377966288376,-1.4));
#10993=CARTESIAN_POINT('',(-2.47738131311187,18.8377966288376,7.));
#10994=CARTESIAN_POINT('Origin',(-1.73472347597681E-15,0.,7.));
#10995=CARTESIAN_POINT('',(-3.46506965370679,18.6813621637974,7.));
#10996=CARTESIAN_POINT('Ctrl Pts',(-3.46506965370701,18.6813621637974,7.));
#10997=CARTESIAN_POINT('Ctrl Pts',(-3.46506965370701,18.6813621637974,-1.39999999999999));
#10998=CARTESIAN_POINT('Ctrl Pts',(-3.51033578853418,18.5181384456162,7.));
#10999=CARTESIAN_POINT('Ctrl Pts',(-3.51033578853418,18.5181384456162,-1.39999999999999));
#11000=CARTESIAN_POINT('Ctrl Pts',(-3.57255446932203,18.265123941733,7.));
#11001=CARTESIAN_POINT('Ctrl Pts',(-3.57255446932203,18.265123941733,-1.39999999999999));
#11002=CARTESIAN_POINT('Ctrl Pts',(-3.63753969769577,17.9270849363835,7.));
#11003=CARTESIAN_POINT('Ctrl Pts',(-3.63753969769577,17.9270849363835,-1.39999999999999));
#11004=CARTESIAN_POINT('Ctrl Pts',(-3.67575622931332,17.6787134541915,7.));
#11005=CARTESIAN_POINT('Ctrl Pts',(-3.67575622931332,17.6787134541915,-1.39999999999999));
#11006=CARTESIAN_POINT('Ctrl Pts',(-3.70218403552948,17.4507975846592,7.));
#11007=CARTESIAN_POINT('Ctrl Pts',(-3.70218403552948,17.4507975846592,-1.39999999999999));
#11008=CARTESIAN_POINT('Ctrl Pts',(-3.7184043554637,17.2438412568379,7.));
#11009=CARTESIAN_POINT('Ctrl Pts',(-3.7184043554637,17.2438412568379,-1.39999999999999));
#11010=CARTESIAN_POINT('Ctrl Pts',(-3.72602328845454,17.0582577813421,7.));
#11011=CARTESIAN_POINT('Ctrl Pts',(-3.72602328845454,17.0582577813421,-1.39999999999999));
#11012=CARTESIAN_POINT('Ctrl Pts',(-3.72664910094709,16.8943723095674,7.));
#11013=CARTESIAN_POINT('Ctrl Pts',(-3.72664910094709,16.8943723095674,-1.39999999999999));
#11014=CARTESIAN_POINT('Ctrl Pts',(-3.72194155665401,16.7524120409277,7.));
#11015=CARTESIAN_POINT('Ctrl Pts',(-3.72194155665401,16.7524120409277,-1.39999999999999));
#11016=CARTESIAN_POINT('Ctrl Pts',(-3.71344611165868,16.632533556064,7.));
#11017=CARTESIAN_POINT('Ctrl Pts',(-3.71344611165868,16.632533556064,-1.39999999999999));
#11018=CARTESIAN_POINT('Ctrl Pts',(-3.70408422142788,16.5444222357228,7.));
#11019=CARTESIAN_POINT('Ctrl Pts',(-3.70408422142788,16.5444222357228,-1.39999999999999));
#11020=CARTESIAN_POINT('Ctrl Pts',(-3.69552774561753,16.4843881842109,7.));
#11021=CARTESIAN_POINT('Ctrl Pts',(-3.69552774561753,16.4843881842109,-1.39999999999999));
#11022=CARTESIAN_POINT('Ctrl Pts',(-3.69014050504823,16.4450105654964,7.));
#11023=CARTESIAN_POINT('Ctrl Pts',(-3.69014050504823,16.4450105654964,-1.39999999999999));
#11024=CARTESIAN_POINT('Ctrl Pts',(-3.68636158229542,16.409563995311,7.));
#11025=CARTESIAN_POINT('Ctrl Pts',(-3.68636158229542,16.409563995311,-1.39999999999999));
#11026=CARTESIAN_POINT('Ctrl Pts',(-3.68169968173256,16.3522749650865,7.));
#11027=CARTESIAN_POINT('Ctrl Pts',(-3.68169968173256,16.3522749650865,-1.39999999999999));
#11028=CARTESIAN_POINT('Ctrl Pts',(-3.67963072201293,16.2732984400115,7.));
#11029=CARTESIAN_POINT('Ctrl Pts',(-3.67963072201293,16.2732984400115,-1.39999999999999));
#11030=CARTESIAN_POINT('Ctrl Pts',(-3.68733631276638,16.1718717115691,7.));
#11031=CARTESIAN_POINT('Ctrl Pts',(-3.68733631276638,16.1718717115691,-1.39999999999999));
#11032=CARTESIAN_POINT('Ctrl Pts',(-3.70904952755066,16.0682204478862,7.));
#11033=CARTESIAN_POINT('Ctrl Pts',(-3.70904952755066,16.0682204478862,-1.39999999999999));
#11034=CARTESIAN_POINT('Ctrl Pts',(-3.75315043649994,15.958574817721,7.));
#11035=CARTESIAN_POINT('Ctrl Pts',(-3.75315043649994,15.958574817721,-1.39999999999999));
#11036=CARTESIAN_POINT('Ctrl Pts',(-3.84407131175633,15.8322454089585,7.));
#11037=CARTESIAN_POINT('Ctrl Pts',(-3.84407131175633,15.8322454089585,-1.39999999999999));
#11038=CARTESIAN_POINT('Ctrl Pts',(-3.94611544431016,15.7691023294921,7.));
#11039=CARTESIAN_POINT('Ctrl Pts',(-3.94611544431016,15.7691023294921,-1.39999999999999));
#11040=CARTESIAN_POINT('Ctrl Pts',(-4.01273932064518,15.7467591314705,7.));
#11041=CARTESIAN_POINT('Ctrl Pts',(-4.01273932064518,15.7467591314705,-1.39999999999999));
#11042=CARTESIAN_POINT('',(-4.01273932064518,15.7467591314705,7.));
#11043=CARTESIAN_POINT('Origin',(0.,0.,7.));
#11044=CARTESIAN_POINT('',(-6.00933848448141,15.0980247376579,7.));
#11045=CARTESIAN_POINT('Ctrl Pts',(-6.00933848448163,15.0980247376578,7.));
#11046=CARTESIAN_POINT('Ctrl Pts',(-6.00933848448163,15.0980247376578,-1.4));
#11047=CARTESIAN_POINT('Ctrl Pts',(-6.076371334954,15.0769402326058,7.));
#11048=CARTESIAN_POINT('Ctrl Pts',(-6.076371334954,15.0769402326058,-1.4));
#11049=CARTESIAN_POINT('Ctrl Pts',(-6.19604134326094,15.0680440207731,7.));
#11050=CARTESIAN_POINT('Ctrl Pts',(-6.19604134326094,15.0680440207731,-1.4));
#11051=CARTESIAN_POINT('Ctrl Pts',(-6.34385243988825,15.1168047097501,7.));
#11052=CARTESIAN_POINT('Ctrl Pts',(-6.34385243988825,15.1168047097501,-1.4));
#11053=CARTESIAN_POINT('Ctrl Pts',(-6.44397890908501,15.1795880240196,7.));
#11054=CARTESIAN_POINT('Ctrl Pts',(-6.44397890908501,15.1795880240196,-1.4));
#11055=CARTESIAN_POINT('Ctrl Pts',(-6.52246995302233,15.2506809503975,7.));
#11056=CARTESIAN_POINT('Ctrl Pts',(-6.52246995302233,15.2506809503975,-1.4));
#11057=CARTESIAN_POINT('Ctrl Pts',(-6.58832104206028,15.3282076647862,7.));
#11058=CARTESIAN_POINT('Ctrl Pts',(-6.58832104206028,15.3282076647862,-1.4));
#11059=CARTESIAN_POINT('Ctrl Pts',(-6.63306845520281,15.3933171197393,7.));
#11060=CARTESIAN_POINT('Ctrl Pts',(-6.63306845520281,15.3933171197393,-1.4));
#11061=CARTESIAN_POINT('Ctrl Pts',(-6.66297054550547,15.4424051151807,7.));
#11062=CARTESIAN_POINT('Ctrl Pts',(-6.66297054550547,15.4424051151807,-1.4));
#11063=CARTESIAN_POINT('Ctrl Pts',(-6.68074830397731,15.4733031879166,7.));
#11064=CARTESIAN_POINT('Ctrl Pts',(-6.68074830397731,15.4733031879166,-1.4));
#11065=CARTESIAN_POINT('Ctrl Pts',(-6.69953551835474,15.5083268912119,7.));
#11066=CARTESIAN_POINT('Ctrl Pts',(-6.69953551835474,15.5083268912119,-1.4));
#11067=CARTESIAN_POINT('Ctrl Pts',(-6.72790031412628,15.5619248294191,7.));
#11068=CARTESIAN_POINT('Ctrl Pts',(-6.72790031412628,15.5619248294191,-1.4));
#11069=CARTESIAN_POINT('Ctrl Pts',(-6.77211692048667,15.6387111659832,7.));
#11070=CARTESIAN_POINT('Ctrl Pts',(-6.77211692048667,15.6387111659832,-1.4));
#11071=CARTESIAN_POINT('Ctrl Pts',(-6.83570676658072,15.7406883947778,7.));
#11072=CARTESIAN_POINT('Ctrl Pts',(-6.83570676658072,15.7406883947778,-1.4));
#11073=CARTESIAN_POINT('Ctrl Pts',(-6.91534043556374,15.8583036897433,7.));
#11074=CARTESIAN_POINT('Ctrl Pts',(-6.91534043556374,15.8583036897433,-1.4));
#11075=CARTESIAN_POINT('Ctrl Pts',(-7.01217619187967,15.9905219781863,7.));
#11076=CARTESIAN_POINT('Ctrl Pts',(-7.01217619187967,15.9905219781863,-1.4));
#11077=CARTESIAN_POINT('Ctrl Pts',(-7.12742326811385,16.1361838672874,7.));
#11078=CARTESIAN_POINT('Ctrl Pts',(-7.12742326811385,16.1361838672874,-1.4));
#11079=CARTESIAN_POINT('Ctrl Pts',(-7.26219165995682,16.2940809887434,7.));
#11080=CARTESIAN_POINT('Ctrl Pts',(-7.26219165995682,16.2940809887434,-1.4));
#11081=CARTESIAN_POINT('Ctrl Pts',(-7.41753779118424,16.4629349257385,7.));
#11082=CARTESIAN_POINT('Ctrl Pts',(-7.41753779118424,16.4629349257385,-1.4));
#11083=CARTESIAN_POINT('Ctrl Pts',(-7.59444470905137,16.6414085620714,7.));
#11084=CARTESIAN_POINT('Ctrl Pts',(-7.59444470905137,16.6414085620714,-1.4));
#11085=CARTESIAN_POINT('Ctrl Pts',(-7.8457132052331,16.8766905033058,7.));
#11086=CARTESIAN_POINT('Ctrl Pts',(-7.8457132052331,16.8766905033058,-1.4));
#11087=CARTESIAN_POINT('Ctrl Pts',(-8.04476736935674,17.0448123137865,7.));
#11088=CARTESIAN_POINT('Ctrl Pts',(-8.04476736935674,17.0448123137865,-1.4));
#11089=CARTESIAN_POINT('Ctrl Pts',(-8.1773289360728,17.1502563092004,7.));
#11090=CARTESIAN_POINT('Ctrl Pts',(-8.1773289360728,17.1502563092004,-1.4));
#11091=CARTESIAN_POINT('',(-8.1773289360728,17.1502563092004,7.));
#11092=CARTESIAN_POINT('Origin',(1.73472347597681E-15,0.,7.));
#11093=CARTESIAN_POINT('',(-9.06833546026097,16.6962658094609,7.));
#11094=CARTESIAN_POINT('Ctrl Pts',(-9.06833546026118,16.6962658094608,7.));
#11095=CARTESIAN_POINT('Ctrl Pts',(-9.06833546026118,16.6962658094608,-1.39999999999999));
#11096=CARTESIAN_POINT('Ctrl Pts',(-9.06094720995302,16.5270428237395,7.));
#11097=CARTESIAN_POINT('Ctrl Pts',(-9.06094720995302,16.5270428237395,-1.39999999999999));
#11098=CARTESIAN_POINT('Ctrl Pts',(-9.04193491022831,16.2671851013731,7.));
#11099=CARTESIAN_POINT('Ctrl Pts',(-9.04193491022831,16.2671851013731,-1.39999999999999));
#11100=CARTESIAN_POINT('Ctrl Pts',(-8.9992797377215,15.9256093626227,7.));
#11101=CARTESIAN_POINT('Ctrl Pts',(-8.9992797377215,15.9256093626227,-1.39999999999999));
#11102=CARTESIAN_POINT('Ctrl Pts',(-8.95887481023115,15.6775844882862,7.));
#11103=CARTESIAN_POINT('Ctrl Pts',(-8.95887481023115,15.6775844882862,-1.39999999999999));
#11104=CARTESIAN_POINT('Ctrl Pts',(-8.91357927057119,15.4526569741556,7.));
#11105=CARTESIAN_POINT('Ctrl Pts',(-8.91357927057119,15.4526569741556,-1.39999999999999));
#11106=CARTESIAN_POINT('Ctrl Pts',(-8.8650526891508,15.2508174554788,7.));
#11107=CARTESIAN_POINT('Ctrl Pts',(-8.8650526891508,15.2508174554788,-1.39999999999999));
#11108=CARTESIAN_POINT('Ctrl Pts',(-8.81495027721559,15.0719627020186,7.));
#11109=CARTESIAN_POINT('Ctrl Pts',(-8.81495027721559,15.0719627020186,-1.39999999999999));
#11110=CARTESIAN_POINT('Ctrl Pts',(-8.76490206435507,14.9159049694657,7.));
#11111=CARTESIAN_POINT('Ctrl Pts',(-8.76490206435507,14.9159049694657,-1.39999999999999));
#11112=CARTESIAN_POINT('Ctrl Pts',(-8.71655678814369,14.7823474421093,7.));
#11113=CARTESIAN_POINT('Ctrl Pts',(-8.71655678814369,14.7823474421093,-1.39999999999999));
#11114=CARTESIAN_POINT('Ctrl Pts',(-8.67143265073926,14.6709614647944,7.));
#11115=CARTESIAN_POINT('Ctrl Pts',(-8.67143265073926,14.6709614647944,-1.39999999999999));
#11116=CARTESIAN_POINT('Ctrl Pts',(-8.63530106864816,14.5900556026053,7.));
#11117=CARTESIAN_POINT('Ctrl Pts',(-8.63530106864816,14.5900556026053,-1.39999999999999));
#11118=CARTESIAN_POINT('Ctrl Pts',(-8.60861183441386,14.5356039231527,7.));
#11119=CARTESIAN_POINT('Ctrl Pts',(-8.60861183441386,14.5356039231527,-1.39999999999999));
#11120=CARTESIAN_POINT('Ctrl Pts',(-8.59131991078476,14.4998183311667,7.));
#11121=CARTESIAN_POINT('Ctrl Pts',(-8.59131991078476,14.4998183311667,-1.39999999999999));
#11122=CARTESIAN_POINT('Ctrl Pts',(-8.57677234909655,14.4672743909627,7.));
#11123=CARTESIAN_POINT('Ctrl Pts',(-8.57677234909655,14.4672743909627,-1.39999999999999));
#11124=CARTESIAN_POINT('Ctrl Pts',(-8.55463533425729,14.4142298919554,7.));
#11125=CARTESIAN_POINT('Ctrl Pts',(-8.55463533425729,14.4142298919554,-1.39999999999999));
#11126=CARTESIAN_POINT('Ctrl Pts',(-8.52826254822913,14.3397580968626,7.));
#11127=CARTESIAN_POINT('Ctrl Pts',(-8.52826254822913,14.3397580968626,-1.39999999999999));
#11128=CARTESIAN_POINT('Ctrl Pts',(-8.50424841775454,14.2409143873564,7.));
#11129=CARTESIAN_POINT('Ctrl Pts',(-8.50424841775454,14.2409143873564,-1.39999999999999));
#11130=CARTESIAN_POINT('Ctrl Pts',(-8.49286891019839,14.1356264252377,7.));
#11131=CARTESIAN_POINT('Ctrl Pts',(-8.49286891019839,14.1356264252377,-1.39999999999999));
#11132=CARTESIAN_POINT('Ctrl Pts',(-8.50092900394916,14.0177193038531,7.));
#11133=CARTESIAN_POINT('Ctrl Pts',(-8.50092900394916,14.0177193038531,-1.39999999999999));
#11134=CARTESIAN_POINT('Ctrl Pts',(-8.54836196063204,13.8694768008521,7.));
#11135=CARTESIAN_POINT('Ctrl Pts',(-8.54836196063204,13.8694768008521,-1.39999999999999));
#11136=CARTESIAN_POINT('Ctrl Pts',(-8.62589941321477,13.7778907925313,7.));
#11137=CARTESIAN_POINT('Ctrl Pts',(-8.62589941321477,13.7778907925313,-1.39999999999999));
#11138=CARTESIAN_POINT('Ctrl Pts',(-8.68235805704666,13.7360532384392,7.));
#11139=CARTESIAN_POINT('Ctrl Pts',(-8.68235805704666,13.7360532384392,-1.39999999999999));
#11140=CARTESIAN_POINT('',(-8.68235805704666,13.7360532384392,7.));
#11141=CARTESIAN_POINT('Origin',(0.,0.,7.));
#11142=CARTESIAN_POINT('',(-10.380766749719,12.5020870932788,7.));
#11143=CARTESIAN_POINT('Ctrl Pts',(-10.3807667497191,12.5020870932787,7.));
#11144=CARTESIAN_POINT('Ctrl Pts',(-10.3807667497191,12.5020870932787,-1.4));
#11145=CARTESIAN_POINT('Ctrl Pts',(-10.4380033085876,12.4613202473787,7.));
#11146=CARTESIAN_POINT('Ctrl Pts',(-10.4380033085876,12.4613202473787,-1.4));
#11147=CARTESIAN_POINT('Ctrl Pts',(-10.5490671691512,12.4158793808611,7.));
#11148=CARTESIAN_POINT('Ctrl Pts',(-10.5490671691512,12.4158793808611,-1.4));
#11149=CARTESIAN_POINT('Ctrl Pts',(-10.7047117573307,12.4165774110367,7.));
#11150=CARTESIAN_POINT('Ctrl Pts',(-10.7047117573307,12.4165774110367,-1.4));
#11151=CARTESIAN_POINT('Ctrl Pts',(-10.8193387993863,12.4453471106187,7.));
#11152=CARTESIAN_POINT('Ctrl Pts',(-10.8193387993863,12.4453471106187,-1.4));
#11153=CARTESIAN_POINT('Ctrl Pts',(-10.9159571406243,12.48870543503,7.));
#11154=CARTESIAN_POINT('Ctrl Pts',(-10.9159571406243,12.48870543503,-1.4));
#11155=CARTESIAN_POINT('Ctrl Pts',(-11.0025423202232,12.5420886163255,7.));
#11156=CARTESIAN_POINT('Ctrl Pts',(-11.0025423202232,12.5420886163255,-1.4));
#11157=CARTESIAN_POINT('Ctrl Pts',(-11.0652195671547,12.5901836766158,7.));
#11158=CARTESIAN_POINT('Ctrl Pts',(-11.0652195671547,12.5901836766158,-1.4));
#11159=CARTESIAN_POINT('Ctrl Pts',(-11.1088271697991,12.6276288804813,7.));
#11160=CARTESIAN_POINT('Ctrl Pts',(-11.1088271697991,12.6276288804813,-1.4));
#11161=CARTESIAN_POINT('Ctrl Pts',(-11.1352828524077,12.651521064408,7.));
#11162=CARTESIAN_POINT('Ctrl Pts',(-11.1352828524077,12.651521064408,-1.4));
#11163=CARTESIAN_POINT('Ctrl Pts',(-11.1639734745886,12.6790250171322,7.));
#11164=CARTESIAN_POINT('Ctrl Pts',(-11.1639734745886,12.6790250171322,-1.4));
#11165=CARTESIAN_POINT('Ctrl Pts',(-11.20751267221,12.7212344815888,7.));
#11166=CARTESIAN_POINT('Ctrl Pts',(-11.20751267221,12.7212344815888,-1.4));
#11167=CARTESIAN_POINT('Ctrl Pts',(-11.2732934467516,12.7805989445416,7.));
#11168=CARTESIAN_POINT('Ctrl Pts',(-11.2732934467516,12.7805989445416,-1.4));
#11169=CARTESIAN_POINT('Ctrl Pts',(-11.3652836809863,12.8579347093876,7.));
#11170=CARTESIAN_POINT('Ctrl Pts',(-11.3652836809863,12.8579347093876,-1.4));
#11171=CARTESIAN_POINT('Ctrl Pts',(-11.4773649257319,12.9451853450404,7.));
#11172=CARTESIAN_POINT('Ctrl Pts',(-11.4773649257319,12.9451853450404,-1.4));
#11173=CARTESIAN_POINT('Ctrl Pts',(-11.6103189008826,13.0410085154727,7.));
#11174=CARTESIAN_POINT('Ctrl Pts',(-11.6103189008826,13.0410085154727,-1.4));
#11175=CARTESIAN_POINT('Ctrl Pts',(-11.764937382884,13.1439278991698,7.));
#11176=CARTESIAN_POINT('Ctrl Pts',(-11.764937382884,13.1439278991698,-1.4));
#11177=CARTESIAN_POINT('Ctrl Pts',(-11.9419026340297,13.2524512620507,7.));
#11178=CARTESIAN_POINT('Ctrl Pts',(-11.9419026340297,13.2524512620507,-1.4));
#11179=CARTESIAN_POINT('Ctrl Pts',(-12.1418243205134,13.3650363045724,7.));
#11180=CARTESIAN_POINT('Ctrl Pts',(-12.1418243205134,13.3650363045724,-1.4));
#11181=CARTESIAN_POINT('Ctrl Pts',(-12.3652241842034,13.4801075753502,7.));
#11182=CARTESIAN_POINT('Ctrl Pts',(-12.3652241842034,13.4801075753502,-1.4));
#11183=CARTESIAN_POINT('Ctrl Pts',(-12.6769008431476,13.6262277632565,7.));
#11184=CARTESIAN_POINT('Ctrl Pts',(-12.6769008431476,13.6262277632565,-1.4));
#11185=CARTESIAN_POINT('Ctrl Pts',(-12.9181650995968,13.7246099871303,7.));
#11186=CARTESIAN_POINT('Ctrl Pts',(-12.9181650995968,13.7246099871303,-1.4));
#11187=CARTESIAN_POINT('Ctrl Pts',(-13.07682262797,13.7839294091566,7.));
#11188=CARTESIAN_POINT('Ctrl Pts',(-13.07682262797,13.7839294091566,-1.4));
#11189=CARTESIAN_POINT('',(-13.07682262797,13.7839294091566,7.));
#11190=CARTESIAN_POINT('Origin',(1.57723797680727E-16,0.,7.));
#11191=CARTESIAN_POINT('',(-13.7839294091564,13.0768226279702,7.));
#11192=CARTESIAN_POINT('Ctrl Pts',(-13.7839294091566,13.07682262797,7.));
#11193=CARTESIAN_POINT('Ctrl Pts',(-13.7839294091566,13.07682262797,-1.39999999999999));
#11194=CARTESIAN_POINT('Ctrl Pts',(-13.7246099871302,12.9181650995968,7.));
#11195=CARTESIAN_POINT('Ctrl Pts',(-13.7246099871302,12.9181650995968,-1.39999999999999));
#11196=CARTESIAN_POINT('Ctrl Pts',(-13.6262277632565,12.6769008431476,7.));
#11197=CARTESIAN_POINT('Ctrl Pts',(-13.6262277632565,12.6769008431476,-1.39999999999999));
#11198=CARTESIAN_POINT('Ctrl Pts',(-13.4801075753502,12.3652241842034,7.));
#11199=CARTESIAN_POINT('Ctrl Pts',(-13.4801075753502,12.3652241842034,-1.39999999999999));
#11200=CARTESIAN_POINT('Ctrl Pts',(-13.3650363045723,12.1418243205134,7.));
#11201=CARTESIAN_POINT('Ctrl Pts',(-13.3650363045723,12.1418243205134,-1.39999999999999));
#11202=CARTESIAN_POINT('Ctrl Pts',(-13.2524512620508,11.9419026340297,7.));
#11203=CARTESIAN_POINT('Ctrl Pts',(-13.2524512620508,11.9419026340297,-1.39999999999999));
#11204=CARTESIAN_POINT('Ctrl Pts',(-13.1439278991698,11.764937382884,7.));
#11205=CARTESIAN_POINT('Ctrl Pts',(-13.1439278991698,11.764937382884,-1.39999999999999));
#11206=CARTESIAN_POINT('Ctrl Pts',(-13.0410085154728,11.6103189008826,7.));
#11207=CARTESIAN_POINT('Ctrl Pts',(-13.0410085154728,11.6103189008826,-1.39999999999999));
#11208=CARTESIAN_POINT('Ctrl Pts',(-12.9451853450404,11.4773649257318,7.));
#11209=CARTESIAN_POINT('Ctrl Pts',(-12.9451853450404,11.4773649257318,-1.39999999999999));
#11210=CARTESIAN_POINT('Ctrl Pts',(-12.8579347093876,11.3652836809863,7.));
#11211=CARTESIAN_POINT('Ctrl Pts',(-12.8579347093876,11.3652836809863,-1.39999999999999));
#11212=CARTESIAN_POINT('Ctrl Pts',(-12.7805989445416,11.2732934467516,7.));
#11213=CARTESIAN_POINT('Ctrl Pts',(-12.7805989445416,11.2732934467516,-1.39999999999999));
#11214=CARTESIAN_POINT('Ctrl Pts',(-12.7212344815888,11.2075126722099,7.));
#11215=CARTESIAN_POINT('Ctrl Pts',(-12.7212344815888,11.2075126722099,-1.39999999999999));
#11216=CARTESIAN_POINT('Ctrl Pts',(-12.6790250171322,11.1639734745886,7.));
#11217=CARTESIAN_POINT('Ctrl Pts',(-12.6790250171322,11.1639734745886,-1.39999999999999));
#11218=CARTESIAN_POINT('Ctrl Pts',(-12.651521064408,11.1352828524077,7.));
#11219=CARTESIAN_POINT('Ctrl Pts',(-12.651521064408,11.1352828524077,-1.39999999999999));
#11220=CARTESIAN_POINT('Ctrl Pts',(-12.6276288804813,11.1088271697991,7.));
#11221=CARTESIAN_POINT('Ctrl Pts',(-12.6276288804813,11.1088271697991,-1.39999999999999));
#11222=CARTESIAN_POINT('Ctrl Pts',(-12.5901836766158,11.0652195671547,7.));
#11223=CARTESIAN_POINT('Ctrl Pts',(-12.5901836766158,11.0652195671547,-1.39999999999999));
#11224=CARTESIAN_POINT('Ctrl Pts',(-12.5420886163255,11.0025423202231,7.));
#11225=CARTESIAN_POINT('Ctrl Pts',(-12.5420886163255,11.0025423202231,-1.39999999999999));
#11226=CARTESIAN_POINT('Ctrl Pts',(-12.48870543503,10.9159571406243,7.));
#11227=CARTESIAN_POINT('Ctrl Pts',(-12.48870543503,10.9159571406243,-1.39999999999999));
#11228=CARTESIAN_POINT('Ctrl Pts',(-12.4453471106187,10.8193387993863,7.));
#11229=CARTESIAN_POINT('Ctrl Pts',(-12.4453471106187,10.8193387993863,-1.39999999999999));
#11230=CARTESIAN_POINT('Ctrl Pts',(-12.4165774110367,10.7047117573307,7.));
#11231=CARTESIAN_POINT('Ctrl Pts',(-12.4165774110367,10.7047117573307,-1.39999999999999));
#11232=CARTESIAN_POINT('Ctrl Pts',(-12.4158793808611,10.5490671691512,7.));
#11233=CARTESIAN_POINT('Ctrl Pts',(-12.4158793808611,10.5490671691512,-1.39999999999999));
#11234=CARTESIAN_POINT('Ctrl Pts',(-12.4613202473787,10.4380033085876,7.));
#11235=CARTESIAN_POINT('Ctrl Pts',(-12.4613202473787,10.4380033085876,-1.39999999999999));
#11236=CARTESIAN_POINT('Ctrl Pts',(-12.5020870932787,10.3807667497191,7.));
#11237=CARTESIAN_POINT('Ctrl Pts',(-12.5020870932787,10.3807667497191,-1.39999999999999));
#11238=CARTESIAN_POINT('',(-12.5020870932787,10.3807667497191,7.));
#11239=CARTESIAN_POINT('Origin',(0.,0.,7.));
#11240=CARTESIAN_POINT('',(-13.7360532384391,8.68235805704682,7.));
#11241=CARTESIAN_POINT('Ctrl Pts',(-13.7360532384392,8.68235805704666,7.));
#11242=CARTESIAN_POINT('Ctrl Pts',(-13.7360532384392,8.68235805704666,-1.4));
#11243=CARTESIAN_POINT('Ctrl Pts',(-13.7778907925313,8.62589941321479,7.));
#11244=CARTESIAN_POINT('Ctrl Pts',(-13.7778907925313,8.62589941321479,-1.4));
#11245=CARTESIAN_POINT('Ctrl Pts',(-13.8694768008521,8.54836196063206,7.));
#11246=CARTESIAN_POINT('Ctrl Pts',(-13.8694768008521,8.54836196063206,-1.4));
#11247=CARTESIAN_POINT('Ctrl Pts',(-14.0177193038531,8.50092900394919,7.));
#11248=CARTESIAN_POINT('Ctrl Pts',(-14.0177193038531,8.50092900394919,-1.4));
#11249=CARTESIAN_POINT('Ctrl Pts',(-14.1356264252377,8.49286891019842,7.));
#11250=CARTESIAN_POINT('Ctrl Pts',(-14.1356264252377,8.49286891019842,-1.4));
#11251=CARTESIAN_POINT('Ctrl Pts',(-14.2409143873564,8.50424841775455,7.));
#11252=CARTESIAN_POINT('Ctrl Pts',(-14.2409143873564,8.50424841775455,-1.4));
#11253=CARTESIAN_POINT('Ctrl Pts',(-14.3397580968626,8.52826254822914,7.));
#11254=CARTESIAN_POINT('Ctrl Pts',(-14.3397580968626,8.52826254822914,-1.4));
#11255=CARTESIAN_POINT('Ctrl Pts',(-14.4142298919555,8.55463533425731,7.));
#11256=CARTESIAN_POINT('Ctrl Pts',(-14.4142298919555,8.55463533425731,-1.4));
#11257=CARTESIAN_POINT('Ctrl Pts',(-14.4672743909627,8.57677234909655,7.));
#11258=CARTESIAN_POINT('Ctrl Pts',(-14.4672743909627,8.57677234909655,-1.4));
#11259=CARTESIAN_POINT('Ctrl Pts',(-14.4998183311667,8.59131991078475,7.));
#11260=CARTESIAN_POINT('Ctrl Pts',(-14.4998183311667,8.59131991078475,-1.4));
#11261=CARTESIAN_POINT('Ctrl Pts',(-14.5356039231527,8.60861183441388,7.));
#11262=CARTESIAN_POINT('Ctrl Pts',(-14.5356039231527,8.60861183441388,-1.4));
#11263=CARTESIAN_POINT('Ctrl Pts',(-14.5900556026053,8.63530106864817,7.));
#11264=CARTESIAN_POINT('Ctrl Pts',(-14.5900556026053,8.63530106864817,-1.4));
#11265=CARTESIAN_POINT('Ctrl Pts',(-14.6709614647944,8.67143265073926,7.));
#11266=CARTESIAN_POINT('Ctrl Pts',(-14.6709614647944,8.67143265073926,-1.4));
#11267=CARTESIAN_POINT('Ctrl Pts',(-14.7823474421093,8.71655678814371,7.));
#11268=CARTESIAN_POINT('Ctrl Pts',(-14.7823474421093,8.71655678814371,-1.4));
#11269=CARTESIAN_POINT('Ctrl Pts',(-14.9159049694657,8.76490206435508,7.));
#11270=CARTESIAN_POINT('Ctrl Pts',(-14.9159049694657,8.76490206435508,-1.4));
#11271=CARTESIAN_POINT('Ctrl Pts',(-15.0719627020186,8.81495027721556,7.));
#11272=CARTESIAN_POINT('Ctrl Pts',(-15.0719627020186,8.81495027721556,-1.4));
#11273=CARTESIAN_POINT('Ctrl Pts',(-15.2508174554788,8.86505268915083,7.));
#11274=CARTESIAN_POINT('Ctrl Pts',(-15.2508174554788,8.86505268915083,-1.4));
#11275=CARTESIAN_POINT('Ctrl Pts',(-15.4526569741556,8.91357927057117,7.));
#11276=CARTESIAN_POINT('Ctrl Pts',(-15.4526569741556,8.91357927057117,-1.4));
#11277=CARTESIAN_POINT('Ctrl Pts',(-15.6775844882863,8.95887481023116,7.));
#11278=CARTESIAN_POINT('Ctrl Pts',(-15.6775844882863,8.95887481023116,-1.4));
#11279=CARTESIAN_POINT('Ctrl Pts',(-15.9256093626227,8.99927973772153,7.));
#11280=CARTESIAN_POINT('Ctrl Pts',(-15.9256093626227,8.99927973772153,-1.4));
#11281=CARTESIAN_POINT('Ctrl Pts',(-16.2671851013731,9.04193491022832,7.));
#11282=CARTESIAN_POINT('Ctrl Pts',(-16.2671851013731,9.04193491022832,-1.4));
#11283=CARTESIAN_POINT('Ctrl Pts',(-16.5270428237395,9.06094720995306,7.));
#11284=CARTESIAN_POINT('Ctrl Pts',(-16.5270428237395,9.06094720995306,-1.4));
#11285=CARTESIAN_POINT('Ctrl Pts',(-16.6962658094608,9.06833546026117,7.));
#11286=CARTESIAN_POINT('Ctrl Pts',(-16.6962658094608,9.06833546026117,-1.4));
#11287=CARTESIAN_POINT('',(-16.6962658094608,9.06833546026117,7.));
#11288=CARTESIAN_POINT('Origin',(-1.73472347597681E-15,0.,7.));
#11289=CARTESIAN_POINT('',(-17.1502563092003,8.17732893607296,7.));
#11290=CARTESIAN_POINT('Ctrl Pts',(-17.1502563092004,8.17732893607281,7.));
#11291=CARTESIAN_POINT('Ctrl Pts',(-17.1502563092004,8.17732893607281,-1.39999999999999));
#11292=CARTESIAN_POINT('Ctrl Pts',(-17.0448123137865,8.04476736935675,7.));
#11293=CARTESIAN_POINT('Ctrl Pts',(-17.0448123137865,8.04476736935675,-1.39999999999999));
#11294=CARTESIAN_POINT('Ctrl Pts',(-16.8766905033057,7.8457132052331,7.));
#11295=CARTESIAN_POINT('Ctrl Pts',(-16.8766905033057,7.8457132052331,-1.39999999999999));
#11296=CARTESIAN_POINT('Ctrl Pts',(-16.6414085620714,7.59444470905138,7.));
#11297=CARTESIAN_POINT('Ctrl Pts',(-16.6414085620714,7.59444470905138,-1.39999999999999));
#11298=CARTESIAN_POINT('Ctrl Pts',(-16.4629349257385,7.41753779118423,7.));
#11299=CARTESIAN_POINT('Ctrl Pts',(-16.4629349257385,7.41753779118423,-1.39999999999999));
#11300=CARTESIAN_POINT('Ctrl Pts',(-16.2940809887434,7.26219165995682,7.));
#11301=CARTESIAN_POINT('Ctrl Pts',(-16.2940809887434,7.26219165995682,-1.39999999999999));
#11302=CARTESIAN_POINT('Ctrl Pts',(-16.1361838672874,7.12742326811386,7.));
#11303=CARTESIAN_POINT('Ctrl Pts',(-16.1361838672874,7.12742326811386,-1.39999999999999));
#11304=CARTESIAN_POINT('Ctrl Pts',(-15.9905219781863,7.01217619187965,7.));
#11305=CARTESIAN_POINT('Ctrl Pts',(-15.9905219781863,7.01217619187965,-1.39999999999999));
#11306=CARTESIAN_POINT('Ctrl Pts',(-15.8583036897432,6.91534043556372,7.));
#11307=CARTESIAN_POINT('Ctrl Pts',(-15.8583036897432,6.91534043556372,-1.39999999999999));
#11308=CARTESIAN_POINT('Ctrl Pts',(-15.7406883947777,6.83570676658073,7.));
#11309=CARTESIAN_POINT('Ctrl Pts',(-15.7406883947777,6.83570676658073,-1.39999999999999));
#11310=CARTESIAN_POINT('Ctrl Pts',(-15.6387111659832,6.77211692048666,7.));
#11311=CARTESIAN_POINT('Ctrl Pts',(-15.6387111659832,6.77211692048666,-1.39999999999999));
#11312=CARTESIAN_POINT('Ctrl Pts',(-15.5619248294191,6.72790031412627,7.));
#11313=CARTESIAN_POINT('Ctrl Pts',(-15.5619248294191,6.72790031412627,-1.39999999999999));
#11314=CARTESIAN_POINT('Ctrl Pts',(-15.5083268912118,6.69953551835476,7.));
#11315=CARTESIAN_POINT('Ctrl Pts',(-15.5083268912118,6.69953551835476,-1.39999999999999));
#11316=CARTESIAN_POINT('Ctrl Pts',(-15.4733031879166,6.68074830397729,7.));
#11317=CARTESIAN_POINT('Ctrl Pts',(-15.4733031879166,6.68074830397729,-1.39999999999999));
#11318=CARTESIAN_POINT('Ctrl Pts',(-15.4424051151807,6.66297054550545,7.));
#11319=CARTESIAN_POINT('Ctrl Pts',(-15.4424051151807,6.66297054550545,-1.39999999999999));
#11320=CARTESIAN_POINT('Ctrl Pts',(-15.3933171197393,6.6330684552028,7.));
#11321=CARTESIAN_POINT('Ctrl Pts',(-15.3933171197393,6.6330684552028,-1.39999999999999));
#11322=CARTESIAN_POINT('Ctrl Pts',(-15.3282076647861,6.58832104206026,7.));
#11323=CARTESIAN_POINT('Ctrl Pts',(-15.3282076647861,6.58832104206026,-1.39999999999999));
#11324=CARTESIAN_POINT('Ctrl Pts',(-15.2506809503975,6.5224699530223,7.));
#11325=CARTESIAN_POINT('Ctrl Pts',(-15.2506809503975,6.5224699530223,-1.39999999999999));
#11326=CARTESIAN_POINT('Ctrl Pts',(-15.1795880240196,6.443978909085,7.));
#11327=CARTESIAN_POINT('Ctrl Pts',(-15.1795880240196,6.443978909085,-1.39999999999999));
#11328=CARTESIAN_POINT('Ctrl Pts',(-15.1168047097501,6.34385243988827,7.));
#11329=CARTESIAN_POINT('Ctrl Pts',(-15.1168047097501,6.34385243988827,-1.39999999999999));
#11330=CARTESIAN_POINT('Ctrl Pts',(-15.0680440207731,6.19604134326095,7.));
#11331=CARTESIAN_POINT('Ctrl Pts',(-15.0680440207731,6.19604134326095,-1.39999999999999));
#11332=CARTESIAN_POINT('Ctrl Pts',(-15.0769402326058,6.07637133495398,7.));
#11333=CARTESIAN_POINT('Ctrl Pts',(-15.0769402326058,6.07637133495398,-1.39999999999999));
#11334=CARTESIAN_POINT('Ctrl Pts',(-15.0980247376578,6.00933848448163,7.));
#11335=CARTESIAN_POINT('Ctrl Pts',(-15.0980247376578,6.00933848448163,-1.39999999999999));
#11336=CARTESIAN_POINT('',(-15.0980247376578,6.00933848448163,7.));
#11337=CARTESIAN_POINT('Origin',(0.,0.,7.));
#11338=CARTESIAN_POINT('',(-15.7467591314704,4.01273932064536,7.));
#11339=CARTESIAN_POINT('Ctrl Pts',(-15.7467591314704,4.0127393206452,7.));
#11340=CARTESIAN_POINT('Ctrl Pts',(-15.7467591314704,4.0127393206452,-1.4));
#11341=CARTESIAN_POINT('Ctrl Pts',(-15.7691023294921,3.94611544431018,7.));
#11342=CARTESIAN_POINT('Ctrl Pts',(-15.7691023294921,3.94611544431018,-1.4));
#11343=CARTESIAN_POINT('Ctrl Pts',(-15.8322454089585,3.84407131175636,7.));
#11344=CARTESIAN_POINT('Ctrl Pts',(-15.8322454089585,3.84407131175636,-1.4));
#11345=CARTESIAN_POINT('Ctrl Pts',(-15.958574817721,3.75315043649999,7.));
#11346=CARTESIAN_POINT('Ctrl Pts',(-15.958574817721,3.75315043649999,-1.4));
#11347=CARTESIAN_POINT('Ctrl Pts',(-16.0682204478862,3.7090495275507,7.));
#11348=CARTESIAN_POINT('Ctrl Pts',(-16.0682204478862,3.7090495275507,-1.4));
#11349=CARTESIAN_POINT('Ctrl Pts',(-16.1718717115691,3.68733631276638,7.));
#11350=CARTESIAN_POINT('Ctrl Pts',(-16.1718717115691,3.68733631276638,-1.4));
#11351=CARTESIAN_POINT('Ctrl Pts',(-16.2732984400115,3.67963072201295,7.));
#11352=CARTESIAN_POINT('Ctrl Pts',(-16.2732984400115,3.67963072201295,-1.4));
#11353=CARTESIAN_POINT('Ctrl Pts',(-16.3522749650865,3.68169968173258,7.));
#11354=CARTESIAN_POINT('Ctrl Pts',(-16.3522749650865,3.68169968173258,-1.4));
#11355=CARTESIAN_POINT('Ctrl Pts',(-16.409563995311,3.68636158229543,7.));
#11356=CARTESIAN_POINT('Ctrl Pts',(-16.409563995311,3.68636158229543,-1.4));
#11357=CARTESIAN_POINT('Ctrl Pts',(-16.4450105654964,3.69014050504823,7.));
#11358=CARTESIAN_POINT('Ctrl Pts',(-16.4450105654964,3.69014050504823,-1.4));
#11359=CARTESIAN_POINT('Ctrl Pts',(-16.4843881842109,3.69552774561757,7.));
#11360=CARTESIAN_POINT('Ctrl Pts',(-16.4843881842109,3.69552774561757,-1.4));
#11361=CARTESIAN_POINT('Ctrl Pts',(-16.5444222357228,3.70408422142789,7.));
#11362=CARTESIAN_POINT('Ctrl Pts',(-16.5444222357228,3.70408422142789,-1.4));
#11363=CARTESIAN_POINT('Ctrl Pts',(-16.632533556064,3.7134461116587,7.));
#11364=CARTESIAN_POINT('Ctrl Pts',(-16.632533556064,3.7134461116587,-1.4));
#11365=CARTESIAN_POINT('Ctrl Pts',(-16.7524120409277,3.72194155665404,7.));
#11366=CARTESIAN_POINT('Ctrl Pts',(-16.7524120409277,3.72194155665404,-1.4));
#11367=CARTESIAN_POINT('Ctrl Pts',(-16.8943723095674,3.72664910094711,7.));
#11368=CARTESIAN_POINT('Ctrl Pts',(-16.8943723095674,3.72664910094711,-1.4));
#11369=CARTESIAN_POINT('Ctrl Pts',(-17.0582577813421,3.72602328845453,7.));
#11370=CARTESIAN_POINT('Ctrl Pts',(-17.0582577813421,3.72602328845453,-1.4));
#11371=CARTESIAN_POINT('Ctrl Pts',(-17.2438412568379,3.71840435546374,7.));
#11372=CARTESIAN_POINT('Ctrl Pts',(-17.2438412568379,3.71840435546374,-1.4));
#11373=CARTESIAN_POINT('Ctrl Pts',(-17.4507975846592,3.70218403552947,7.));
#11374=CARTESIAN_POINT('Ctrl Pts',(-17.4507975846592,3.70218403552947,-1.4));
#11375=CARTESIAN_POINT('Ctrl Pts',(-17.6787134541915,3.67575622931334,7.));
#11376=CARTESIAN_POINT('Ctrl Pts',(-17.6787134541915,3.67575622931334,-1.4));
#11377=CARTESIAN_POINT('Ctrl Pts',(-17.9270849363835,3.63753969769581,7.));
#11378=CARTESIAN_POINT('Ctrl Pts',(-17.9270849363835,3.63753969769581,-1.4));
#11379=CARTESIAN_POINT('Ctrl Pts',(-18.265123941733,3.57255446932205,7.));
#11380=CARTESIAN_POINT('Ctrl Pts',(-18.265123941733,3.57255446932205,-1.4));
#11381=CARTESIAN_POINT('Ctrl Pts',(-18.5181384456163,3.51033578853423,7.));
#11382=CARTESIAN_POINT('Ctrl Pts',(-18.5181384456163,3.51033578853423,-1.4));
#11383=CARTESIAN_POINT('Ctrl Pts',(-18.6813621637973,3.46506965370702,7.));
#11384=CARTESIAN_POINT('Ctrl Pts',(-18.6813621637973,3.46506965370702,-1.4));
#11385=CARTESIAN_POINT('',(-18.6813621637973,3.46506965370702,7.));
#11386=CARTESIAN_POINT('Origin',(0.,0.,7.));
#11387=CARTESIAN_POINT('',(-18.8377966288375,2.47738131311205,7.));
#11388=CARTESIAN_POINT('Ctrl Pts',(-18.8377966288376,2.47738131311188,7.));
#11389=CARTESIAN_POINT('Ctrl Pts',(-18.8377966288376,2.47738131311188,-1.39999999999999));
#11390=CARTESIAN_POINT('Ctrl Pts',(-18.6965496529788,2.38389175781397,7.));
#11391=CARTESIAN_POINT('Ctrl Pts',(-18.6965496529788,2.38389175781397,-1.39999999999999));
#11392=CARTESIAN_POINT('Ctrl Pts',(-18.4751451900744,2.24653249449212,7.));
#11393=CARTESIAN_POINT('Ctrl Pts',(-18.4751451900744,2.24653249449212,-1.39999999999999));
#11394=CARTESIAN_POINT('Ctrl Pts',(-18.1737325312257,2.08026807216975,7.));
#11395=CARTESIAN_POINT('Ctrl Pts',(-18.1737325312257,2.08026807216975,-1.39999999999999));
#11396=CARTESIAN_POINT('Ctrl Pts',(-17.949326772361,1.96717098182926,7.));
#11397=CARTESIAN_POINT('Ctrl Pts',(-17.949326772361,1.96717098182926,-1.39999999999999));
#11398=CARTESIAN_POINT('Ctrl Pts',(-17.7407325407201,1.87160676754277,7.));
#11399=CARTESIAN_POINT('Ctrl Pts',(-17.7407325407201,1.87160676754277,-1.39999999999999));
#11400=CARTESIAN_POINT('Ctrl Pts',(-17.548917731071,1.79222730418272,7.));
#11401=CARTESIAN_POINT('Ctrl Pts',(-17.548917731071,1.79222730418272,-1.39999999999999));
#11402=CARTESIAN_POINT('Ctrl Pts',(-17.3747717371572,1.72763282051119,7.));
#11403=CARTESIAN_POINT('Ctrl Pts',(-17.3747717371572,1.72763282051119,-1.39999999999999));
#11404=CARTESIAN_POINT('Ctrl Pts',(-17.2191007779952,1.67639424155264,7.));
#11405=CARTESIAN_POINT('Ctrl Pts',(-17.2191007779952,1.67639424155264,-1.39999999999999));
#11406=CARTESIAN_POINT('Ctrl Pts',(-17.0826338282621,1.63700324669263,7.));
#11407=CARTESIAN_POINT('Ctrl Pts',(-17.0826338282621,1.63700324669263,-1.39999999999999));
#11408=CARTESIAN_POINT('Ctrl Pts',(-16.9659973771906,1.60803840593145,7.));
#11409=CARTESIAN_POINT('Ctrl Pts',(-16.9659973771906,1.60803840593145,-1.39999999999999));
#11410=CARTESIAN_POINT('Ctrl Pts',(-16.8793055486399,1.58971419725805,7.));
#11411=CARTESIAN_POINT('Ctrl Pts',(-16.8793055486399,1.58971419725805,-1.39999999999999));
#11412=CARTESIAN_POINT('Ctrl Pts',(-16.8195656763126,1.57930034717566,7.));
#11413=CARTESIAN_POINT('Ctrl Pts',(-16.8195656763126,1.57930034717566,-1.39999999999999));
#11414=CARTESIAN_POINT('Ctrl Pts',(-16.7804505865492,1.57225556404312,7.));
#11415=CARTESIAN_POINT('Ctrl Pts',(-16.7804505865492,1.57225556404312,-1.39999999999999));
#11416=CARTESIAN_POINT('Ctrl Pts',(-16.7455711436431,1.56489594057218,7.));
#11417=CARTESIAN_POINT('Ctrl Pts',(-16.7455711436431,1.56489594057218,-1.39999999999999));
#11418=CARTESIAN_POINT('Ctrl Pts',(-16.6896454316358,1.55162638755017,7.));
#11419=CARTESIAN_POINT('Ctrl Pts',(-16.6896454316358,1.55162638755017,-1.39999999999999));
#11420=CARTESIAN_POINT('Ctrl Pts',(-16.6138949491149,1.52918899676863,7.));
#11421=CARTESIAN_POINT('Ctrl Pts',(-16.6138949491149,1.52918899676863,-1.39999999999999));
#11422=CARTESIAN_POINT('Ctrl Pts',(-16.5198135565977,1.4905179616981,7.));
#11423=CARTESIAN_POINT('Ctrl Pts',(-16.5198135565977,1.4905179616981,-1.39999999999999));
#11424=CARTESIAN_POINT('Ctrl Pts',(-16.4279450992207,1.43783746532133,7.));
#11425=CARTESIAN_POINT('Ctrl Pts',(-16.4279450992207,1.43783746532133,-1.39999999999999));
#11426=CARTESIAN_POINT('Ctrl Pts',(-16.3372938385016,1.3620126454106,7.));
#11427=CARTESIAN_POINT('Ctrl Pts',(-16.3372938385016,1.3620126454106,-1.39999999999999));
#11428=CARTESIAN_POINT('Ctrl Pts',(-16.2452435266959,1.23650382033378,7.));
#11429=CARTESIAN_POINT('Ctrl Pts',(-16.2452435266959,1.23650382033378,-1.39999999999999));
#11430=CARTESIAN_POINT('Ctrl Pts',(-16.2167242606458,1.1199417984865,7.));
#11431=CARTESIAN_POINT('Ctrl Pts',(-16.2167242606458,1.1199417984865,-1.39999999999999));
#11432=CARTESIAN_POINT('Ctrl Pts',(-16.2160625265911,1.04967429885986,7.));
#11433=CARTESIAN_POINT('Ctrl Pts',(-16.2160625265911,1.04967429885986,-1.39999999999999));
#11434=CARTESIAN_POINT('Ctrl Pts',(-16.2160625265911,-1.04967429885984,
7.));
#11435=CARTESIAN_POINT('Ctrl Pts',(-16.2160625265911,-1.04967429885984,
-1.4));
#11436=CARTESIAN_POINT('Ctrl Pts',(-16.2167242606459,-1.11994179848649,
7.));
#11437=CARTESIAN_POINT('Ctrl Pts',(-16.2167242606459,-1.11994179848649,
-1.4));
#11438=CARTESIAN_POINT('Ctrl Pts',(-16.2452435266959,-1.23650382033376,
7.));
#11439=CARTESIAN_POINT('Ctrl Pts',(-16.2452435266959,-1.23650382033376,
-1.4));
#11440=CARTESIAN_POINT('Ctrl Pts',(-16.3372938385016,-1.36201264541056,
7.));
#11441=CARTESIAN_POINT('Ctrl Pts',(-16.3372938385016,-1.36201264541056,
-1.4));
#11442=CARTESIAN_POINT('Ctrl Pts',(-16.4279450992208,-1.43783746532131,
7.));
#11443=CARTESIAN_POINT('Ctrl Pts',(-16.4279450992208,-1.43783746532131,
-1.4));
#11444=CARTESIAN_POINT('Ctrl Pts',(-16.5198135565978,-1.49051796169811,
7.));
#11445=CARTESIAN_POINT('Ctrl Pts',(-16.5198135565978,-1.49051796169811,
-1.4));
#11446=CARTESIAN_POINT('Ctrl Pts',(-16.6138949491149,-1.52918899676863,
7.));
#11447=CARTESIAN_POINT('Ctrl Pts',(-16.6138949491149,-1.52918899676863,
-1.4));
#11448=CARTESIAN_POINT('Ctrl Pts',(-16.6896454316359,-1.55162638755017,
7.));
#11449=CARTESIAN_POINT('Ctrl Pts',(-16.6896454316359,-1.55162638755017,
-1.4));
#11450=CARTESIAN_POINT('Ctrl Pts',(-16.7455711436431,-1.56489594057219,
7.));
#11451=CARTESIAN_POINT('Ctrl Pts',(-16.7455711436431,-1.56489594057219,
-1.4));
#11452=CARTESIAN_POINT('Ctrl Pts',(-16.7804505865492,-1.57225556404312,
7.));
#11453=CARTESIAN_POINT('Ctrl Pts',(-16.7804505865492,-1.57225556404312,
-1.4));
#11454=CARTESIAN_POINT('Ctrl Pts',(-16.8195656763126,-1.57930034717562,
7.));
#11455=CARTESIAN_POINT('Ctrl Pts',(-16.8195656763126,-1.57930034717562,
-1.4));
#11456=CARTESIAN_POINT('Ctrl Pts',(-16.8793055486399,-1.58971419725805,
7.));
#11457=CARTESIAN_POINT('Ctrl Pts',(-16.8793055486399,-1.58971419725805,
-1.4));
#11458=CARTESIAN_POINT('Ctrl Pts',(-16.9659973771906,-1.60803840593145,
7.));
#11459=CARTESIAN_POINT('Ctrl Pts',(-16.9659973771906,-1.60803840593145,
-1.4));
#11460=CARTESIAN_POINT('Ctrl Pts',(-17.0826338282621,-1.63700324669261,
7.));
#11461=CARTESIAN_POINT('Ctrl Pts',(-17.0826338282621,-1.63700324669261,
-1.4));
#11462=CARTESIAN_POINT('Ctrl Pts',(-17.2191007779953,-1.67639424155264,
7.));
#11463=CARTESIAN_POINT('Ctrl Pts',(-17.2191007779953,-1.67639424155264,
-1.4));
#11464=CARTESIAN_POINT('Ctrl Pts',(-17.3747717371572,-1.72763282051121,
7.));
#11465=CARTESIAN_POINT('Ctrl Pts',(-17.3747717371572,-1.72763282051121,
-1.4));
#11466=CARTESIAN_POINT('Ctrl Pts',(-17.548917731071,-1.79222730418269,7.));
#11467=CARTESIAN_POINT('Ctrl Pts',(-17.548917731071,-1.79222730418269,-1.4));
#11468=CARTESIAN_POINT('Ctrl Pts',(-17.7407325407201,-1.87160676754278,
7.));
#11469=CARTESIAN_POINT('Ctrl Pts',(-17.7407325407201,-1.87160676754278,
-1.4));
#11470=CARTESIAN_POINT('Ctrl Pts',(-17.949326772361,-1.96717098182925,7.));
#11471=CARTESIAN_POINT('Ctrl Pts',(-17.949326772361,-1.96717098182925,-1.4));
#11472=CARTESIAN_POINT('Ctrl Pts',(-18.1737325312258,-2.08026807216972,
7.));
#11473=CARTESIAN_POINT('Ctrl Pts',(-18.1737325312258,-2.08026807216972,
-1.4));
#11474=CARTESIAN_POINT('Ctrl Pts',(-18.4751451900744,-2.2465324944921,7.));
#11475=CARTESIAN_POINT('Ctrl Pts',(-18.4751451900744,-2.2465324944921,-1.4));
#11476=CARTESIAN_POINT('Ctrl Pts',(-18.6965496529788,-2.38389175781394,
7.));
#11477=CARTESIAN_POINT('Ctrl Pts',(-18.6965496529788,-2.38389175781394,
-1.4));
#11478=CARTESIAN_POINT('Ctrl Pts',(-18.8377966288376,-2.47738131311187,
7.));
#11479=CARTESIAN_POINT('Ctrl Pts',(-18.8377966288376,-2.47738131311187,
-1.4));
#11480=CARTESIAN_POINT('',(-18.8377966288376,-2.47738131311187,7.));
#11481=CARTESIAN_POINT('Origin',(0.,0.,7.));
#11482=CARTESIAN_POINT('',(-18.6813621637974,-3.46506965370684,7.));
#11483=CARTESIAN_POINT('Ctrl Pts',(-18.6813621637974,-3.46506965370701,
7.));
#11484=CARTESIAN_POINT('Ctrl Pts',(-18.6813621637974,-3.46506965370701,
-1.39999999999999));
#11485=CARTESIAN_POINT('Ctrl Pts',(-18.5181384456162,-3.51033578853419,
7.));
#11486=CARTESIAN_POINT('Ctrl Pts',(-18.5181384456162,-3.51033578853419,
-1.39999999999999));
#11487=CARTESIAN_POINT('Ctrl Pts',(-18.265123941733,-3.57255446932203,7.));
#11488=CARTESIAN_POINT('Ctrl Pts',(-18.265123941733,-3.57255446932203,-1.39999999999999));
#11489=CARTESIAN_POINT('Ctrl Pts',(-17.9270849363835,-3.63753969769578,
7.));
#11490=CARTESIAN_POINT('Ctrl Pts',(-17.9270849363835,-3.63753969769578,
-1.39999999999999));
#11491=CARTESIAN_POINT('Ctrl Pts',(-17.6787134541915,-3.67575622931333,
7.));
#11492=CARTESIAN_POINT('Ctrl Pts',(-17.6787134541915,-3.67575622931333,
-1.39999999999999));
#11493=CARTESIAN_POINT('Ctrl Pts',(-17.4507975846592,-3.70218403552949,
7.));
#11494=CARTESIAN_POINT('Ctrl Pts',(-17.4507975846592,-3.70218403552949,
-1.39999999999999));
#11495=CARTESIAN_POINT('Ctrl Pts',(-17.2438412568379,-3.71840435546371,
7.));
#11496=CARTESIAN_POINT('Ctrl Pts',(-17.2438412568379,-3.71840435546371,
-1.39999999999999));
#11497=CARTESIAN_POINT('Ctrl Pts',(-17.0582577813421,-3.72602328845455,
7.));
#11498=CARTESIAN_POINT('Ctrl Pts',(-17.0582577813421,-3.72602328845455,
-1.39999999999999));
#11499=CARTESIAN_POINT('Ctrl Pts',(-16.8943723095674,-3.7266491009471,7.));
#11500=CARTESIAN_POINT('Ctrl Pts',(-16.8943723095674,-3.7266491009471,-1.39999999999999));
#11501=CARTESIAN_POINT('Ctrl Pts',(-16.7524120409277,-3.72194155665402,
7.));
#11502=CARTESIAN_POINT('Ctrl Pts',(-16.7524120409277,-3.72194155665402,
-1.39999999999999));
#11503=CARTESIAN_POINT('Ctrl Pts',(-16.632533556064,-3.7134461116587,7.));
#11504=CARTESIAN_POINT('Ctrl Pts',(-16.632533556064,-3.7134461116587,-1.39999999999999));
#11505=CARTESIAN_POINT('Ctrl Pts',(-16.5444222357228,-3.70408422142789,
7.));
#11506=CARTESIAN_POINT('Ctrl Pts',(-16.5444222357228,-3.70408422142789,
-1.39999999999999));
#11507=CARTESIAN_POINT('Ctrl Pts',(-16.4843881842109,-3.69552774561754,
7.));
#11508=CARTESIAN_POINT('Ctrl Pts',(-16.4843881842109,-3.69552774561754,
-1.39999999999999));
#11509=CARTESIAN_POINT('Ctrl Pts',(-16.4450105654964,-3.69014050504824,
7.));
#11510=CARTESIAN_POINT('Ctrl Pts',(-16.4450105654964,-3.69014050504824,
-1.39999999999999));
#11511=CARTESIAN_POINT('Ctrl Pts',(-16.409563995311,-3.68636158229544,7.));
#11512=CARTESIAN_POINT('Ctrl Pts',(-16.409563995311,-3.68636158229544,-1.39999999999999));
#11513=CARTESIAN_POINT('Ctrl Pts',(-16.3522749650865,-3.68169968173258,
7.));
#11514=CARTESIAN_POINT('Ctrl Pts',(-16.3522749650865,-3.68169968173258,
-1.39999999999999));
#11515=CARTESIAN_POINT('Ctrl Pts',(-16.2732984400115,-3.67963072201294,
7.));
#11516=CARTESIAN_POINT('Ctrl Pts',(-16.2732984400115,-3.67963072201294,
-1.39999999999999));
#11517=CARTESIAN_POINT('Ctrl Pts',(-16.1718717115691,-3.68733631276639,
7.));
#11518=CARTESIAN_POINT('Ctrl Pts',(-16.1718717115691,-3.68733631276639,
-1.39999999999999));
#11519=CARTESIAN_POINT('Ctrl Pts',(-16.0682204478862,-3.70904952755068,
7.));
#11520=CARTESIAN_POINT('Ctrl Pts',(-16.0682204478862,-3.70904952755068,
-1.39999999999999));
#11521=CARTESIAN_POINT('Ctrl Pts',(-15.958574817721,-3.75315043649995,7.));
#11522=CARTESIAN_POINT('Ctrl Pts',(-15.958574817721,-3.75315043649995,-1.39999999999999));
#11523=CARTESIAN_POINT('Ctrl Pts',(-15.8322454089585,-3.84407131175635,
7.));
#11524=CARTESIAN_POINT('Ctrl Pts',(-15.8322454089585,-3.84407131175635,
-1.39999999999999));
#11525=CARTESIAN_POINT('Ctrl Pts',(-15.7691023294921,-3.94611544431017,
7.));
#11526=CARTESIAN_POINT('Ctrl Pts',(-15.7691023294921,-3.94611544431017,
-1.39999999999999));
#11527=CARTESIAN_POINT('Ctrl Pts',(-15.7467591314705,-4.0127393206452,7.));
#11528=CARTESIAN_POINT('Ctrl Pts',(-15.7467591314705,-4.0127393206452,-1.39999999999999));
#11529=CARTESIAN_POINT('',(-15.7467591314705,-4.0127393206452,7.));
#11530=CARTESIAN_POINT('Origin',(0.,0.,7.));
#11531=CARTESIAN_POINT('',(-15.0980247376579,-6.00933848448149,7.));
#11532=CARTESIAN_POINT('Ctrl Pts',(-15.0980247376578,-6.00933848448161,
7.));
#11533=CARTESIAN_POINT('Ctrl Pts',(-15.0980247376578,-6.00933848448161,
-1.40000000000002));
#11534=CARTESIAN_POINT('Ctrl Pts',(-15.0769402326058,-6.07637133495397,
7.));
#11535=CARTESIAN_POINT('Ctrl Pts',(-15.0769402326058,-6.07637133495397,
-1.40000000000002));
#11536=CARTESIAN_POINT('Ctrl Pts',(-15.0680440207731,-6.19604134326091,
7.));
#11537=CARTESIAN_POINT('Ctrl Pts',(-15.0680440207731,-6.19604134326091,
-1.40000000000002));
#11538=CARTESIAN_POINT('Ctrl Pts',(-15.1168047097502,-6.34385243988823,
7.));
#11539=CARTESIAN_POINT('Ctrl Pts',(-15.1168047097502,-6.34385243988823,
-1.40000000000002));
#11540=CARTESIAN_POINT('Ctrl Pts',(-15.1795880240196,-6.44397890908498,
7.));
#11541=CARTESIAN_POINT('Ctrl Pts',(-15.1795880240196,-6.44397890908498,
-1.40000000000002));
#11542=CARTESIAN_POINT('Ctrl Pts',(-15.2506809503975,-6.52246995302231,
7.));
#11543=CARTESIAN_POINT('Ctrl Pts',(-15.2506809503975,-6.52246995302231,
-1.40000000000002));
#11544=CARTESIAN_POINT('Ctrl Pts',(-15.3282076647862,-6.58832104206025,
7.));
#11545=CARTESIAN_POINT('Ctrl Pts',(-15.3282076647862,-6.58832104206025,
-1.40000000000002));
#11546=CARTESIAN_POINT('Ctrl Pts',(-15.3933171197393,-6.63306845520279,
7.));
#11547=CARTESIAN_POINT('Ctrl Pts',(-15.3933171197393,-6.63306845520279,
-1.40000000000002));
#11548=CARTESIAN_POINT('Ctrl Pts',(-15.4424051151807,-6.66297054550545,
7.));
#11549=CARTESIAN_POINT('Ctrl Pts',(-15.4424051151807,-6.66297054550545,
-1.40000000000002));
#11550=CARTESIAN_POINT('Ctrl Pts',(-15.4733031879166,-6.68074830397729,
7.));
#11551=CARTESIAN_POINT('Ctrl Pts',(-15.4733031879166,-6.68074830397729,
-1.40000000000002));
#11552=CARTESIAN_POINT('Ctrl Pts',(-15.5083268912119,-6.69953551835472,
7.));
#11553=CARTESIAN_POINT('Ctrl Pts',(-15.5083268912119,-6.69953551835472,
-1.40000000000002));
#11554=CARTESIAN_POINT('Ctrl Pts',(-15.5619248294191,-6.72790031412626,
7.));
#11555=CARTESIAN_POINT('Ctrl Pts',(-15.5619248294191,-6.72790031412626,
-1.40000000000002));
#11556=CARTESIAN_POINT('Ctrl Pts',(-15.6387111659832,-6.77211692048665,
7.));
#11557=CARTESIAN_POINT('Ctrl Pts',(-15.6387111659832,-6.77211692048665,
-1.40000000000002));
#11558=CARTESIAN_POINT('Ctrl Pts',(-15.7406883947778,-6.8357067665807,7.));
#11559=CARTESIAN_POINT('Ctrl Pts',(-15.7406883947778,-6.8357067665807,-1.40000000000002));
#11560=CARTESIAN_POINT('Ctrl Pts',(-15.8583036897433,-6.91534043556372,
7.));
#11561=CARTESIAN_POINT('Ctrl Pts',(-15.8583036897433,-6.91534043556372,
-1.40000000000002));
#11562=CARTESIAN_POINT('Ctrl Pts',(-15.9905219781863,-7.01217619187965,
7.));
#11563=CARTESIAN_POINT('Ctrl Pts',(-15.9905219781863,-7.01217619187965,
-1.40000000000002));
#11564=CARTESIAN_POINT('Ctrl Pts',(-16.1361838672874,-7.12742326811382,
7.));
#11565=CARTESIAN_POINT('Ctrl Pts',(-16.1361838672874,-7.12742326811382,
-1.40000000000002));
#11566=CARTESIAN_POINT('Ctrl Pts',(-16.2940809887434,-7.26219165995681,
7.));
#11567=CARTESIAN_POINT('Ctrl Pts',(-16.2940809887434,-7.26219165995681,
-1.40000000000002));
#11568=CARTESIAN_POINT('Ctrl Pts',(-16.4629349257385,-7.41753779118423,
7.));
#11569=CARTESIAN_POINT('Ctrl Pts',(-16.4629349257385,-7.41753779118423,
-1.40000000000002));
#11570=CARTESIAN_POINT('Ctrl Pts',(-16.6414085620714,-7.59444470905136,
7.));
#11571=CARTESIAN_POINT('Ctrl Pts',(-16.6414085620714,-7.59444470905136,
-1.40000000000002));
#11572=CARTESIAN_POINT('Ctrl Pts',(-16.8766905033058,-7.84571320523309,
7.));
#11573=CARTESIAN_POINT('Ctrl Pts',(-16.8766905033058,-7.84571320523309,
-1.40000000000002));
#11574=CARTESIAN_POINT('Ctrl Pts',(-17.0448123137865,-8.04476736935674,
7.));
#11575=CARTESIAN_POINT('Ctrl Pts',(-17.0448123137865,-8.04476736935674,
-1.40000000000002));
#11576=CARTESIAN_POINT('Ctrl Pts',(-17.1502563092004,-8.1773289360728,7.));
#11577=CARTESIAN_POINT('Ctrl Pts',(-17.1502563092004,-8.1773289360728,-1.40000000000002));
#11578=CARTESIAN_POINT('',(-17.1502563092004,-8.1773289360728,7.));
#11579=CARTESIAN_POINT('Origin',(0.,0.,7.));
#11580=CARTESIAN_POINT('',(-16.6962658094609,-9.06833546026103,7.));
#11581=CARTESIAN_POINT('Ctrl Pts',(-16.6962658094608,-9.06833546026117,
7.));
#11582=CARTESIAN_POINT('Ctrl Pts',(-16.6962658094608,-9.06833546026117,
-1.39999999999999));
#11583=CARTESIAN_POINT('Ctrl Pts',(-16.5270428237395,-9.06094720995301,
7.));
#11584=CARTESIAN_POINT('Ctrl Pts',(-16.5270428237395,-9.06094720995301,
-1.39999999999999));
#11585=CARTESIAN_POINT('Ctrl Pts',(-16.2671851013731,-9.0419349102283,7.));
#11586=CARTESIAN_POINT('Ctrl Pts',(-16.2671851013731,-9.0419349102283,-1.39999999999999));
#11587=CARTESIAN_POINT('Ctrl Pts',(-15.9256093626227,-8.99927973772149,
7.));
#11588=CARTESIAN_POINT('Ctrl Pts',(-15.9256093626227,-8.99927973772149,
-1.39999999999999));
#11589=CARTESIAN_POINT('Ctrl Pts',(-15.6775844882862,-8.95887481023114,
7.));
#11590=CARTESIAN_POINT('Ctrl Pts',(-15.6775844882862,-8.95887481023114,
-1.39999999999999));
#11591=CARTESIAN_POINT('Ctrl Pts',(-15.4526569741556,-8.91357927057118,
7.));
#11592=CARTESIAN_POINT('Ctrl Pts',(-15.4526569741556,-8.91357927057118,
-1.39999999999999));
#11593=CARTESIAN_POINT('Ctrl Pts',(-15.2508174554788,-8.8650526891508,7.));
#11594=CARTESIAN_POINT('Ctrl Pts',(-15.2508174554788,-8.8650526891508,-1.39999999999999));
#11595=CARTESIAN_POINT('Ctrl Pts',(-15.0719627020186,-8.81495027721558,
7.));
#11596=CARTESIAN_POINT('Ctrl Pts',(-15.0719627020186,-8.81495027721558,
-1.39999999999999));
#11597=CARTESIAN_POINT('Ctrl Pts',(-14.9159049694657,-8.76490206435507,
7.));
#11598=CARTESIAN_POINT('Ctrl Pts',(-14.9159049694657,-8.76490206435507,
-1.39999999999999));
#11599=CARTESIAN_POINT('Ctrl Pts',(-14.7823474421093,-8.71655678814369,
7.));
#11600=CARTESIAN_POINT('Ctrl Pts',(-14.7823474421093,-8.71655678814369,
-1.39999999999999));
#11601=CARTESIAN_POINT('Ctrl Pts',(-14.6709614647944,-8.67143265073926,
7.));
#11602=CARTESIAN_POINT('Ctrl Pts',(-14.6709614647944,-8.67143265073926,
-1.39999999999999));
#11603=CARTESIAN_POINT('Ctrl Pts',(-14.5900556026053,-8.63530106864816,
7.));
#11604=CARTESIAN_POINT('Ctrl Pts',(-14.5900556026053,-8.63530106864816,
-1.39999999999999));
#11605=CARTESIAN_POINT('Ctrl Pts',(-14.5356039231527,-8.60861183441385,
7.));
#11606=CARTESIAN_POINT('Ctrl Pts',(-14.5356039231527,-8.60861183441385,
-1.39999999999999));
#11607=CARTESIAN_POINT('Ctrl Pts',(-14.4998183311667,-8.59131991078476,
7.));
#11608=CARTESIAN_POINT('Ctrl Pts',(-14.4998183311667,-8.59131991078476,
-1.39999999999999));
#11609=CARTESIAN_POINT('Ctrl Pts',(-14.4672743909627,-8.57677234909656,
7.));
#11610=CARTESIAN_POINT('Ctrl Pts',(-14.4672743909627,-8.57677234909656,
-1.39999999999999));
#11611=CARTESIAN_POINT('Ctrl Pts',(-14.4142298919554,-8.5546353342573,7.));
#11612=CARTESIAN_POINT('Ctrl Pts',(-14.4142298919554,-8.5546353342573,-1.39999999999999));
#11613=CARTESIAN_POINT('Ctrl Pts',(-14.3397580968625,-8.52826254822913,
7.));
#11614=CARTESIAN_POINT('Ctrl Pts',(-14.3397580968625,-8.52826254822913,
-1.39999999999999));
#11615=CARTESIAN_POINT('Ctrl Pts',(-14.2409143873564,-8.50424841775454,
7.));
#11616=CARTESIAN_POINT('Ctrl Pts',(-14.2409143873564,-8.50424841775454,
-1.39999999999999));
#11617=CARTESIAN_POINT('Ctrl Pts',(-14.1356264252376,-8.4928689101984,7.));
#11618=CARTESIAN_POINT('Ctrl Pts',(-14.1356264252376,-8.4928689101984,-1.39999999999999));
#11619=CARTESIAN_POINT('Ctrl Pts',(-14.0177193038531,-8.50092900394916,
7.));
#11620=CARTESIAN_POINT('Ctrl Pts',(-14.0177193038531,-8.50092900394916,
-1.39999999999999));
#11621=CARTESIAN_POINT('Ctrl Pts',(-13.8694768008521,-8.54836196063206,
7.));
#11622=CARTESIAN_POINT('Ctrl Pts',(-13.8694768008521,-8.54836196063206,
-1.39999999999999));
#11623=CARTESIAN_POINT('Ctrl Pts',(-13.7778907925313,-8.62589941321478,
7.));
#11624=CARTESIAN_POINT('Ctrl Pts',(-13.7778907925313,-8.62589941321478,
-1.39999999999999));
#11625=CARTESIAN_POINT('Ctrl Pts',(-13.7360532384392,-8.68235805704666,
7.));
#11626=CARTESIAN_POINT('Ctrl Pts',(-13.7360532384392,-8.68235805704666,
-1.39999999999999));
#11627=CARTESIAN_POINT('',(-13.7360532384392,-8.68235805704666,7.));
#11628=CARTESIAN_POINT('Origin',(0.,0.,7.));
#11629=CARTESIAN_POINT('',(-12.5020870932788,-10.380766749719,7.));
#11630=CARTESIAN_POINT('Ctrl Pts',(-12.5020870932787,-10.3807667497191,
7.));
#11631=CARTESIAN_POINT('Ctrl Pts',(-12.5020870932787,-10.3807667497191,
-1.4));
#11632=CARTESIAN_POINT('Ctrl Pts',(-12.4613202473788,-10.4380033085876,
7.));
#11633=CARTESIAN_POINT('Ctrl Pts',(-12.4613202473788,-10.4380033085876,
-1.4));
#11634=CARTESIAN_POINT('Ctrl Pts',(-12.4158793808611,-10.5490671691512,
7.));
#11635=CARTESIAN_POINT('Ctrl Pts',(-12.4158793808611,-10.5490671691512,
-1.4));
#11636=CARTESIAN_POINT('Ctrl Pts',(-12.4165774110367,-10.7047117573306,
7.));
#11637=CARTESIAN_POINT('Ctrl Pts',(-12.4165774110367,-10.7047117573306,
-1.4));
#11638=CARTESIAN_POINT('Ctrl Pts',(-12.4453471106188,-10.8193387993863,
7.));
#11639=CARTESIAN_POINT('Ctrl Pts',(-12.4453471106188,-10.8193387993863,
-1.4));
#11640=CARTESIAN_POINT('Ctrl Pts',(-12.4887054350301,-10.9159571406243,
7.));
#11641=CARTESIAN_POINT('Ctrl Pts',(-12.4887054350301,-10.9159571406243,
-1.4));
#11642=CARTESIAN_POINT('Ctrl Pts',(-12.5420886163255,-11.0025423202231,
7.));
#11643=CARTESIAN_POINT('Ctrl Pts',(-12.5420886163255,-11.0025423202231,
-1.4));
#11644=CARTESIAN_POINT('Ctrl Pts',(-12.5901836766158,-11.0652195671547,
7.));
#11645=CARTESIAN_POINT('Ctrl Pts',(-12.5901836766158,-11.0652195671547,
-1.4));
#11646=CARTESIAN_POINT('Ctrl Pts',(-12.6276288804813,-11.1088271697991,
7.));
#11647=CARTESIAN_POINT('Ctrl Pts',(-12.6276288804813,-11.1088271697991,
-1.4));
#11648=CARTESIAN_POINT('Ctrl Pts',(-12.6515210644081,-11.1352828524077,
7.));
#11649=CARTESIAN_POINT('Ctrl Pts',(-12.6515210644081,-11.1352828524077,
-1.4));
#11650=CARTESIAN_POINT('Ctrl Pts',(-12.6790250171322,-11.1639734745885,
7.));
#11651=CARTESIAN_POINT('Ctrl Pts',(-12.6790250171322,-11.1639734745885,
-1.4));
#11652=CARTESIAN_POINT('Ctrl Pts',(-12.7212344815888,-11.2075126722099,
7.));
#11653=CARTESIAN_POINT('Ctrl Pts',(-12.7212344815888,-11.2075126722099,
-1.4));
#11654=CARTESIAN_POINT('Ctrl Pts',(-12.7805989445416,-11.2732934467515,
7.));
#11655=CARTESIAN_POINT('Ctrl Pts',(-12.7805989445416,-11.2732934467515,
-1.4));
#11656=CARTESIAN_POINT('Ctrl Pts',(-12.8579347093876,-11.3652836809863,
7.));
#11657=CARTESIAN_POINT('Ctrl Pts',(-12.8579347093876,-11.3652836809863,
-1.4));
#11658=CARTESIAN_POINT('Ctrl Pts',(-12.9451853450404,-11.4773649257318,
7.));
#11659=CARTESIAN_POINT('Ctrl Pts',(-12.9451853450404,-11.4773649257318,
-1.4));
#11660=CARTESIAN_POINT('Ctrl Pts',(-13.0410085154727,-11.6103189008825,
7.));
#11661=CARTESIAN_POINT('Ctrl Pts',(-13.0410085154727,-11.6103189008825,
-1.4));
#11662=CARTESIAN_POINT('Ctrl Pts',(-13.1439278991698,-11.764937382884,7.));
#11663=CARTESIAN_POINT('Ctrl Pts',(-13.1439278991698,-11.764937382884,-1.4));
#11664=CARTESIAN_POINT('Ctrl Pts',(-13.2524512620508,-11.9419026340297,
7.));
#11665=CARTESIAN_POINT('Ctrl Pts',(-13.2524512620508,-11.9419026340297,
-1.4));
#11666=CARTESIAN_POINT('Ctrl Pts',(-13.3650363045724,-12.1418243205134,
7.));
#11667=CARTESIAN_POINT('Ctrl Pts',(-13.3650363045724,-12.1418243205134,
-1.4));
#11668=CARTESIAN_POINT('Ctrl Pts',(-13.4801075753502,-12.3652241842034,
7.));
#11669=CARTESIAN_POINT('Ctrl Pts',(-13.4801075753502,-12.3652241842034,
-1.4));
#11670=CARTESIAN_POINT('Ctrl Pts',(-13.6262277632565,-12.6769008431476,
7.));
#11671=CARTESIAN_POINT('Ctrl Pts',(-13.6262277632565,-12.6769008431476,
-1.4));
#11672=CARTESIAN_POINT('Ctrl Pts',(-13.7246099871303,-12.9181650995967,
7.));
#11673=CARTESIAN_POINT('Ctrl Pts',(-13.7246099871303,-12.9181650995967,
-1.4));
#11674=CARTESIAN_POINT('Ctrl Pts',(-13.7839294091566,-13.07682262797,7.));
#11675=CARTESIAN_POINT('Ctrl Pts',(-13.7839294091566,-13.07682262797,-1.4));
#11676=CARTESIAN_POINT('',(-13.7839294091566,-13.07682262797,7.));
#11677=CARTESIAN_POINT('Origin',(0.,0.,7.));
#11678=CARTESIAN_POINT('',(-13.0768226279701,-13.7839294091565,7.));
#11679=CARTESIAN_POINT('Ctrl Pts',(-13.07682262797,-13.7839294091566,7.));
#11680=CARTESIAN_POINT('Ctrl Pts',(-13.07682262797,-13.7839294091566,-1.39999999999999));
#11681=CARTESIAN_POINT('Ctrl Pts',(-12.9181650995967,-13.7246099871302,
7.));
#11682=CARTESIAN_POINT('Ctrl Pts',(-12.9181650995967,-13.7246099871302,
-1.39999999999999));
#11683=CARTESIAN_POINT('Ctrl Pts',(-12.6769008431476,-13.6262277632565,
7.));
#11684=CARTESIAN_POINT('Ctrl Pts',(-12.6769008431476,-13.6262277632565,
-1.39999999999999));
#11685=CARTESIAN_POINT('Ctrl Pts',(-12.3652241842034,-13.4801075753502,
7.));
#11686=CARTESIAN_POINT('Ctrl Pts',(-12.3652241842034,-13.4801075753502,
-1.39999999999999));
#11687=CARTESIAN_POINT('Ctrl Pts',(-12.1418243205134,-13.3650363045723,
7.));
#11688=CARTESIAN_POINT('Ctrl Pts',(-12.1418243205134,-13.3650363045723,
-1.39999999999999));
#11689=CARTESIAN_POINT('Ctrl Pts',(-11.9419026340297,-13.2524512620508,
7.));
#11690=CARTESIAN_POINT('Ctrl Pts',(-11.9419026340297,-13.2524512620508,
-1.39999999999999));
#11691=CARTESIAN_POINT('Ctrl Pts',(-11.764937382884,-13.1439278991698,7.));
#11692=CARTESIAN_POINT('Ctrl Pts',(-11.764937382884,-13.1439278991698,-1.39999999999999));
#11693=CARTESIAN_POINT('Ctrl Pts',(-11.6103189008825,-13.0410085154728,
7.));
#11694=CARTESIAN_POINT('Ctrl Pts',(-11.6103189008825,-13.0410085154728,
-1.39999999999999));
#11695=CARTESIAN_POINT('Ctrl Pts',(-11.4773649257318,-12.9451853450404,
7.));
#11696=CARTESIAN_POINT('Ctrl Pts',(-11.4773649257318,-12.9451853450404,
-1.39999999999999));
#11697=CARTESIAN_POINT('Ctrl Pts',(-11.3652836809863,-12.8579347093876,
7.));
#11698=CARTESIAN_POINT('Ctrl Pts',(-11.3652836809863,-12.8579347093876,
-1.39999999999999));
#11699=CARTESIAN_POINT('Ctrl Pts',(-11.2732934467515,-12.7805989445416,
7.));
#11700=CARTESIAN_POINT('Ctrl Pts',(-11.2732934467515,-12.7805989445416,
-1.39999999999999));
#11701=CARTESIAN_POINT('Ctrl Pts',(-11.2075126722099,-12.7212344815888,
7.));
#11702=CARTESIAN_POINT('Ctrl Pts',(-11.2075126722099,-12.7212344815888,
-1.39999999999999));
#11703=CARTESIAN_POINT('Ctrl Pts',(-11.1639734745886,-12.6790250171322,
7.));
#11704=CARTESIAN_POINT('Ctrl Pts',(-11.1639734745886,-12.6790250171322,
-1.39999999999999));
#11705=CARTESIAN_POINT('Ctrl Pts',(-11.1352828524077,-12.651521064408,7.));
#11706=CARTESIAN_POINT('Ctrl Pts',(-11.1352828524077,-12.651521064408,-1.39999999999999));
#11707=CARTESIAN_POINT('Ctrl Pts',(-11.1088271697991,-12.6276288804813,
7.));
#11708=CARTESIAN_POINT('Ctrl Pts',(-11.1088271697991,-12.6276288804813,
-1.39999999999999));
#11709=CARTESIAN_POINT('Ctrl Pts',(-11.0652195671547,-12.5901836766158,
7.));
#11710=CARTESIAN_POINT('Ctrl Pts',(-11.0652195671547,-12.5901836766158,
-1.39999999999999));
#11711=CARTESIAN_POINT('Ctrl Pts',(-11.0025423202231,-12.5420886163255,
7.));
#11712=CARTESIAN_POINT('Ctrl Pts',(-11.0025423202231,-12.5420886163255,
-1.39999999999999));
#11713=CARTESIAN_POINT('Ctrl Pts',(-10.9159571406243,-12.48870543503,7.));
#11714=CARTESIAN_POINT('Ctrl Pts',(-10.9159571406243,-12.48870543503,-1.39999999999999));
#11715=CARTESIAN_POINT('Ctrl Pts',(-10.8193387993863,-12.4453471106187,
7.));
#11716=CARTESIAN_POINT('Ctrl Pts',(-10.8193387993863,-12.4453471106187,
-1.39999999999999));
#11717=CARTESIAN_POINT('Ctrl Pts',(-10.7047117573307,-12.4165774110367,
7.));
#11718=CARTESIAN_POINT('Ctrl Pts',(-10.7047117573307,-12.4165774110367,
-1.39999999999999));
#11719=CARTESIAN_POINT('Ctrl Pts',(-10.5490671691512,-12.4158793808611,
7.));
#11720=CARTESIAN_POINT('Ctrl Pts',(-10.5490671691512,-12.4158793808611,
-1.39999999999999));
#11721=CARTESIAN_POINT('Ctrl Pts',(-10.4380033085876,-12.4613202473787,
7.));
#11722=CARTESIAN_POINT('Ctrl Pts',(-10.4380033085876,-12.4613202473787,
-1.39999999999999));
#11723=CARTESIAN_POINT('Ctrl Pts',(-10.3807667497191,-12.5020870932787,
7.));
#11724=CARTESIAN_POINT('Ctrl Pts',(-10.3807667497191,-12.5020870932787,
-1.39999999999999));
#11725=CARTESIAN_POINT('',(-10.3807667497191,-12.5020870932787,7.));
#11726=CARTESIAN_POINT('Origin',(0.,0.,7.));
#11727=CARTESIAN_POINT('',(-8.68235805704677,-13.7360532384392,7.));
#11728=CARTESIAN_POINT('Ctrl Pts',(-8.68235805704668,-13.7360532384392,
7.));
#11729=CARTESIAN_POINT('Ctrl Pts',(-8.68235805704668,-13.7360532384392,
-1.39999999999998));
#11730=CARTESIAN_POINT('Ctrl Pts',(-8.62589941321481,-13.7778907925313,
7.));
#11731=CARTESIAN_POINT('Ctrl Pts',(-8.62589941321481,-13.7778907925313,
-1.39999999999998));
#11732=CARTESIAN_POINT('Ctrl Pts',(-8.54836196063208,-13.8694768008521,
7.));
#11733=CARTESIAN_POINT('Ctrl Pts',(-8.54836196063208,-13.8694768008521,
-1.39999999999998));
#11734=CARTESIAN_POINT('Ctrl Pts',(-8.50092900394921,-14.0177193038531,
7.));
#11735=CARTESIAN_POINT('Ctrl Pts',(-8.50092900394921,-14.0177193038531,
-1.39999999999998));
#11736=CARTESIAN_POINT('Ctrl Pts',(-8.49286891019844,-14.1356264252377,
7.));
#11737=CARTESIAN_POINT('Ctrl Pts',(-8.49286891019844,-14.1356264252377,
-1.39999999999998));
#11738=CARTESIAN_POINT('Ctrl Pts',(-8.50424841775456,-14.2409143873564,
7.));
#11739=CARTESIAN_POINT('Ctrl Pts',(-8.50424841775456,-14.2409143873564,
-1.39999999999998));
#11740=CARTESIAN_POINT('Ctrl Pts',(-8.52826254822915,-14.3397580968626,
7.));
#11741=CARTESIAN_POINT('Ctrl Pts',(-8.52826254822915,-14.3397580968626,
-1.39999999999998));
#11742=CARTESIAN_POINT('Ctrl Pts',(-8.55463533425732,-14.4142298919555,
7.));
#11743=CARTESIAN_POINT('Ctrl Pts',(-8.55463533425732,-14.4142298919555,
-1.39999999999998));
#11744=CARTESIAN_POINT('Ctrl Pts',(-8.57677234909656,-14.4672743909627,
7.));
#11745=CARTESIAN_POINT('Ctrl Pts',(-8.57677234909656,-14.4672743909627,
-1.39999999999998));
#11746=CARTESIAN_POINT('Ctrl Pts',(-8.59131991078476,-14.4998183311667,
7.));
#11747=CARTESIAN_POINT('Ctrl Pts',(-8.59131991078476,-14.4998183311667,
-1.39999999999998));
#11748=CARTESIAN_POINT('Ctrl Pts',(-8.6086118344139,-14.5356039231527,7.));
#11749=CARTESIAN_POINT('Ctrl Pts',(-8.6086118344139,-14.5356039231527,-1.39999999999998));
#11750=CARTESIAN_POINT('Ctrl Pts',(-8.63530106864818,-14.5900556026053,
7.));
#11751=CARTESIAN_POINT('Ctrl Pts',(-8.63530106864818,-14.5900556026053,
-1.39999999999998));
#11752=CARTESIAN_POINT('Ctrl Pts',(-8.67143265073928,-14.6709614647944,
7.));
#11753=CARTESIAN_POINT('Ctrl Pts',(-8.67143265073928,-14.6709614647944,
-1.39999999999998));
#11754=CARTESIAN_POINT('Ctrl Pts',(-8.71655678814373,-14.7823474421093,
7.));
#11755=CARTESIAN_POINT('Ctrl Pts',(-8.71655678814373,-14.7823474421093,
-1.39999999999998));
#11756=CARTESIAN_POINT('Ctrl Pts',(-8.76490206435509,-14.9159049694657,
7.));
#11757=CARTESIAN_POINT('Ctrl Pts',(-8.76490206435509,-14.9159049694657,
-1.39999999999998));
#11758=CARTESIAN_POINT('Ctrl Pts',(-8.81495027721557,-15.0719627020186,
7.));
#11759=CARTESIAN_POINT('Ctrl Pts',(-8.81495027721557,-15.0719627020186,
-1.39999999999998));
#11760=CARTESIAN_POINT('Ctrl Pts',(-8.86505268915084,-15.2508174554788,
7.));
#11761=CARTESIAN_POINT('Ctrl Pts',(-8.86505268915084,-15.2508174554788,
-1.39999999999998));
#11762=CARTESIAN_POINT('Ctrl Pts',(-8.91357927057117,-15.4526569741556,
7.));
#11763=CARTESIAN_POINT('Ctrl Pts',(-8.91357927057117,-15.4526569741556,
-1.39999999999998));
#11764=CARTESIAN_POINT('Ctrl Pts',(-8.95887481023116,-15.6775844882862,
7.));
#11765=CARTESIAN_POINT('Ctrl Pts',(-8.95887481023116,-15.6775844882862,
-1.39999999999998));
#11766=CARTESIAN_POINT('Ctrl Pts',(-8.99927973772154,-15.9256093626227,
7.));
#11767=CARTESIAN_POINT('Ctrl Pts',(-8.99927973772154,-15.9256093626227,
-1.39999999999998));
#11768=CARTESIAN_POINT('Ctrl Pts',(-9.04193491022832,-16.2671851013731,
7.));
#11769=CARTESIAN_POINT('Ctrl Pts',(-9.04193491022832,-16.2671851013731,
-1.39999999999998));
#11770=CARTESIAN_POINT('Ctrl Pts',(-9.06094720995306,-16.5270428237395,
7.));
#11771=CARTESIAN_POINT('Ctrl Pts',(-9.06094720995306,-16.5270428237395,
-1.39999999999998));
#11772=CARTESIAN_POINT('Ctrl Pts',(-9.06833546026116,-16.6962658094608,
7.));
#11773=CARTESIAN_POINT('Ctrl Pts',(-9.06833546026116,-16.6962658094608,
-1.39999999999998));
#11774=CARTESIAN_POINT('',(-9.06833546026116,-16.6962658094608,7.));
#11775=CARTESIAN_POINT('Origin',(0.,0.,7.));
#11776=CARTESIAN_POINT('',(-8.17732893607292,-17.1502563092003,7.));
#11777=CARTESIAN_POINT('Ctrl Pts',(-8.1773289360728,-17.1502563092004,7.));
#11778=CARTESIAN_POINT('Ctrl Pts',(-8.1773289360728,-17.1502563092004,-1.39999999999998));
#11779=CARTESIAN_POINT('Ctrl Pts',(-8.04476736935674,-17.0448123137865,
7.));
#11780=CARTESIAN_POINT('Ctrl Pts',(-8.04476736935674,-17.0448123137865,
-1.39999999999998));
#11781=CARTESIAN_POINT('Ctrl Pts',(-7.8457132052331,-16.8766905033057,7.));
#11782=CARTESIAN_POINT('Ctrl Pts',(-7.8457132052331,-16.8766905033057,-1.39999999999998));
#11783=CARTESIAN_POINT('Ctrl Pts',(-7.59444470905137,-16.6414085620714,
7.));
#11784=CARTESIAN_POINT('Ctrl Pts',(-7.59444470905137,-16.6414085620714,
-1.39999999999998));
#11785=CARTESIAN_POINT('Ctrl Pts',(-7.41753779118422,-16.4629349257385,
7.));
#11786=CARTESIAN_POINT('Ctrl Pts',(-7.41753779118422,-16.4629349257385,
-1.39999999999998));
#11787=CARTESIAN_POINT('Ctrl Pts',(-7.2621916599568,-16.2940809887434,7.));
#11788=CARTESIAN_POINT('Ctrl Pts',(-7.2621916599568,-16.2940809887434,-1.39999999999998));
#11789=CARTESIAN_POINT('Ctrl Pts',(-7.12742326811384,-16.1361838672874,
7.));
#11790=CARTESIAN_POINT('Ctrl Pts',(-7.12742326811384,-16.1361838672874,
-1.39999999999998));
#11791=CARTESIAN_POINT('Ctrl Pts',(-7.01217619187963,-15.9905219781863,
7.));
#11792=CARTESIAN_POINT('Ctrl Pts',(-7.01217619187963,-15.9905219781863,
-1.39999999999998));
#11793=CARTESIAN_POINT('Ctrl Pts',(-6.9153404355637,-15.8583036897432,7.));
#11794=CARTESIAN_POINT('Ctrl Pts',(-6.9153404355637,-15.8583036897432,-1.39999999999998));
#11795=CARTESIAN_POINT('Ctrl Pts',(-6.8357067665807,-15.7406883947777,7.));
#11796=CARTESIAN_POINT('Ctrl Pts',(-6.8357067665807,-15.7406883947777,-1.39999999999998));
#11797=CARTESIAN_POINT('Ctrl Pts',(-6.77211692048664,-15.6387111659832,
7.));
#11798=CARTESIAN_POINT('Ctrl Pts',(-6.77211692048664,-15.6387111659832,
-1.39999999999998));
#11799=CARTESIAN_POINT('Ctrl Pts',(-6.72790031412625,-15.5619248294191,
7.));
#11800=CARTESIAN_POINT('Ctrl Pts',(-6.72790031412625,-15.5619248294191,
-1.39999999999998));
#11801=CARTESIAN_POINT('Ctrl Pts',(-6.69953551835473,-15.5083268912118,
7.));
#11802=CARTESIAN_POINT('Ctrl Pts',(-6.69953551835473,-15.5083268912118,
-1.39999999999998));
#11803=CARTESIAN_POINT('Ctrl Pts',(-6.68074830397727,-15.4733031879166,
7.));
#11804=CARTESIAN_POINT('Ctrl Pts',(-6.68074830397727,-15.4733031879166,
-1.39999999999998));
#11805=CARTESIAN_POINT('Ctrl Pts',(-6.66297054550543,-15.4424051151807,
7.));
#11806=CARTESIAN_POINT('Ctrl Pts',(-6.66297054550543,-15.4424051151807,
-1.39999999999998));
#11807=CARTESIAN_POINT('Ctrl Pts',(-6.63306845520277,-15.3933171197393,
7.));
#11808=CARTESIAN_POINT('Ctrl Pts',(-6.63306845520277,-15.3933171197393,
-1.39999999999998));
#11809=CARTESIAN_POINT('Ctrl Pts',(-6.58832104206024,-15.3282076647861,
7.));
#11810=CARTESIAN_POINT('Ctrl Pts',(-6.58832104206024,-15.3282076647861,
-1.39999999999998));
#11811=CARTESIAN_POINT('Ctrl Pts',(-6.52246995302227,-15.2506809503975,
7.));
#11812=CARTESIAN_POINT('Ctrl Pts',(-6.52246995302227,-15.2506809503975,
-1.39999999999998));
#11813=CARTESIAN_POINT('Ctrl Pts',(-6.44397890908497,-15.1795880240196,
7.));
#11814=CARTESIAN_POINT('Ctrl Pts',(-6.44397890908497,-15.1795880240196,
-1.39999999999998));
#11815=CARTESIAN_POINT('Ctrl Pts',(-6.34385243988824,-15.1168047097501,
7.));
#11816=CARTESIAN_POINT('Ctrl Pts',(-6.34385243988824,-15.1168047097501,
-1.39999999999998));
#11817=CARTESIAN_POINT('Ctrl Pts',(-6.19604134326091,-15.0680440207731,
7.));
#11818=CARTESIAN_POINT('Ctrl Pts',(-6.19604134326091,-15.0680440207731,
-1.39999999999998));
#11819=CARTESIAN_POINT('Ctrl Pts',(-6.07637133495395,-15.0769402326058,
7.));
#11820=CARTESIAN_POINT('Ctrl Pts',(-6.07637133495395,-15.0769402326058,
-1.39999999999998));
#11821=CARTESIAN_POINT('Ctrl Pts',(-6.0093384844816,-15.0980247376578,7.));
#11822=CARTESIAN_POINT('Ctrl Pts',(-6.0093384844816,-15.0980247376578,-1.39999999999998));
#11823=CARTESIAN_POINT('',(-6.0093384844816,-15.0980247376578,7.));
#11824=CARTESIAN_POINT('Origin',(0.,0.,7.));
#11825=CARTESIAN_POINT('',(-4.01273932064531,-15.7467591314704,7.));
#11826=CARTESIAN_POINT('Ctrl Pts',(-4.01273932064524,-15.7467591314704,
7.));
#11827=CARTESIAN_POINT('Ctrl Pts',(-4.01273932064524,-15.7467591314704,
-1.39999999999997));
#11828=CARTESIAN_POINT('Ctrl Pts',(-3.94611544431022,-15.7691023294921,
7.));
#11829=CARTESIAN_POINT('Ctrl Pts',(-3.94611544431022,-15.7691023294921,
-1.39999999999997));
#11830=CARTESIAN_POINT('Ctrl Pts',(-3.8440713117564,-15.8322454089585,7.));
#11831=CARTESIAN_POINT('Ctrl Pts',(-3.8440713117564,-15.8322454089585,-1.39999999999997));
#11832=CARTESIAN_POINT('Ctrl Pts',(-3.75315043650002,-15.958574817721,7.));
#11833=CARTESIAN_POINT('Ctrl Pts',(-3.75315043650002,-15.958574817721,-1.39999999999997));
#11834=CARTESIAN_POINT('Ctrl Pts',(-3.70904952755073,-16.0682204478862,
7.));
#11835=CARTESIAN_POINT('Ctrl Pts',(-3.70904952755073,-16.0682204478862,
-1.39999999999997));
#11836=CARTESIAN_POINT('Ctrl Pts',(-3.68733631276642,-16.1718717115691,
7.));
#11837=CARTESIAN_POINT('Ctrl Pts',(-3.68733631276642,-16.1718717115691,
-1.39999999999997));
#11838=CARTESIAN_POINT('Ctrl Pts',(-3.67963072201298,-16.2732984400115,
7.));
#11839=CARTESIAN_POINT('Ctrl Pts',(-3.67963072201298,-16.2732984400115,
-1.39999999999997));
#11840=CARTESIAN_POINT('Ctrl Pts',(-3.68169968173261,-16.3522749650865,
7.));
#11841=CARTESIAN_POINT('Ctrl Pts',(-3.68169968173261,-16.3522749650865,
-1.39999999999997));
#11842=CARTESIAN_POINT('Ctrl Pts',(-3.68636158229546,-16.409563995311,7.));
#11843=CARTESIAN_POINT('Ctrl Pts',(-3.68636158229546,-16.409563995311,-1.39999999999997));
#11844=CARTESIAN_POINT('Ctrl Pts',(-3.69014050504826,-16.4450105654963,
7.));
#11845=CARTESIAN_POINT('Ctrl Pts',(-3.69014050504826,-16.4450105654963,
-1.39999999999997));
#11846=CARTESIAN_POINT('Ctrl Pts',(-3.6955277456176,-16.4843881842109,7.));
#11847=CARTESIAN_POINT('Ctrl Pts',(-3.6955277456176,-16.4843881842109,-1.39999999999997));
#11848=CARTESIAN_POINT('Ctrl Pts',(-3.70408422142792,-16.5444222357228,
7.));
#11849=CARTESIAN_POINT('Ctrl Pts',(-3.70408422142792,-16.5444222357228,
-1.39999999999997));
#11850=CARTESIAN_POINT('Ctrl Pts',(-3.71344611165872,-16.632533556064,7.));
#11851=CARTESIAN_POINT('Ctrl Pts',(-3.71344611165872,-16.632533556064,-1.39999999999997));
#11852=CARTESIAN_POINT('Ctrl Pts',(-3.72194155665407,-16.7524120409277,
7.));
#11853=CARTESIAN_POINT('Ctrl Pts',(-3.72194155665407,-16.7524120409277,
-1.39999999999997));
#11854=CARTESIAN_POINT('Ctrl Pts',(-3.72664910094713,-16.8943723095674,
7.));
#11855=CARTESIAN_POINT('Ctrl Pts',(-3.72664910094713,-16.8943723095674,
-1.39999999999997));
#11856=CARTESIAN_POINT('Ctrl Pts',(-3.72602328845455,-17.0582577813421,
7.));
#11857=CARTESIAN_POINT('Ctrl Pts',(-3.72602328845455,-17.0582577813421,
-1.39999999999997));
#11858=CARTESIAN_POINT('Ctrl Pts',(-3.71840435546375,-17.2438412568379,
7.));
#11859=CARTESIAN_POINT('Ctrl Pts',(-3.71840435546375,-17.2438412568379,
-1.39999999999997));
#11860=CARTESIAN_POINT('Ctrl Pts',(-3.70218403552949,-17.4507975846592,
7.));
#11861=CARTESIAN_POINT('Ctrl Pts',(-3.70218403552949,-17.4507975846592,
-1.39999999999997));
#11862=CARTESIAN_POINT('Ctrl Pts',(-3.67575622931335,-17.6787134541915,
7.));
#11863=CARTESIAN_POINT('Ctrl Pts',(-3.67575622931335,-17.6787134541915,
-1.39999999999997));
#11864=CARTESIAN_POINT('Ctrl Pts',(-3.63753969769582,-17.9270849363835,
7.));
#11865=CARTESIAN_POINT('Ctrl Pts',(-3.63753969769582,-17.9270849363835,
-1.39999999999997));
#11866=CARTESIAN_POINT('Ctrl Pts',(-3.57255446932205,-18.265123941733,7.));
#11867=CARTESIAN_POINT('Ctrl Pts',(-3.57255446932205,-18.265123941733,-1.39999999999997));
#11868=CARTESIAN_POINT('Ctrl Pts',(-3.51033578853422,-18.5181384456163,
7.));
#11869=CARTESIAN_POINT('Ctrl Pts',(-3.51033578853422,-18.5181384456163,
-1.39999999999997));
#11870=CARTESIAN_POINT('Ctrl Pts',(-3.46506965370701,-18.6813621637973,
7.));
#11871=CARTESIAN_POINT('Ctrl Pts',(-3.46506965370701,-18.6813621637973,
-1.39999999999997));
#11872=CARTESIAN_POINT('',(-3.46506965370701,-18.6813621637973,7.));
#11873=CARTESIAN_POINT('Origin',(0.,0.,7.));
#11874=CARTESIAN_POINT('',(-2.47738131311198,-18.8377966288376,7.));
#11875=CARTESIAN_POINT('Ctrl Pts',(-2.47738131311189,-18.8377966288376,
7.));
#11876=CARTESIAN_POINT('Ctrl Pts',(-2.47738131311189,-18.8377966288376,
-1.39999999999999));
#11877=CARTESIAN_POINT('Ctrl Pts',(-2.38389175781398,-18.6965496529788,
7.));
#11878=CARTESIAN_POINT('Ctrl Pts',(-2.38389175781398,-18.6965496529788,
-1.39999999999999));
#11879=CARTESIAN_POINT('Ctrl Pts',(-2.24653249449213,-18.4751451900744,
7.));
#11880=CARTESIAN_POINT('Ctrl Pts',(-2.24653249449213,-18.4751451900744,
-1.39999999999999));
#11881=CARTESIAN_POINT('Ctrl Pts',(-2.08026807216976,-18.1737325312257,
7.));
#11882=CARTESIAN_POINT('Ctrl Pts',(-2.08026807216976,-18.1737325312257,
-1.39999999999999));
#11883=CARTESIAN_POINT('Ctrl Pts',(-1.96717098182926,-17.949326772361,7.));
#11884=CARTESIAN_POINT('Ctrl Pts',(-1.96717098182926,-17.949326772361,-1.39999999999999));
#11885=CARTESIAN_POINT('Ctrl Pts',(-1.87160676754278,-17.7407325407201,
7.));
#11886=CARTESIAN_POINT('Ctrl Pts',(-1.87160676754278,-17.7407325407201,
-1.39999999999999));
#11887=CARTESIAN_POINT('Ctrl Pts',(-1.79222730418273,-17.548917731071,7.));
#11888=CARTESIAN_POINT('Ctrl Pts',(-1.79222730418273,-17.548917731071,-1.39999999999999));
#11889=CARTESIAN_POINT('Ctrl Pts',(-1.7276328205112,-17.3747717371572,7.));
#11890=CARTESIAN_POINT('Ctrl Pts',(-1.7276328205112,-17.3747717371572,-1.39999999999999));
#11891=CARTESIAN_POINT('Ctrl Pts',(-1.67639424155264,-17.2191007779952,
7.));
#11892=CARTESIAN_POINT('Ctrl Pts',(-1.67639424155264,-17.2191007779952,
-1.39999999999999));
#11893=CARTESIAN_POINT('Ctrl Pts',(-1.63700324669264,-17.0826338282621,
7.));
#11894=CARTESIAN_POINT('Ctrl Pts',(-1.63700324669264,-17.0826338282621,
-1.39999999999999));
#11895=CARTESIAN_POINT('Ctrl Pts',(-1.60803840593146,-16.9659973771906,
7.));
#11896=CARTESIAN_POINT('Ctrl Pts',(-1.60803840593146,-16.9659973771906,
-1.39999999999999));
#11897=CARTESIAN_POINT('Ctrl Pts',(-1.58971419725806,-16.8793055486399,
7.));
#11898=CARTESIAN_POINT('Ctrl Pts',(-1.58971419725806,-16.8793055486399,
-1.39999999999999));
#11899=CARTESIAN_POINT('Ctrl Pts',(-1.57930034717566,-16.8195656763126,
7.));
#11900=CARTESIAN_POINT('Ctrl Pts',(-1.57930034717566,-16.8195656763126,
-1.39999999999999));
#11901=CARTESIAN_POINT('Ctrl Pts',(-1.57225556404312,-16.7804505865492,
7.));
#11902=CARTESIAN_POINT('Ctrl Pts',(-1.57225556404312,-16.7804505865492,
-1.39999999999999));
#11903=CARTESIAN_POINT('Ctrl Pts',(-1.56489594057218,-16.7455711436431,
7.));
#11904=CARTESIAN_POINT('Ctrl Pts',(-1.56489594057218,-16.7455711436431,
-1.39999999999999));
#11905=CARTESIAN_POINT('Ctrl Pts',(-1.55162638755018,-16.6896454316358,
7.));
#11906=CARTESIAN_POINT('Ctrl Pts',(-1.55162638755018,-16.6896454316358,
-1.39999999999999));
#11907=CARTESIAN_POINT('Ctrl Pts',(-1.52918899676863,-16.6138949491149,
7.));
#11908=CARTESIAN_POINT('Ctrl Pts',(-1.52918899676863,-16.6138949491149,
-1.39999999999999));
#11909=CARTESIAN_POINT('Ctrl Pts',(-1.49051796169811,-16.5198135565977,
7.));
#11910=CARTESIAN_POINT('Ctrl Pts',(-1.49051796169811,-16.5198135565977,
-1.39999999999999));
#11911=CARTESIAN_POINT('Ctrl Pts',(-1.43783746532133,-16.4279450992207,
7.));
#11912=CARTESIAN_POINT('Ctrl Pts',(-1.43783746532133,-16.4279450992207,
-1.39999999999999));
#11913=CARTESIAN_POINT('Ctrl Pts',(-1.3620126454106,-16.3372938385016,7.));
#11914=CARTESIAN_POINT('Ctrl Pts',(-1.3620126454106,-16.3372938385016,-1.39999999999999));
#11915=CARTESIAN_POINT('Ctrl Pts',(-1.23650382033378,-16.2452435266959,
7.));
#11916=CARTESIAN_POINT('Ctrl Pts',(-1.23650382033378,-16.2452435266959,
-1.39999999999999));
#11917=CARTESIAN_POINT('Ctrl Pts',(-1.1199417984865,-16.2167242606458,7.));
#11918=CARTESIAN_POINT('Ctrl Pts',(-1.1199417984865,-16.2167242606458,-1.39999999999999));
#11919=CARTESIAN_POINT('Ctrl Pts',(-1.04967429885986,-16.2160625265911,
7.));
#11920=CARTESIAN_POINT('Ctrl Pts',(-1.04967429885986,-16.2160625265911,
-1.39999999999999));
#11921=CARTESIAN_POINT('',(-1.04967429885986,-16.2160625265911,7.));
#11922=CARTESIAN_POINT('Origin',(0.,0.,7.));
#11923=CARTESIAN_POINT('',(1.04967429885974,-16.2160625265911,7.));
#11924=CARTESIAN_POINT('Ctrl Pts',(1.04967429885983,-16.2160625265911,7.));
#11925=CARTESIAN_POINT('Ctrl Pts',(1.04967429885983,-16.2160625265911,-1.4));
#11926=CARTESIAN_POINT('Ctrl Pts',(1.11994179848648,-16.2167242606459,7.));
#11927=CARTESIAN_POINT('Ctrl Pts',(1.11994179848648,-16.2167242606459,-1.4));
#11928=CARTESIAN_POINT('Ctrl Pts',(1.23650382033375,-16.2452435266959,7.));
#11929=CARTESIAN_POINT('Ctrl Pts',(1.23650382033375,-16.2452435266959,-1.4));
#11930=CARTESIAN_POINT('Ctrl Pts',(1.36201264541055,-16.3372938385016,7.));
#11931=CARTESIAN_POINT('Ctrl Pts',(1.36201264541055,-16.3372938385016,-1.4));
#11932=CARTESIAN_POINT('Ctrl Pts',(1.4378374653213,-16.4279450992208,7.));
#11933=CARTESIAN_POINT('Ctrl Pts',(1.4378374653213,-16.4279450992208,-1.4));
#11934=CARTESIAN_POINT('Ctrl Pts',(1.4905179616981,-16.5198135565978,7.));
#11935=CARTESIAN_POINT('Ctrl Pts',(1.4905179616981,-16.5198135565978,-1.4));
#11936=CARTESIAN_POINT('Ctrl Pts',(1.52918899676862,-16.6138949491149,7.));
#11937=CARTESIAN_POINT('Ctrl Pts',(1.52918899676862,-16.6138949491149,-1.4));
#11938=CARTESIAN_POINT('Ctrl Pts',(1.55162638755016,-16.6896454316359,7.));
#11939=CARTESIAN_POINT('Ctrl Pts',(1.55162638755016,-16.6896454316359,-1.4));
#11940=CARTESIAN_POINT('Ctrl Pts',(1.56489594057218,-16.7455711436431,7.));
#11941=CARTESIAN_POINT('Ctrl Pts',(1.56489594057218,-16.7455711436431,-1.4));
#11942=CARTESIAN_POINT('Ctrl Pts',(1.57225556404312,-16.7804505865492,7.));
#11943=CARTESIAN_POINT('Ctrl Pts',(1.57225556404312,-16.7804505865492,-1.4));
#11944=CARTESIAN_POINT('Ctrl Pts',(1.57930034717562,-16.8195656763126,7.));
#11945=CARTESIAN_POINT('Ctrl Pts',(1.57930034717562,-16.8195656763126,-1.4));
#11946=CARTESIAN_POINT('Ctrl Pts',(1.58971419725804,-16.8793055486399,7.));
#11947=CARTESIAN_POINT('Ctrl Pts',(1.58971419725804,-16.8793055486399,-1.4));
#11948=CARTESIAN_POINT('Ctrl Pts',(1.60803840593144,-16.9659973771906,7.));
#11949=CARTESIAN_POINT('Ctrl Pts',(1.60803840593144,-16.9659973771906,-1.4));
#11950=CARTESIAN_POINT('Ctrl Pts',(1.6370032466926,-17.0826338282622,7.));
#11951=CARTESIAN_POINT('Ctrl Pts',(1.6370032466926,-17.0826338282622,-1.4));
#11952=CARTESIAN_POINT('Ctrl Pts',(1.67639424155263,-17.2191007779953,7.));
#11953=CARTESIAN_POINT('Ctrl Pts',(1.67639424155263,-17.2191007779953,-1.4));
#11954=CARTESIAN_POINT('Ctrl Pts',(1.72763282051121,-17.3747717371572,7.));
#11955=CARTESIAN_POINT('Ctrl Pts',(1.72763282051121,-17.3747717371572,-1.4));
#11956=CARTESIAN_POINT('Ctrl Pts',(1.79222730418269,-17.548917731071,7.));
#11957=CARTESIAN_POINT('Ctrl Pts',(1.79222730418269,-17.548917731071,-1.4));
#11958=CARTESIAN_POINT('Ctrl Pts',(1.87160676754277,-17.7407325407201,7.));
#11959=CARTESIAN_POINT('Ctrl Pts',(1.87160676754277,-17.7407325407201,-1.4));
#11960=CARTESIAN_POINT('Ctrl Pts',(1.96717098182925,-17.949326772361,7.));
#11961=CARTESIAN_POINT('Ctrl Pts',(1.96717098182925,-17.949326772361,-1.4));
#11962=CARTESIAN_POINT('Ctrl Pts',(2.08026807216972,-18.1737325312257,7.));
#11963=CARTESIAN_POINT('Ctrl Pts',(2.08026807216972,-18.1737325312257,-1.4));
#11964=CARTESIAN_POINT('Ctrl Pts',(2.2465324944921,-18.4751451900744,7.));
#11965=CARTESIAN_POINT('Ctrl Pts',(2.2465324944921,-18.4751451900744,-1.4));
#11966=CARTESIAN_POINT('Ctrl Pts',(2.38389175781394,-18.6965496529788,7.));
#11967=CARTESIAN_POINT('Ctrl Pts',(2.38389175781394,-18.6965496529788,-1.4));
#11968=CARTESIAN_POINT('Ctrl Pts',(2.47738131311187,-18.8377966288376,7.));
#11969=CARTESIAN_POINT('Ctrl Pts',(2.47738131311187,-18.8377966288376,-1.4));
#11970=CARTESIAN_POINT('',(2.47738131311187,-18.8377966288376,7.));
#11971=CARTESIAN_POINT('Origin',(0.,0.,7.));
#11972=CARTESIAN_POINT('',(3.46506965370692,-18.6813621637974,7.));
#11973=CARTESIAN_POINT('Ctrl Pts',(3.46506965370701,-18.6813621637973,7.));
#11974=CARTESIAN_POINT('Ctrl Pts',(3.46506965370701,-18.6813621637973,-1.39999999999999));
#11975=CARTESIAN_POINT('Ctrl Pts',(3.51033578853419,-18.5181384456162,7.));
#11976=CARTESIAN_POINT('Ctrl Pts',(3.51033578853419,-18.5181384456162,-1.39999999999999));
#11977=CARTESIAN_POINT('Ctrl Pts',(3.57255446932203,-18.2651239417329,7.));
#11978=CARTESIAN_POINT('Ctrl Pts',(3.57255446932203,-18.2651239417329,-1.39999999999999));
#11979=CARTESIAN_POINT('Ctrl Pts',(3.63753969769579,-17.9270849363835,7.));
#11980=CARTESIAN_POINT('Ctrl Pts',(3.63753969769579,-17.9270849363835,-1.39999999999999));
#11981=CARTESIAN_POINT('Ctrl Pts',(3.67575622931334,-17.6787134541915,7.));
#11982=CARTESIAN_POINT('Ctrl Pts',(3.67575622931334,-17.6787134541915,-1.39999999999999));
#11983=CARTESIAN_POINT('Ctrl Pts',(3.7021840355295,-17.4507975846592,7.));
#11984=CARTESIAN_POINT('Ctrl Pts',(3.7021840355295,-17.4507975846592,-1.39999999999999));
#11985=CARTESIAN_POINT('Ctrl Pts',(3.71840435546372,-17.2438412568379,7.));
#11986=CARTESIAN_POINT('Ctrl Pts',(3.71840435546372,-17.2438412568379,-1.39999999999999));
#11987=CARTESIAN_POINT('Ctrl Pts',(3.72602328845457,-17.0582577813421,7.));
#11988=CARTESIAN_POINT('Ctrl Pts',(3.72602328845457,-17.0582577813421,-1.39999999999999));
#11989=CARTESIAN_POINT('Ctrl Pts',(3.72664910094712,-16.8943723095674,7.));
#11990=CARTESIAN_POINT('Ctrl Pts',(3.72664910094712,-16.8943723095674,-1.39999999999999));
#11991=CARTESIAN_POINT('Ctrl Pts',(3.72194155665404,-16.7524120409277,7.));
#11992=CARTESIAN_POINT('Ctrl Pts',(3.72194155665404,-16.7524120409277,-1.39999999999999));
#11993=CARTESIAN_POINT('Ctrl Pts',(3.71344611165872,-16.632533556064,7.));
#11994=CARTESIAN_POINT('Ctrl Pts',(3.71344611165872,-16.632533556064,-1.39999999999999));
#11995=CARTESIAN_POINT('Ctrl Pts',(3.70408422142791,-16.5444222357228,7.));
#11996=CARTESIAN_POINT('Ctrl Pts',(3.70408422142791,-16.5444222357228,-1.39999999999999));
#11997=CARTESIAN_POINT('Ctrl Pts',(3.69552774561757,-16.4843881842109,7.));
#11998=CARTESIAN_POINT('Ctrl Pts',(3.69552774561757,-16.4843881842109,-1.39999999999999));
#11999=CARTESIAN_POINT('Ctrl Pts',(3.69014050504827,-16.4450105654963,7.));
#12000=CARTESIAN_POINT('Ctrl Pts',(3.69014050504827,-16.4450105654963,-1.39999999999999));
#12001=CARTESIAN_POINT('Ctrl Pts',(3.68636158229547,-16.409563995311,7.));
#12002=CARTESIAN_POINT('Ctrl Pts',(3.68636158229547,-16.409563995311,-1.39999999999999));
#12003=CARTESIAN_POINT('Ctrl Pts',(3.68169968173261,-16.3522749650865,7.));
#12004=CARTESIAN_POINT('Ctrl Pts',(3.68169968173261,-16.3522749650865,-1.39999999999999));
#12005=CARTESIAN_POINT('Ctrl Pts',(3.67963072201297,-16.2732984400115,7.));
#12006=CARTESIAN_POINT('Ctrl Pts',(3.67963072201297,-16.2732984400115,-1.39999999999999));
#12007=CARTESIAN_POINT('Ctrl Pts',(3.68733631276642,-16.1718717115691,7.));
#12008=CARTESIAN_POINT('Ctrl Pts',(3.68733631276642,-16.1718717115691,-1.39999999999999));
#12009=CARTESIAN_POINT('Ctrl Pts',(3.70904952755071,-16.0682204478862,7.));
#12010=CARTESIAN_POINT('Ctrl Pts',(3.70904952755071,-16.0682204478862,-1.39999999999999));
#12011=CARTESIAN_POINT('Ctrl Pts',(3.75315043649999,-15.958574817721,7.));
#12012=CARTESIAN_POINT('Ctrl Pts',(3.75315043649999,-15.958574817721,-1.39999999999999));
#12013=CARTESIAN_POINT('Ctrl Pts',(3.84407131175639,-15.8322454089585,7.));
#12014=CARTESIAN_POINT('Ctrl Pts',(3.84407131175639,-15.8322454089585,-1.39999999999999));
#12015=CARTESIAN_POINT('Ctrl Pts',(3.94611544431021,-15.7691023294921,7.));
#12016=CARTESIAN_POINT('Ctrl Pts',(3.94611544431021,-15.7691023294921,-1.39999999999999));
#12017=CARTESIAN_POINT('Ctrl Pts',(4.01273932064523,-15.7467591314704,7.));
#12018=CARTESIAN_POINT('Ctrl Pts',(4.01273932064523,-15.7467591314704,-1.39999999999999));
#12019=CARTESIAN_POINT('',(4.01273932064523,-15.7467591314704,7.));
#12020=CARTESIAN_POINT('Origin',(0.,0.,7.));
#12021=CARTESIAN_POINT('',(6.00933848448151,-15.0980247376579,7.));
#12022=CARTESIAN_POINT('Ctrl Pts',(6.00933848448159,-15.0980247376579,7.));
#12023=CARTESIAN_POINT('Ctrl Pts',(6.00933848448159,-15.0980247376579,-1.4));
#12024=CARTESIAN_POINT('Ctrl Pts',(6.07637133495396,-15.0769402326058,7.));
#12025=CARTESIAN_POINT('Ctrl Pts',(6.07637133495396,-15.0769402326058,-1.4));
#12026=CARTESIAN_POINT('Ctrl Pts',(6.1960413432609,-15.0680440207731,7.));
#12027=CARTESIAN_POINT('Ctrl Pts',(6.1960413432609,-15.0680440207731,-1.4));
#12028=CARTESIAN_POINT('Ctrl Pts',(6.34385243988821,-15.1168047097502,7.));
#12029=CARTESIAN_POINT('Ctrl Pts',(6.34385243988821,-15.1168047097502,-1.4));
#12030=CARTESIAN_POINT('Ctrl Pts',(6.44397890908497,-15.1795880240196,7.));
#12031=CARTESIAN_POINT('Ctrl Pts',(6.44397890908497,-15.1795880240196,-1.4));
#12032=CARTESIAN_POINT('Ctrl Pts',(6.52246995302229,-15.2506809503975,7.));
#12033=CARTESIAN_POINT('Ctrl Pts',(6.52246995302229,-15.2506809503975,-1.4));
#12034=CARTESIAN_POINT('Ctrl Pts',(6.58832104206024,-15.3282076647862,7.));
#12035=CARTESIAN_POINT('Ctrl Pts',(6.58832104206024,-15.3282076647862,-1.4));
#12036=CARTESIAN_POINT('Ctrl Pts',(6.63306845520277,-15.3933171197393,7.));
#12037=CARTESIAN_POINT('Ctrl Pts',(6.63306845520277,-15.3933171197393,-1.4));
#12038=CARTESIAN_POINT('Ctrl Pts',(6.66297054550544,-15.4424051151807,7.));
#12039=CARTESIAN_POINT('Ctrl Pts',(6.66297054550544,-15.4424051151807,-1.4));
#12040=CARTESIAN_POINT('Ctrl Pts',(6.68074830397727,-15.4733031879166,7.));
#12041=CARTESIAN_POINT('Ctrl Pts',(6.68074830397727,-15.4733031879166,-1.4));
#12042=CARTESIAN_POINT('Ctrl Pts',(6.69953551835471,-15.5083268912119,7.));
#12043=CARTESIAN_POINT('Ctrl Pts',(6.69953551835471,-15.5083268912119,-1.4));
#12044=CARTESIAN_POINT('Ctrl Pts',(6.72790031412625,-15.5619248294191,7.));
#12045=CARTESIAN_POINT('Ctrl Pts',(6.72790031412625,-15.5619248294191,-1.4));
#12046=CARTESIAN_POINT('Ctrl Pts',(6.77211692048664,-15.6387111659832,7.));
#12047=CARTESIAN_POINT('Ctrl Pts',(6.77211692048664,-15.6387111659832,-1.4));
#12048=CARTESIAN_POINT('Ctrl Pts',(6.83570676658069,-15.7406883947778,7.));
#12049=CARTESIAN_POINT('Ctrl Pts',(6.83570676658069,-15.7406883947778,-1.4));
#12050=CARTESIAN_POINT('Ctrl Pts',(6.91534043556371,-15.8583036897433,7.));
#12051=CARTESIAN_POINT('Ctrl Pts',(6.91534043556371,-15.8583036897433,-1.4));
#12052=CARTESIAN_POINT('Ctrl Pts',(7.01217619187964,-15.9905219781863,7.));
#12053=CARTESIAN_POINT('Ctrl Pts',(7.01217619187964,-15.9905219781863,-1.4));
#12054=CARTESIAN_POINT('Ctrl Pts',(7.12742326811382,-16.1361838672874,7.));
#12055=CARTESIAN_POINT('Ctrl Pts',(7.12742326811382,-16.1361838672874,-1.4));
#12056=CARTESIAN_POINT('Ctrl Pts',(7.2621916599568,-16.2940809887434,7.));
#12057=CARTESIAN_POINT('Ctrl Pts',(7.2621916599568,-16.2940809887434,-1.4));
#12058=CARTESIAN_POINT('Ctrl Pts',(7.41753779118422,-16.4629349257385,7.));
#12059=CARTESIAN_POINT('Ctrl Pts',(7.41753779118422,-16.4629349257385,-1.4));
#12060=CARTESIAN_POINT('Ctrl Pts',(7.59444470905135,-16.6414085620714,7.));
#12061=CARTESIAN_POINT('Ctrl Pts',(7.59444470905135,-16.6414085620714,-1.4));
#12062=CARTESIAN_POINT('Ctrl Pts',(7.84571320523309,-16.8766905033058,7.));
#12063=CARTESIAN_POINT('Ctrl Pts',(7.84571320523309,-16.8766905033058,-1.4));
#12064=CARTESIAN_POINT('Ctrl Pts',(8.04476736935673,-17.0448123137865,7.));
#12065=CARTESIAN_POINT('Ctrl Pts',(8.04476736935673,-17.0448123137865,-1.4));
#12066=CARTESIAN_POINT('Ctrl Pts',(8.17732893607279,-17.1502563092004,7.));
#12067=CARTESIAN_POINT('Ctrl Pts',(8.17732893607279,-17.1502563092004,-1.4));
#12068=CARTESIAN_POINT('',(8.17732893607279,-17.1502563092004,7.));
#12069=CARTESIAN_POINT('Origin',(0.,0.,7.));
#12070=CARTESIAN_POINT('',(9.06833546026109,-16.6962658094609,7.));
#12071=CARTESIAN_POINT('Ctrl Pts',(9.06833546026116,-16.6962658094608,7.));
#12072=CARTESIAN_POINT('Ctrl Pts',(9.06833546026116,-16.6962658094608,-1.39999999999999));
#12073=CARTESIAN_POINT('Ctrl Pts',(9.06094720995301,-16.5270428237395,7.));
#12074=CARTESIAN_POINT('Ctrl Pts',(9.06094720995301,-16.5270428237395,-1.39999999999999));
#12075=CARTESIAN_POINT('Ctrl Pts',(9.0419349102283,-16.267185101373,7.));
#12076=CARTESIAN_POINT('Ctrl Pts',(9.0419349102283,-16.267185101373,-1.39999999999999));
#12077=CARTESIAN_POINT('Ctrl Pts',(8.99927973772149,-15.9256093626227,7.));
#12078=CARTESIAN_POINT('Ctrl Pts',(8.99927973772149,-15.9256093626227,-1.39999999999999));
#12079=CARTESIAN_POINT('Ctrl Pts',(8.95887481023114,-15.6775844882862,7.));
#12080=CARTESIAN_POINT('Ctrl Pts',(8.95887481023114,-15.6775844882862,-1.39999999999999));
#12081=CARTESIAN_POINT('Ctrl Pts',(8.91357927057119,-15.4526569741556,7.));
#12082=CARTESIAN_POINT('Ctrl Pts',(8.91357927057119,-15.4526569741556,-1.39999999999999));
#12083=CARTESIAN_POINT('Ctrl Pts',(8.8650526891508,-15.2508174554787,7.));
#12084=CARTESIAN_POINT('Ctrl Pts',(8.8650526891508,-15.2508174554787,-1.39999999999999));
#12085=CARTESIAN_POINT('Ctrl Pts',(8.81495027721559,-15.0719627020186,7.));
#12086=CARTESIAN_POINT('Ctrl Pts',(8.81495027721559,-15.0719627020186,-1.39999999999999));
#12087=CARTESIAN_POINT('Ctrl Pts',(8.76490206435508,-14.9159049694657,7.));
#12088=CARTESIAN_POINT('Ctrl Pts',(8.76490206435508,-14.9159049694657,-1.39999999999999));
#12089=CARTESIAN_POINT('Ctrl Pts',(8.7165567881437,-14.7823474421092,7.));
#12090=CARTESIAN_POINT('Ctrl Pts',(8.7165567881437,-14.7823474421092,-1.39999999999999));
#12091=CARTESIAN_POINT('Ctrl Pts',(8.67143265073927,-14.6709614647944,7.));
#12092=CARTESIAN_POINT('Ctrl Pts',(8.67143265073927,-14.6709614647944,-1.39999999999999));
#12093=CARTESIAN_POINT('Ctrl Pts',(8.63530106864817,-14.5900556026053,7.));
#12094=CARTESIAN_POINT('Ctrl Pts',(8.63530106864817,-14.5900556026053,-1.39999999999999));
#12095=CARTESIAN_POINT('Ctrl Pts',(8.60861183441386,-14.5356039231526,7.));
#12096=CARTESIAN_POINT('Ctrl Pts',(8.60861183441386,-14.5356039231526,-1.39999999999999));
#12097=CARTESIAN_POINT('Ctrl Pts',(8.59131991078477,-14.4998183311667,7.));
#12098=CARTESIAN_POINT('Ctrl Pts',(8.59131991078477,-14.4998183311667,-1.39999999999999));
#12099=CARTESIAN_POINT('Ctrl Pts',(8.57677234909656,-14.4672743909626,7.));
#12100=CARTESIAN_POINT('Ctrl Pts',(8.57677234909656,-14.4672743909626,-1.39999999999999));
#12101=CARTESIAN_POINT('Ctrl Pts',(8.55463533425731,-14.4142298919554,7.));
#12102=CARTESIAN_POINT('Ctrl Pts',(8.55463533425731,-14.4142298919554,-1.39999999999999));
#12103=CARTESIAN_POINT('Ctrl Pts',(8.52826254822914,-14.3397580968625,7.));
#12104=CARTESIAN_POINT('Ctrl Pts',(8.52826254822914,-14.3397580968625,-1.39999999999999));
#12105=CARTESIAN_POINT('Ctrl Pts',(8.50424841775455,-14.2409143873564,7.));
#12106=CARTESIAN_POINT('Ctrl Pts',(8.50424841775455,-14.2409143873564,-1.39999999999999));
#12107=CARTESIAN_POINT('Ctrl Pts',(8.49286891019841,-14.1356264252376,7.));
#12108=CARTESIAN_POINT('Ctrl Pts',(8.49286891019841,-14.1356264252376,-1.39999999999999));
#12109=CARTESIAN_POINT('Ctrl Pts',(8.50092900394917,-14.0177193038531,7.));
#12110=CARTESIAN_POINT('Ctrl Pts',(8.50092900394917,-14.0177193038531,-1.39999999999999));
#12111=CARTESIAN_POINT('Ctrl Pts',(8.54836196063206,-13.8694768008521,7.));
#12112=CARTESIAN_POINT('Ctrl Pts',(8.54836196063206,-13.8694768008521,-1.39999999999999));
#12113=CARTESIAN_POINT('Ctrl Pts',(8.62589941321478,-13.7778907925312,7.));
#12114=CARTESIAN_POINT('Ctrl Pts',(8.62589941321478,-13.7778907925312,-1.39999999999999));
#12115=CARTESIAN_POINT('Ctrl Pts',(8.68235805704667,-13.7360532384392,7.));
#12116=CARTESIAN_POINT('Ctrl Pts',(8.68235805704667,-13.7360532384392,-1.39999999999999));
#12117=CARTESIAN_POINT('',(8.68235805704667,-13.7360532384392,7.));
#12118=CARTESIAN_POINT('Origin',(0.,0.,7.));
#12119=CARTESIAN_POINT('',(10.3807667497191,-12.5020870932787,7.));
#12120=CARTESIAN_POINT('Ctrl Pts',(10.3807667497191,-12.5020870932787,7.));
#12121=CARTESIAN_POINT('Ctrl Pts',(10.3807667497191,-12.5020870932787,-1.4));
#12122=CARTESIAN_POINT('Ctrl Pts',(10.4380033085876,-12.4613202473788,7.));
#12123=CARTESIAN_POINT('Ctrl Pts',(10.4380033085876,-12.4613202473788,-1.4));
#12124=CARTESIAN_POINT('Ctrl Pts',(10.5490671691512,-12.4158793808611,7.));
#12125=CARTESIAN_POINT('Ctrl Pts',(10.5490671691512,-12.4158793808611,-1.4));
#12126=CARTESIAN_POINT('Ctrl Pts',(10.7047117573306,-12.4165774110367,7.));
#12127=CARTESIAN_POINT('Ctrl Pts',(10.7047117573306,-12.4165774110367,-1.4));
#12128=CARTESIAN_POINT('Ctrl Pts',(10.8193387993863,-12.4453471106188,7.));
#12129=CARTESIAN_POINT('Ctrl Pts',(10.8193387993863,-12.4453471106188,-1.4));
#12130=CARTESIAN_POINT('Ctrl Pts',(10.9159571406243,-12.48870543503,7.));
#12131=CARTESIAN_POINT('Ctrl Pts',(10.9159571406243,-12.48870543503,-1.4));
#12132=CARTESIAN_POINT('Ctrl Pts',(11.0025423202231,-12.5420886163255,7.));
#12133=CARTESIAN_POINT('Ctrl Pts',(11.0025423202231,-12.5420886163255,-1.4));
#12134=CARTESIAN_POINT('Ctrl Pts',(11.0652195671547,-12.5901836766158,7.));
#12135=CARTESIAN_POINT('Ctrl Pts',(11.0652195671547,-12.5901836766158,-1.4));
#12136=CARTESIAN_POINT('Ctrl Pts',(11.1088271697991,-12.6276288804813,7.));
#12137=CARTESIAN_POINT('Ctrl Pts',(11.1088271697991,-12.6276288804813,-1.4));
#12138=CARTESIAN_POINT('Ctrl Pts',(11.1352828524077,-12.651521064408,7.));
#12139=CARTESIAN_POINT('Ctrl Pts',(11.1352828524077,-12.651521064408,-1.4));
#12140=CARTESIAN_POINT('Ctrl Pts',(11.1639734745885,-12.6790250171322,7.));
#12141=CARTESIAN_POINT('Ctrl Pts',(11.1639734745885,-12.6790250171322,-1.4));
#12142=CARTESIAN_POINT('Ctrl Pts',(11.2075126722099,-12.7212344815888,7.));
#12143=CARTESIAN_POINT('Ctrl Pts',(11.2075126722099,-12.7212344815888,-1.4));
#12144=CARTESIAN_POINT('Ctrl Pts',(11.2732934467515,-12.7805989445416,7.));
#12145=CARTESIAN_POINT('Ctrl Pts',(11.2732934467515,-12.7805989445416,-1.4));
#12146=CARTESIAN_POINT('Ctrl Pts',(11.3652836809863,-12.8579347093876,7.));
#12147=CARTESIAN_POINT('Ctrl Pts',(11.3652836809863,-12.8579347093876,-1.4));
#12148=CARTESIAN_POINT('Ctrl Pts',(11.4773649257318,-12.9451853450404,7.));
#12149=CARTESIAN_POINT('Ctrl Pts',(11.4773649257318,-12.9451853450404,-1.4));
#12150=CARTESIAN_POINT('Ctrl Pts',(11.6103189008825,-13.0410085154727,7.));
#12151=CARTESIAN_POINT('Ctrl Pts',(11.6103189008825,-13.0410085154727,-1.4));
#12152=CARTESIAN_POINT('Ctrl Pts',(11.764937382884,-13.1439278991698,7.));
#12153=CARTESIAN_POINT('Ctrl Pts',(11.764937382884,-13.1439278991698,-1.4));
#12154=CARTESIAN_POINT('Ctrl Pts',(11.9419026340297,-13.2524512620507,7.));
#12155=CARTESIAN_POINT('Ctrl Pts',(11.9419026340297,-13.2524512620507,-1.4));
#12156=CARTESIAN_POINT('Ctrl Pts',(12.1418243205134,-13.3650363045724,7.));
#12157=CARTESIAN_POINT('Ctrl Pts',(12.1418243205134,-13.3650363045724,-1.4));
#12158=CARTESIAN_POINT('Ctrl Pts',(12.3652241842034,-13.4801075753502,7.));
#12159=CARTESIAN_POINT('Ctrl Pts',(12.3652241842034,-13.4801075753502,-1.4));
#12160=CARTESIAN_POINT('Ctrl Pts',(12.6769008431476,-13.6262277632565,7.));
#12161=CARTESIAN_POINT('Ctrl Pts',(12.6769008431476,-13.6262277632565,-1.4));
#12162=CARTESIAN_POINT('Ctrl Pts',(12.9181650995967,-13.7246099871303,7.));
#12163=CARTESIAN_POINT('Ctrl Pts',(12.9181650995967,-13.7246099871303,-1.4));
#12164=CARTESIAN_POINT('Ctrl Pts',(13.07682262797,-13.7839294091566,7.));
#12165=CARTESIAN_POINT('Ctrl Pts',(13.07682262797,-13.7839294091566,-1.4));
#12166=CARTESIAN_POINT('',(13.07682262797,-13.7839294091566,7.));
#12167=CARTESIAN_POINT('Origin',(0.,1.10390771809154E-15,7.));
#12168=CARTESIAN_POINT('',(13.7839294091565,-13.0768226279701,7.));
#12169=CARTESIAN_POINT('Ctrl Pts',(13.7839294091566,-13.07682262797,7.));
#12170=CARTESIAN_POINT('Ctrl Pts',(13.7839294091566,-13.07682262797,-1.39999999999999));
#12171=CARTESIAN_POINT('Ctrl Pts',(13.7246099871302,-12.9181650995967,7.));
#12172=CARTESIAN_POINT('Ctrl Pts',(13.7246099871302,-12.9181650995967,-1.39999999999999));
#12173=CARTESIAN_POINT('Ctrl Pts',(13.6262277632565,-12.6769008431476,7.));
#12174=CARTESIAN_POINT('Ctrl Pts',(13.6262277632565,-12.6769008431476,-1.39999999999999));
#12175=CARTESIAN_POINT('Ctrl Pts',(13.4801075753502,-12.3652241842034,7.));
#12176=CARTESIAN_POINT('Ctrl Pts',(13.4801075753502,-12.3652241842034,-1.39999999999999));
#12177=CARTESIAN_POINT('Ctrl Pts',(13.3650363045723,-12.1418243205134,7.));
#12178=CARTESIAN_POINT('Ctrl Pts',(13.3650363045723,-12.1418243205134,-1.39999999999999));
#12179=CARTESIAN_POINT('Ctrl Pts',(13.2524512620508,-11.9419026340297,7.));
#12180=CARTESIAN_POINT('Ctrl Pts',(13.2524512620508,-11.9419026340297,-1.39999999999999));
#12181=CARTESIAN_POINT('Ctrl Pts',(13.1439278991698,-11.764937382884,7.));
#12182=CARTESIAN_POINT('Ctrl Pts',(13.1439278991698,-11.764937382884,-1.39999999999999));
#12183=CARTESIAN_POINT('Ctrl Pts',(13.0410085154728,-11.6103189008825,7.));
#12184=CARTESIAN_POINT('Ctrl Pts',(13.0410085154728,-11.6103189008825,-1.39999999999999));
#12185=CARTESIAN_POINT('Ctrl Pts',(12.9451853450404,-11.4773649257318,7.));
#12186=CARTESIAN_POINT('Ctrl Pts',(12.9451853450404,-11.4773649257318,-1.39999999999999));
#12187=CARTESIAN_POINT('Ctrl Pts',(12.8579347093876,-11.3652836809863,7.));
#12188=CARTESIAN_POINT('Ctrl Pts',(12.8579347093876,-11.3652836809863,-1.39999999999999));
#12189=CARTESIAN_POINT('Ctrl Pts',(12.7805989445416,-11.2732934467515,7.));
#12190=CARTESIAN_POINT('Ctrl Pts',(12.7805989445416,-11.2732934467515,-1.39999999999999));
#12191=CARTESIAN_POINT('Ctrl Pts',(12.7212344815888,-11.2075126722099,7.));
#12192=CARTESIAN_POINT('Ctrl Pts',(12.7212344815888,-11.2075126722099,-1.39999999999999));
#12193=CARTESIAN_POINT('Ctrl Pts',(12.6790250171322,-11.1639734745885,7.));
#12194=CARTESIAN_POINT('Ctrl Pts',(12.6790250171322,-11.1639734745885,-1.39999999999999));
#12195=CARTESIAN_POINT('Ctrl Pts',(12.6515210644081,-11.1352828524076,7.));
#12196=CARTESIAN_POINT('Ctrl Pts',(12.6515210644081,-11.1352828524076,-1.39999999999999));
#12197=CARTESIAN_POINT('Ctrl Pts',(12.6276288804813,-11.108827169799,7.));
#12198=CARTESIAN_POINT('Ctrl Pts',(12.6276288804813,-11.108827169799,-1.39999999999999));
#12199=CARTESIAN_POINT('Ctrl Pts',(12.5901836766158,-11.0652195671547,7.));
#12200=CARTESIAN_POINT('Ctrl Pts',(12.5901836766158,-11.0652195671547,-1.39999999999999));
#12201=CARTESIAN_POINT('Ctrl Pts',(12.5420886163255,-11.0025423202231,7.));
#12202=CARTESIAN_POINT('Ctrl Pts',(12.5420886163255,-11.0025423202231,-1.39999999999999));
#12203=CARTESIAN_POINT('Ctrl Pts',(12.48870543503,-10.9159571406243,7.));
#12204=CARTESIAN_POINT('Ctrl Pts',(12.48870543503,-10.9159571406243,-1.39999999999999));
#12205=CARTESIAN_POINT('Ctrl Pts',(12.4453471106188,-10.8193387993863,7.));
#12206=CARTESIAN_POINT('Ctrl Pts',(12.4453471106188,-10.8193387993863,-1.39999999999999));
#12207=CARTESIAN_POINT('Ctrl Pts',(12.4165774110367,-10.7047117573306,7.));
#12208=CARTESIAN_POINT('Ctrl Pts',(12.4165774110367,-10.7047117573306,-1.39999999999999));
#12209=CARTESIAN_POINT('Ctrl Pts',(12.4158793808611,-10.5490671691512,7.));
#12210=CARTESIAN_POINT('Ctrl Pts',(12.4158793808611,-10.5490671691512,-1.39999999999999));
#12211=CARTESIAN_POINT('Ctrl Pts',(12.4613202473788,-10.4380033085876,7.));
#12212=CARTESIAN_POINT('Ctrl Pts',(12.4613202473788,-10.4380033085876,-1.39999999999999));
#12213=CARTESIAN_POINT('Ctrl Pts',(12.5020870932787,-10.3807667497191,7.));
#12214=CARTESIAN_POINT('Ctrl Pts',(12.5020870932787,-10.3807667497191,-1.39999999999999));
#12215=CARTESIAN_POINT('',(12.5020870932787,-10.3807667497191,7.));
#12216=CARTESIAN_POINT('Origin',(0.,0.,7.));
#12217=CARTESIAN_POINT('',(13.7360532384392,-8.68235805704669,7.));
#12218=CARTESIAN_POINT('Ctrl Pts',(13.7360532384392,-8.68235805704669,7.));
#12219=CARTESIAN_POINT('Ctrl Pts',(13.7360532384392,-8.68235805704669,-1.39999999999998));
#12220=CARTESIAN_POINT('Ctrl Pts',(13.7778907925313,-8.62589941321482,7.));
#12221=CARTESIAN_POINT('Ctrl Pts',(13.7778907925313,-8.62589941321482,-1.39999999999998));
#12222=CARTESIAN_POINT('Ctrl Pts',(13.8694768008521,-8.54836196063209,7.));
#12223=CARTESIAN_POINT('Ctrl Pts',(13.8694768008521,-8.54836196063209,-1.39999999999998));
#12224=CARTESIAN_POINT('Ctrl Pts',(14.0177193038531,-8.50092900394922,7.));
#12225=CARTESIAN_POINT('Ctrl Pts',(14.0177193038531,-8.50092900394922,-1.39999999999998));
#12226=CARTESIAN_POINT('Ctrl Pts',(14.1356264252377,-8.49286891019844,7.));
#12227=CARTESIAN_POINT('Ctrl Pts',(14.1356264252377,-8.49286891019844,-1.39999999999998));
#12228=CARTESIAN_POINT('Ctrl Pts',(14.2409143873564,-8.50424841775457,7.));
#12229=CARTESIAN_POINT('Ctrl Pts',(14.2409143873564,-8.50424841775457,-1.39999999999998));
#12230=CARTESIAN_POINT('Ctrl Pts',(14.3397580968626,-8.52826254822916,7.));
#12231=CARTESIAN_POINT('Ctrl Pts',(14.3397580968626,-8.52826254822916,-1.39999999999998));
#12232=CARTESIAN_POINT('Ctrl Pts',(14.4142298919554,-8.55463533425733,7.));
#12233=CARTESIAN_POINT('Ctrl Pts',(14.4142298919554,-8.55463533425733,-1.39999999999998));
#12234=CARTESIAN_POINT('Ctrl Pts',(14.4672743909627,-8.57677234909657,7.));
#12235=CARTESIAN_POINT('Ctrl Pts',(14.4672743909627,-8.57677234909657,-1.39999999999998));
#12236=CARTESIAN_POINT('Ctrl Pts',(14.4998183311667,-8.59131991078477,7.));
#12237=CARTESIAN_POINT('Ctrl Pts',(14.4998183311667,-8.59131991078477,-1.39999999999998));
#12238=CARTESIAN_POINT('Ctrl Pts',(14.5356039231527,-8.6086118344139,7.));
#12239=CARTESIAN_POINT('Ctrl Pts',(14.5356039231527,-8.6086118344139,-1.39999999999998));
#12240=CARTESIAN_POINT('Ctrl Pts',(14.5900556026053,-8.63530106864818,7.));
#12241=CARTESIAN_POINT('Ctrl Pts',(14.5900556026053,-8.63530106864818,-1.39999999999998));
#12242=CARTESIAN_POINT('Ctrl Pts',(14.6709614647944,-8.67143265073928,7.));
#12243=CARTESIAN_POINT('Ctrl Pts',(14.6709614647944,-8.67143265073928,-1.39999999999998));
#12244=CARTESIAN_POINT('Ctrl Pts',(14.7823474421092,-8.71655678814373,7.));
#12245=CARTESIAN_POINT('Ctrl Pts',(14.7823474421092,-8.71655678814373,-1.39999999999998));
#12246=CARTESIAN_POINT('Ctrl Pts',(14.9159049694657,-8.7649020643551,7.));
#12247=CARTESIAN_POINT('Ctrl Pts',(14.9159049694657,-8.7649020643551,-1.39999999999998));
#12248=CARTESIAN_POINT('Ctrl Pts',(15.0719627020186,-8.81495027721557,7.));
#12249=CARTESIAN_POINT('Ctrl Pts',(15.0719627020186,-8.81495027721557,-1.39999999999998));
#12250=CARTESIAN_POINT('Ctrl Pts',(15.2508174554788,-8.86505268915084,7.));
#12251=CARTESIAN_POINT('Ctrl Pts',(15.2508174554788,-8.86505268915084,-1.39999999999998));
#12252=CARTESIAN_POINT('Ctrl Pts',(15.4526569741556,-8.91357927057117,7.));
#12253=CARTESIAN_POINT('Ctrl Pts',(15.4526569741556,-8.91357927057117,-1.39999999999998));
#12254=CARTESIAN_POINT('Ctrl Pts',(15.6775844882862,-8.95887481023116,7.));
#12255=CARTESIAN_POINT('Ctrl Pts',(15.6775844882862,-8.95887481023116,-1.39999999999998));
#12256=CARTESIAN_POINT('Ctrl Pts',(15.9256093626227,-8.99927973772153,7.));
#12257=CARTESIAN_POINT('Ctrl Pts',(15.9256093626227,-8.99927973772153,-1.39999999999998));
#12258=CARTESIAN_POINT('Ctrl Pts',(16.2671851013731,-9.04193491022831,7.));
#12259=CARTESIAN_POINT('Ctrl Pts',(16.2671851013731,-9.04193491022831,-1.39999999999998));
#12260=CARTESIAN_POINT('Ctrl Pts',(16.5270428237395,-9.06094720995305,7.));
#12261=CARTESIAN_POINT('Ctrl Pts',(16.5270428237395,-9.06094720995305,-1.39999999999998));
#12262=CARTESIAN_POINT('Ctrl Pts',(16.6962658094608,-9.06833546026116,7.));
#12263=CARTESIAN_POINT('Ctrl Pts',(16.6962658094608,-9.06833546026116,-1.39999999999998));
#12264=CARTESIAN_POINT('',(16.6962658094608,-9.06833546026116,7.));
#12265=CARTESIAN_POINT('Origin',(0.,0.,7.));
#12266=CARTESIAN_POINT('',(17.1502563092003,-8.17732893607285,7.));
#12267=CARTESIAN_POINT('Ctrl Pts',(17.1502563092004,-8.17732893607279,7.));
#12268=CARTESIAN_POINT('Ctrl Pts',(17.1502563092004,-8.17732893607279,-1.39999999999999));
#12269=CARTESIAN_POINT('Ctrl Pts',(17.0448123137865,-8.04476736935674,7.));
#12270=CARTESIAN_POINT('Ctrl Pts',(17.0448123137865,-8.04476736935674,-1.39999999999999));
#12271=CARTESIAN_POINT('Ctrl Pts',(16.8766905033057,-7.84571320523309,7.));
#12272=CARTESIAN_POINT('Ctrl Pts',(16.8766905033057,-7.84571320523309,-1.39999999999999));
#12273=CARTESIAN_POINT('Ctrl Pts',(16.6414085620714,-7.59444470905136,7.));
#12274=CARTESIAN_POINT('Ctrl Pts',(16.6414085620714,-7.59444470905136,-1.39999999999999));
#12275=CARTESIAN_POINT('Ctrl Pts',(16.4629349257385,-7.41753779118421,7.));
#12276=CARTESIAN_POINT('Ctrl Pts',(16.4629349257385,-7.41753779118421,-1.39999999999999));
#12277=CARTESIAN_POINT('Ctrl Pts',(16.2940809887434,-7.26219165995679,7.));
#12278=CARTESIAN_POINT('Ctrl Pts',(16.2940809887434,-7.26219165995679,-1.39999999999999));
#12279=CARTESIAN_POINT('Ctrl Pts',(16.1361838672874,-7.12742326811383,7.));
#12280=CARTESIAN_POINT('Ctrl Pts',(16.1361838672874,-7.12742326811383,-1.39999999999999));
#12281=CARTESIAN_POINT('Ctrl Pts',(15.9905219781863,-7.01217619187962,7.));
#12282=CARTESIAN_POINT('Ctrl Pts',(15.9905219781863,-7.01217619187962,-1.39999999999999));
#12283=CARTESIAN_POINT('Ctrl Pts',(15.8583036897433,-6.91534043556369,7.));
#12284=CARTESIAN_POINT('Ctrl Pts',(15.8583036897433,-6.91534043556369,-1.39999999999999));
#12285=CARTESIAN_POINT('Ctrl Pts',(15.7406883947777,-6.83570676658069,7.));
#12286=CARTESIAN_POINT('Ctrl Pts',(15.7406883947777,-6.83570676658069,-1.39999999999999));
#12287=CARTESIAN_POINT('Ctrl Pts',(15.6387111659832,-6.77211692048663,7.));
#12288=CARTESIAN_POINT('Ctrl Pts',(15.6387111659832,-6.77211692048663,-1.39999999999999));
#12289=CARTESIAN_POINT('Ctrl Pts',(15.5619248294191,-6.72790031412624,7.));
#12290=CARTESIAN_POINT('Ctrl Pts',(15.5619248294191,-6.72790031412624,-1.39999999999999));
#12291=CARTESIAN_POINT('Ctrl Pts',(15.5083268912119,-6.69953551835472,7.));
#12292=CARTESIAN_POINT('Ctrl Pts',(15.5083268912119,-6.69953551835472,-1.39999999999999));
#12293=CARTESIAN_POINT('Ctrl Pts',(15.4733031879166,-6.68074830397725,7.));
#12294=CARTESIAN_POINT('Ctrl Pts',(15.4733031879166,-6.68074830397725,-1.39999999999999));
#12295=CARTESIAN_POINT('Ctrl Pts',(15.4424051151807,-6.66297054550541,7.));
#12296=CARTESIAN_POINT('Ctrl Pts',(15.4424051151807,-6.66297054550541,-1.39999999999999));
#12297=CARTESIAN_POINT('Ctrl Pts',(15.3933171197393,-6.63306845520276,7.));
#12298=CARTESIAN_POINT('Ctrl Pts',(15.3933171197393,-6.63306845520276,-1.39999999999999));
#12299=CARTESIAN_POINT('Ctrl Pts',(15.3282076647862,-6.58832104206022,7.));
#12300=CARTESIAN_POINT('Ctrl Pts',(15.3282076647862,-6.58832104206022,-1.39999999999999));
#12301=CARTESIAN_POINT('Ctrl Pts',(15.2506809503975,-6.52246995302226,7.));
#12302=CARTESIAN_POINT('Ctrl Pts',(15.2506809503975,-6.52246995302226,-1.39999999999999));
#12303=CARTESIAN_POINT('Ctrl Pts',(15.1795880240196,-6.44397890908496,7.));
#12304=CARTESIAN_POINT('Ctrl Pts',(15.1795880240196,-6.44397890908496,-1.39999999999999));
#12305=CARTESIAN_POINT('Ctrl Pts',(15.1168047097501,-6.34385243988822,7.));
#12306=CARTESIAN_POINT('Ctrl Pts',(15.1168047097501,-6.34385243988822,-1.39999999999999));
#12307=CARTESIAN_POINT('Ctrl Pts',(15.0680440207731,-6.1960413432609,7.));
#12308=CARTESIAN_POINT('Ctrl Pts',(15.0680440207731,-6.1960413432609,-1.39999999999999));
#12309=CARTESIAN_POINT('Ctrl Pts',(15.0769402326058,-6.07637133495394,7.));
#12310=CARTESIAN_POINT('Ctrl Pts',(15.0769402326058,-6.07637133495394,-1.39999999999999));
#12311=CARTESIAN_POINT('Ctrl Pts',(15.0980247376579,-6.00933848448159,7.));
#12312=CARTESIAN_POINT('Ctrl Pts',(15.0980247376579,-6.00933848448159,-1.39999999999999));
#12313=CARTESIAN_POINT('',(15.0980247376579,-6.00933848448159,7.));
#12314=CARTESIAN_POINT('Origin',(0.,0.,7.));
#12315=CARTESIAN_POINT('',(15.7467591314704,-4.01273932064523,7.));
#12316=CARTESIAN_POINT('Ctrl Pts',(15.7467591314704,-4.01273932064524,7.));
#12317=CARTESIAN_POINT('Ctrl Pts',(15.7467591314704,-4.01273932064524,-1.4));
#12318=CARTESIAN_POINT('Ctrl Pts',(15.7691023294921,-3.94611544431022,7.));
#12319=CARTESIAN_POINT('Ctrl Pts',(15.7691023294921,-3.94611544431022,-1.4));
#12320=CARTESIAN_POINT('Ctrl Pts',(15.8322454089585,-3.8440713117564,7.));
#12321=CARTESIAN_POINT('Ctrl Pts',(15.8322454089585,-3.8440713117564,-1.4));
#12322=CARTESIAN_POINT('Ctrl Pts',(15.958574817721,-3.75315043650002,7.));
#12323=CARTESIAN_POINT('Ctrl Pts',(15.958574817721,-3.75315043650002,-1.4));
#12324=CARTESIAN_POINT('Ctrl Pts',(16.0682204478862,-3.70904952755073,7.));
#12325=CARTESIAN_POINT('Ctrl Pts',(16.0682204478862,-3.70904952755073,-1.4));
#12326=CARTESIAN_POINT('Ctrl Pts',(16.1718717115691,-3.68733631276642,7.));
#12327=CARTESIAN_POINT('Ctrl Pts',(16.1718717115691,-3.68733631276642,-1.4));
#12328=CARTESIAN_POINT('Ctrl Pts',(16.2732984400115,-3.67963072201298,7.));
#12329=CARTESIAN_POINT('Ctrl Pts',(16.2732984400115,-3.67963072201298,-1.4));
#12330=CARTESIAN_POINT('Ctrl Pts',(16.3522749650865,-3.68169968173262,7.));
#12331=CARTESIAN_POINT('Ctrl Pts',(16.3522749650865,-3.68169968173262,-1.4));
#12332=CARTESIAN_POINT('Ctrl Pts',(16.409563995311,-3.68636158229546,7.));
#12333=CARTESIAN_POINT('Ctrl Pts',(16.409563995311,-3.68636158229546,-1.4));
#12334=CARTESIAN_POINT('Ctrl Pts',(16.4450105654963,-3.69014050504826,7.));
#12335=CARTESIAN_POINT('Ctrl Pts',(16.4450105654963,-3.69014050504826,-1.4));
#12336=CARTESIAN_POINT('Ctrl Pts',(16.4843881842109,-3.6955277456176,7.));
#12337=CARTESIAN_POINT('Ctrl Pts',(16.4843881842109,-3.6955277456176,-1.4));
#12338=CARTESIAN_POINT('Ctrl Pts',(16.5444222357228,-3.70408422142792,7.));
#12339=CARTESIAN_POINT('Ctrl Pts',(16.5444222357228,-3.70408422142792,-1.4));
#12340=CARTESIAN_POINT('Ctrl Pts',(16.632533556064,-3.71344611165872,7.));
#12341=CARTESIAN_POINT('Ctrl Pts',(16.632533556064,-3.71344611165872,-1.4));
#12342=CARTESIAN_POINT('Ctrl Pts',(16.7524120409277,-3.72194155665406,7.));
#12343=CARTESIAN_POINT('Ctrl Pts',(16.7524120409277,-3.72194155665406,-1.4));
#12344=CARTESIAN_POINT('Ctrl Pts',(16.8943723095674,-3.72664910094713,7.));
#12345=CARTESIAN_POINT('Ctrl Pts',(16.8943723095674,-3.72664910094713,-1.4));
#12346=CARTESIAN_POINT('Ctrl Pts',(17.0582577813421,-3.72602328845455,7.));
#12347=CARTESIAN_POINT('Ctrl Pts',(17.0582577813421,-3.72602328845455,-1.4));
#12348=CARTESIAN_POINT('Ctrl Pts',(17.2438412568379,-3.71840435546376,7.));
#12349=CARTESIAN_POINT('Ctrl Pts',(17.2438412568379,-3.71840435546376,-1.4));
#12350=CARTESIAN_POINT('Ctrl Pts',(17.4507975846592,-3.70218403552949,7.));
#12351=CARTESIAN_POINT('Ctrl Pts',(17.4507975846592,-3.70218403552949,-1.4));
#12352=CARTESIAN_POINT('Ctrl Pts',(17.6787134541915,-3.67575622931335,7.));
#12353=CARTESIAN_POINT('Ctrl Pts',(17.6787134541915,-3.67575622931335,-1.4));
#12354=CARTESIAN_POINT('Ctrl Pts',(17.9270849363835,-3.63753969769582,7.));
#12355=CARTESIAN_POINT('Ctrl Pts',(17.9270849363835,-3.63753969769582,-1.4));
#12356=CARTESIAN_POINT('Ctrl Pts',(18.265123941733,-3.57255446932205,7.));
#12357=CARTESIAN_POINT('Ctrl Pts',(18.265123941733,-3.57255446932205,-1.4));
#12358=CARTESIAN_POINT('Ctrl Pts',(18.5181384456163,-3.51033578853422,7.));
#12359=CARTESIAN_POINT('Ctrl Pts',(18.5181384456163,-3.51033578853422,-1.4));
#12360=CARTESIAN_POINT('Ctrl Pts',(18.6813621637973,-3.46506965370701,7.));
#12361=CARTESIAN_POINT('Ctrl Pts',(18.6813621637973,-3.46506965370701,-1.4));
#12362=CARTESIAN_POINT('',(18.6813621637973,-3.46506965370701,7.));
#12363=CARTESIAN_POINT('Origin',(0.,0.,7.));
#12364=CARTESIAN_POINT('',(18.8377966288376,-2.47738131311191,7.));
#12365=CARTESIAN_POINT('Ctrl Pts',(18.8377966288376,-2.47738131311187,7.));
#12366=CARTESIAN_POINT('Ctrl Pts',(18.8377966288376,-2.47738131311187,-1.39999999999999));
#12367=CARTESIAN_POINT('Ctrl Pts',(18.6965496529788,-2.38389175781396,7.));
#12368=CARTESIAN_POINT('Ctrl Pts',(18.6965496529788,-2.38389175781396,-1.39999999999999));
#12369=CARTESIAN_POINT('Ctrl Pts',(18.4751451900744,-2.24653249449211,7.));
#12370=CARTESIAN_POINT('Ctrl Pts',(18.4751451900744,-2.24653249449211,-1.39999999999999));
#12371=CARTESIAN_POINT('Ctrl Pts',(18.1737325312257,-2.08026807216974,7.));
#12372=CARTESIAN_POINT('Ctrl Pts',(18.1737325312257,-2.08026807216974,-1.39999999999999));
#12373=CARTESIAN_POINT('Ctrl Pts',(17.949326772361,-1.96717098182924,7.));
#12374=CARTESIAN_POINT('Ctrl Pts',(17.949326772361,-1.96717098182924,-1.39999999999999));
#12375=CARTESIAN_POINT('Ctrl Pts',(17.7407325407201,-1.87160676754275,7.));
#12376=CARTESIAN_POINT('Ctrl Pts',(17.7407325407201,-1.87160676754275,-1.39999999999999));
#12377=CARTESIAN_POINT('Ctrl Pts',(17.548917731071,-1.7922273041827,7.));
#12378=CARTESIAN_POINT('Ctrl Pts',(17.548917731071,-1.7922273041827,-1.39999999999999));
#12379=CARTESIAN_POINT('Ctrl Pts',(17.3747717371572,-1.72763282051117,7.));
#12380=CARTESIAN_POINT('Ctrl Pts',(17.3747717371572,-1.72763282051117,-1.39999999999999));
#12381=CARTESIAN_POINT('Ctrl Pts',(17.2191007779952,-1.67639424155261,7.));
#12382=CARTESIAN_POINT('Ctrl Pts',(17.2191007779952,-1.67639424155261,-1.39999999999999));
#12383=CARTESIAN_POINT('Ctrl Pts',(17.0826338282621,-1.6370032466926,7.));
#12384=CARTESIAN_POINT('Ctrl Pts',(17.0826338282621,-1.6370032466926,-1.39999999999999));
#12385=CARTESIAN_POINT('Ctrl Pts',(16.9659973771906,-1.60803840593143,7.));
#12386=CARTESIAN_POINT('Ctrl Pts',(16.9659973771906,-1.60803840593143,-1.39999999999999));
#12387=CARTESIAN_POINT('Ctrl Pts',(16.8793055486399,-1.58971419725802,7.));
#12388=CARTESIAN_POINT('Ctrl Pts',(16.8793055486399,-1.58971419725802,-1.39999999999999));
#12389=CARTESIAN_POINT('Ctrl Pts',(16.8195656763126,-1.57930034717563,7.));
#12390=CARTESIAN_POINT('Ctrl Pts',(16.8195656763126,-1.57930034717563,-1.39999999999999));
#12391=CARTESIAN_POINT('Ctrl Pts',(16.7804505865492,-1.57225556404309,7.));
#12392=CARTESIAN_POINT('Ctrl Pts',(16.7804505865492,-1.57225556404309,-1.39999999999999));
#12393=CARTESIAN_POINT('Ctrl Pts',(16.7455711436431,-1.56489594057215,7.));
#12394=CARTESIAN_POINT('Ctrl Pts',(16.7455711436431,-1.56489594057215,-1.39999999999999));
#12395=CARTESIAN_POINT('Ctrl Pts',(16.6896454316358,-1.55162638755015,7.));
#12396=CARTESIAN_POINT('Ctrl Pts',(16.6896454316358,-1.55162638755015,-1.39999999999999));
#12397=CARTESIAN_POINT('Ctrl Pts',(16.6138949491149,-1.5291889967686,7.));
#12398=CARTESIAN_POINT('Ctrl Pts',(16.6138949491149,-1.5291889967686,-1.39999999999999));
#12399=CARTESIAN_POINT('Ctrl Pts',(16.5198135565977,-1.49051796169807,7.));
#12400=CARTESIAN_POINT('Ctrl Pts',(16.5198135565977,-1.49051796169807,-1.39999999999999));
#12401=CARTESIAN_POINT('Ctrl Pts',(16.4279450992207,-1.43783746532129,7.));
#12402=CARTESIAN_POINT('Ctrl Pts',(16.4279450992207,-1.43783746532129,-1.39999999999999));
#12403=CARTESIAN_POINT('Ctrl Pts',(16.3372938385016,-1.36201264541057,7.));
#12404=CARTESIAN_POINT('Ctrl Pts',(16.3372938385016,-1.36201264541057,-1.39999999999999));
#12405=CARTESIAN_POINT('Ctrl Pts',(16.2452435266959,-1.23650382033374,7.));
#12406=CARTESIAN_POINT('Ctrl Pts',(16.2452435266959,-1.23650382033374,-1.39999999999999));
#12407=CARTESIAN_POINT('Ctrl Pts',(16.2167242606458,-1.11994179848647,7.));
#12408=CARTESIAN_POINT('Ctrl Pts',(16.2167242606458,-1.11994179848647,-1.39999999999999));
#12409=CARTESIAN_POINT('Ctrl Pts',(16.2160625265911,-1.04967429885982,7.));
#12410=CARTESIAN_POINT('Ctrl Pts',(16.2160625265911,-1.04967429885982,-1.39999999999999));
#12411=CARTESIAN_POINT('',(16.2160625265911,-1.04967429885982,7.));
#12412=CARTESIAN_POINT('Origin',(0.,0.,7.));
#12413=CARTESIAN_POINT('',(16.2160625265911,1.0496742988598,7.));
#12414=CARTESIAN_POINT('Ctrl Pts',(16.2160625265911,1.04967429885982,7.));
#12415=CARTESIAN_POINT('Ctrl Pts',(16.2160625265911,1.04967429885982,-1.4));
#12416=CARTESIAN_POINT('Ctrl Pts',(16.2167242606459,1.11994179848647,7.));
#12417=CARTESIAN_POINT('Ctrl Pts',(16.2167242606459,1.11994179848647,-1.4));
#12418=CARTESIAN_POINT('Ctrl Pts',(16.2452435266959,1.23650382033374,7.));
#12419=CARTESIAN_POINT('Ctrl Pts',(16.2452435266959,1.23650382033374,-1.4));
#12420=CARTESIAN_POINT('Ctrl Pts',(16.3372938385016,1.36201264541054,7.));
#12421=CARTESIAN_POINT('Ctrl Pts',(16.3372938385016,1.36201264541054,-1.4));
#12422=CARTESIAN_POINT('Ctrl Pts',(16.4279450992208,1.43783746532129,7.));
#12423=CARTESIAN_POINT('Ctrl Pts',(16.4279450992208,1.43783746532129,-1.4));
#12424=CARTESIAN_POINT('Ctrl Pts',(16.5198135565978,1.49051796169809,7.));
#12425=CARTESIAN_POINT('Ctrl Pts',(16.5198135565978,1.49051796169809,-1.4));
#12426=CARTESIAN_POINT('Ctrl Pts',(16.6138949491149,1.52918899676861,7.));
#12427=CARTESIAN_POINT('Ctrl Pts',(16.6138949491149,1.52918899676861,-1.4));
#12428=CARTESIAN_POINT('Ctrl Pts',(16.6896454316359,1.55162638755015,7.));
#12429=CARTESIAN_POINT('Ctrl Pts',(16.6896454316359,1.55162638755015,-1.4));
#12430=CARTESIAN_POINT('Ctrl Pts',(16.7455711436431,1.56489594057217,7.));
#12431=CARTESIAN_POINT('Ctrl Pts',(16.7455711436431,1.56489594057217,-1.4));
#12432=CARTESIAN_POINT('Ctrl Pts',(16.7804505865492,1.57225556404311,7.));
#12433=CARTESIAN_POINT('Ctrl Pts',(16.7804505865492,1.57225556404311,-1.4));
#12434=CARTESIAN_POINT('Ctrl Pts',(16.8195656763126,1.57930034717561,7.));
#12435=CARTESIAN_POINT('Ctrl Pts',(16.8195656763126,1.57930034717561,-1.4));
#12436=CARTESIAN_POINT('Ctrl Pts',(16.8793055486399,1.58971419725803,7.));
#12437=CARTESIAN_POINT('Ctrl Pts',(16.8793055486399,1.58971419725803,-1.4));
#12438=CARTESIAN_POINT('Ctrl Pts',(16.9659973771906,1.60803840593143,7.));
#12439=CARTESIAN_POINT('Ctrl Pts',(16.9659973771906,1.60803840593143,-1.4));
#12440=CARTESIAN_POINT('Ctrl Pts',(17.0826338282621,1.63700324669259,7.));
#12441=CARTESIAN_POINT('Ctrl Pts',(17.0826338282621,1.63700324669259,-1.4));
#12442=CARTESIAN_POINT('Ctrl Pts',(17.2191007779953,1.67639424155262,7.));
#12443=CARTESIAN_POINT('Ctrl Pts',(17.2191007779953,1.67639424155262,-1.4));
#12444=CARTESIAN_POINT('Ctrl Pts',(17.3747717371572,1.7276328205112,7.));
#12445=CARTESIAN_POINT('Ctrl Pts',(17.3747717371572,1.7276328205112,-1.4));
#12446=CARTESIAN_POINT('Ctrl Pts',(17.548917731071,1.79222730418268,7.));
#12447=CARTESIAN_POINT('Ctrl Pts',(17.548917731071,1.79222730418268,-1.4));
#12448=CARTESIAN_POINT('Ctrl Pts',(17.7407325407201,1.87160676754277,7.));
#12449=CARTESIAN_POINT('Ctrl Pts',(17.7407325407201,1.87160676754277,-1.4));
#12450=CARTESIAN_POINT('Ctrl Pts',(17.949326772361,1.96717098182924,7.));
#12451=CARTESIAN_POINT('Ctrl Pts',(17.949326772361,1.96717098182924,-1.4));
#12452=CARTESIAN_POINT('Ctrl Pts',(18.1737325312257,2.08026807216972,7.));
#12453=CARTESIAN_POINT('Ctrl Pts',(18.1737325312257,2.08026807216972,-1.4));
#12454=CARTESIAN_POINT('Ctrl Pts',(18.4751451900744,2.2465324944921,7.));
#12455=CARTESIAN_POINT('Ctrl Pts',(18.4751451900744,2.2465324944921,-1.4));
#12456=CARTESIAN_POINT('Ctrl Pts',(18.6965496529788,2.38389175781394,7.));
#12457=CARTESIAN_POINT('Ctrl Pts',(18.6965496529788,2.38389175781394,-1.4));
#12458=CARTESIAN_POINT('Ctrl Pts',(18.8377966288376,2.47738131311188,7.));
#12459=CARTESIAN_POINT('Ctrl Pts',(18.8377966288376,2.47738131311188,-1.4));
#12460=CARTESIAN_POINT('',(18.8377966288376,2.47738131311188,7.));
#12461=CARTESIAN_POINT('Origin',(1.73472347597681E-15,0.,7.));
#12462=CARTESIAN_POINT('',(18.6813621637973,3.46506965370699,7.));
#12463=CARTESIAN_POINT('Ctrl Pts',(18.6813621637973,3.46506965370701,7.));
#12464=CARTESIAN_POINT('Ctrl Pts',(18.6813621637973,3.46506965370701,-1.39999999999999));
#12465=CARTESIAN_POINT('Ctrl Pts',(18.5181384456162,3.51033578853419,7.));
#12466=CARTESIAN_POINT('Ctrl Pts',(18.5181384456162,3.51033578853419,-1.39999999999999));
#12467=CARTESIAN_POINT('Ctrl Pts',(18.2651239417329,3.57255446932204,7.));
#12468=CARTESIAN_POINT('Ctrl Pts',(18.2651239417329,3.57255446932204,-1.39999999999999));
#12469=CARTESIAN_POINT('Ctrl Pts',(17.9270849363835,3.63753969769579,7.));
#12470=CARTESIAN_POINT('Ctrl Pts',(17.9270849363835,3.63753969769579,-1.39999999999999));
#12471=CARTESIAN_POINT('Ctrl Pts',(17.6787134541915,3.67575622931334,7.));
#12472=CARTESIAN_POINT('Ctrl Pts',(17.6787134541915,3.67575622931334,-1.39999999999999));
#12473=CARTESIAN_POINT('Ctrl Pts',(17.4507975846592,3.70218403552951,7.));
#12474=CARTESIAN_POINT('Ctrl Pts',(17.4507975846592,3.70218403552951,-1.39999999999999));
#12475=CARTESIAN_POINT('Ctrl Pts',(17.2438412568379,3.71840435546372,7.));
#12476=CARTESIAN_POINT('Ctrl Pts',(17.2438412568379,3.71840435546372,-1.39999999999999));
#12477=CARTESIAN_POINT('Ctrl Pts',(17.0582577813421,3.72602328845457,7.));
#12478=CARTESIAN_POINT('Ctrl Pts',(17.0582577813421,3.72602328845457,-1.39999999999999));
#12479=CARTESIAN_POINT('Ctrl Pts',(16.8943723095674,3.72664910094712,7.));
#12480=CARTESIAN_POINT('Ctrl Pts',(16.8943723095674,3.72664910094712,-1.39999999999999));
#12481=CARTESIAN_POINT('Ctrl Pts',(16.7524120409277,3.72194155665404,7.));
#12482=CARTESIAN_POINT('Ctrl Pts',(16.7524120409277,3.72194155665404,-1.39999999999999));
#12483=CARTESIAN_POINT('Ctrl Pts',(16.632533556064,3.71344611165872,7.));
#12484=CARTESIAN_POINT('Ctrl Pts',(16.632533556064,3.71344611165872,-1.39999999999999));
#12485=CARTESIAN_POINT('Ctrl Pts',(16.5444222357228,3.70408422142792,7.));
#12486=CARTESIAN_POINT('Ctrl Pts',(16.5444222357228,3.70408422142792,-1.39999999999999));
#12487=CARTESIAN_POINT('Ctrl Pts',(16.4843881842109,3.69552774561757,7.));
#12488=CARTESIAN_POINT('Ctrl Pts',(16.4843881842109,3.69552774561757,-1.39999999999999));
#12489=CARTESIAN_POINT('Ctrl Pts',(16.4450105654963,3.69014050504827,7.));
#12490=CARTESIAN_POINT('Ctrl Pts',(16.4450105654963,3.69014050504827,-1.39999999999999));
#12491=CARTESIAN_POINT('Ctrl Pts',(16.409563995311,3.68636158229547,7.));
#12492=CARTESIAN_POINT('Ctrl Pts',(16.409563995311,3.68636158229547,-1.39999999999999));
#12493=CARTESIAN_POINT('Ctrl Pts',(16.3522749650865,3.68169968173261,7.));
#12494=CARTESIAN_POINT('Ctrl Pts',(16.3522749650865,3.68169968173261,-1.39999999999999));
#12495=CARTESIAN_POINT('Ctrl Pts',(16.2732984400115,3.67963072201297,7.));
#12496=CARTESIAN_POINT('Ctrl Pts',(16.2732984400115,3.67963072201297,-1.39999999999999));
#12497=CARTESIAN_POINT('Ctrl Pts',(16.1718717115691,3.68733631276642,7.));
#12498=CARTESIAN_POINT('Ctrl Pts',(16.1718717115691,3.68733631276642,-1.39999999999999));
#12499=CARTESIAN_POINT('Ctrl Pts',(16.0682204478862,3.70904952755071,7.));
#12500=CARTESIAN_POINT('Ctrl Pts',(16.0682204478862,3.70904952755071,-1.39999999999999));
#12501=CARTESIAN_POINT('Ctrl Pts',(15.958574817721,3.75315043649999,7.));
#12502=CARTESIAN_POINT('Ctrl Pts',(15.958574817721,3.75315043649999,-1.39999999999999));
#12503=CARTESIAN_POINT('Ctrl Pts',(15.8322454089585,3.84407131175639,7.));
#12504=CARTESIAN_POINT('Ctrl Pts',(15.8322454089585,3.84407131175639,-1.39999999999999));
#12505=CARTESIAN_POINT('Ctrl Pts',(15.7691023294921,3.94611544431022,7.));
#12506=CARTESIAN_POINT('Ctrl Pts',(15.7691023294921,3.94611544431022,-1.39999999999999));
#12507=CARTESIAN_POINT('Ctrl Pts',(15.7467591314704,4.01273932064524,7.));
#12508=CARTESIAN_POINT('Ctrl Pts',(15.7467591314704,4.01273932064524,-1.39999999999999));
#12509=CARTESIAN_POINT('',(15.7467591314704,4.01273932064524,7.));
#12510=CARTESIAN_POINT('Origin',(0.,0.,7.));
#12511=CARTESIAN_POINT('Origin',(0.,0.,6.));
#12512=CARTESIAN_POINT('Origin',(0.,0.,1.));
#12950=UNCERTAINTY_MEASURE_WITH_UNIT(LENGTH_MEASURE(0.01),#12967,
'DISTANCE_ACCURACY_VALUE',
'Maximum model space distance between geometric entities at asserted c
onnectivities');
#12956=UNCERTAINTY_MEASURE_WITH_UNIT(LENGTH_MEASURE(0.01),#12967,
'DISTANCE_ACCURACY_VALUE',
'Maximum model space distance between geometric entities at asserted c
onnectivities');
#12960=(
GEOMETRIC_REPRESENTATION_CONTEXT(3)
GLOBAL_UNCERTAINTY_ASSIGNED_CONTEXT((#12950))
GLOBAL_UNIT_ASSIGNED_CONTEXT((#12967,#12969,#12970))
REPRESENTATION_CONTEXT('','3D')
);
#12966=(
GEOMETRIC_REPRESENTATION_CONTEXT(3)
GLOBAL_UNCERTAINTY_ASSIGNED_CONTEXT((#12956))
GLOBAL_UNIT_ASSIGNED_CONTEXT((#12967,#12969,#12970))
REPRESENTATION_CONTEXT('','3D')
);
#12967=(
LENGTH_UNIT()
NAMED_UNIT(*)
SI_UNIT(.MILLI.,.METRE.)
);
#12969=(
NAMED_UNIT(*)
PLANE_ANGLE_UNIT()
SI_UNIT($,.RADIAN.)
);
#12970=(
NAMED_UNIT(*)
SI_UNIT($,.STERADIAN.)
SOLID_ANGLE_UNIT()
);
#12974=SHAPE_DEFINITION_REPRESENTATION(#12983,#13027);
#12983=PRODUCT_DEFINITION_SHAPE('',$,#13037);
#13027=SHAPE_REPRESENTATION('',(#5884),#12960);
#13033=PRODUCT_DEFINITION_CONTEXT('part definition',#13062,'design');
#13037=PRODUCT_DEFINITION('Gear','Gear',#13046,#13033);
#13046=PRODUCT_DEFINITION_FORMATION('',$,#13067);
#13062=APPLICATION_CONTEXT(
'Core Data for Automotive Mechanical Design Process');
#13063=PRODUCT_CONTEXT('part definition',#13062,'mechanical');
#13067=PRODUCT('Gear','Gear',$,(#13063));
#13076=PRESENTATION_STYLE_ASSIGNMENT((#13081));
#13081=SURFACE_STYLE_USAGE(.BOTH.,#13086);
#13086=SURFACE_SIDE_STYLE('',(#13091));
#13091=SURFACE_STYLE_FILL_AREA(#13096);
#13096=FILL_AREA_STYLE('Opaque(227,224,212)',(#13101));
#13101=FILL_AREA_STYLE_COLOUR('Opaque(227,224,212)',#13106);
#13106=COLOUR_RGB('Opaque(227,224,212)',0.890196078431372,0.87843137254902,
0.831372549019608);
ENDSEC;
END-ISO-10303-21;
